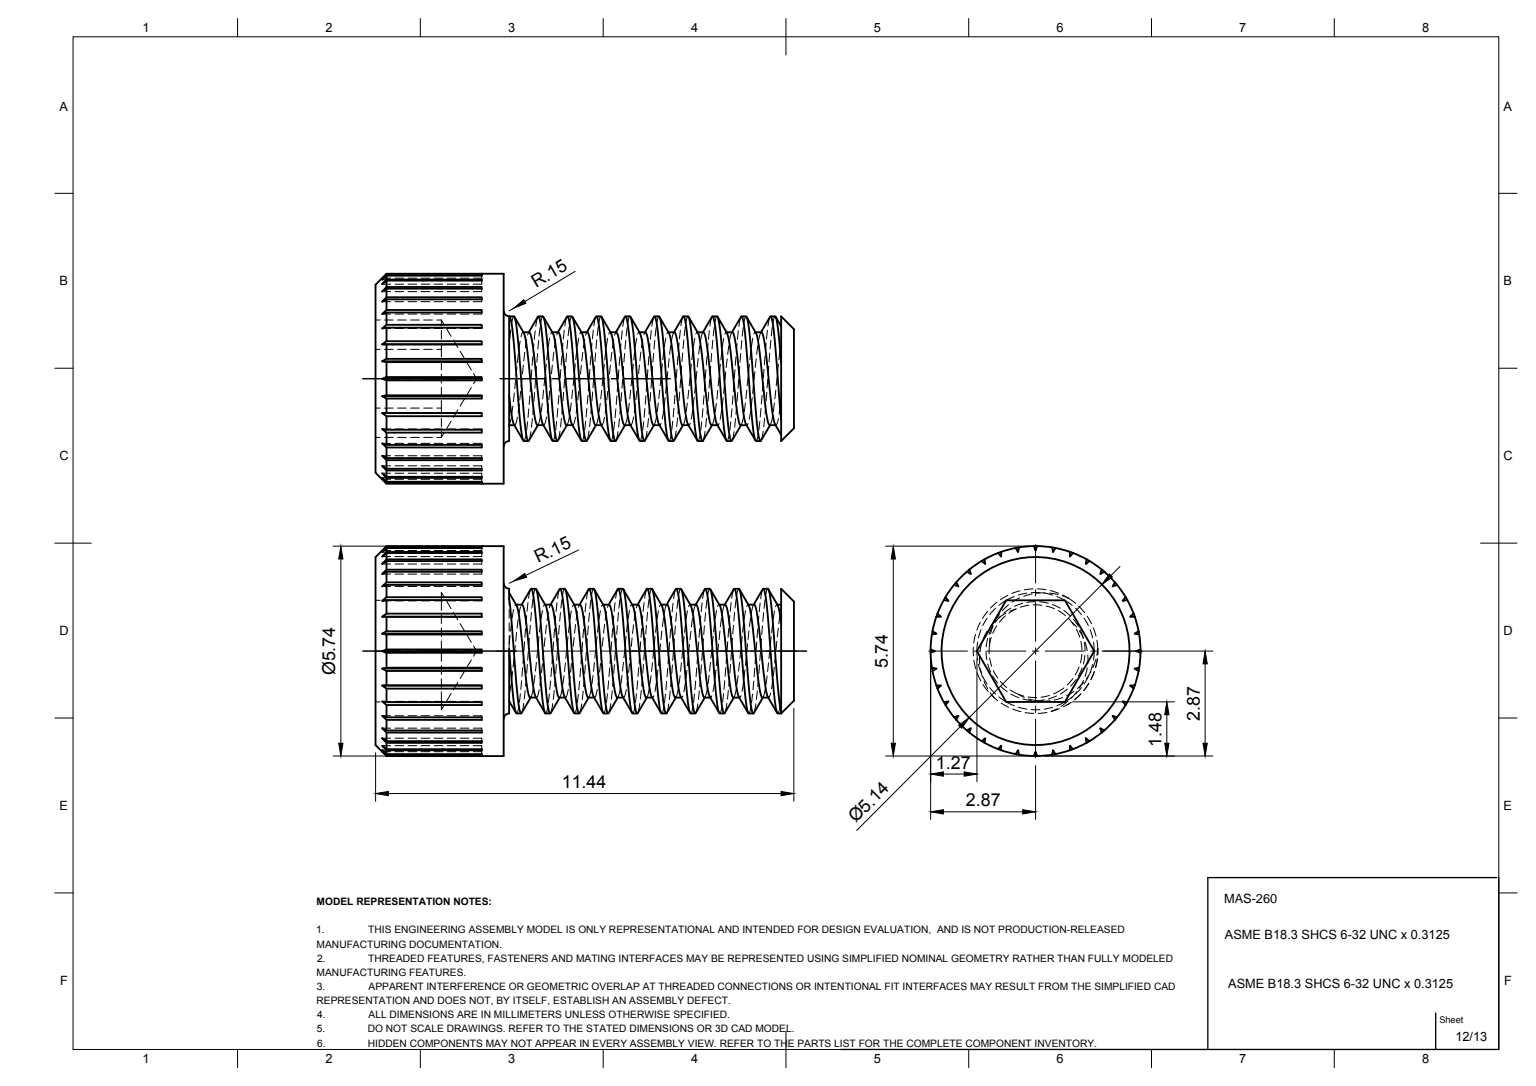
ISO-10303-21;
HEADER;
/* Generated by software containing ST-Developer
 * from STEP Tools, Inc. (www.steptools.com) 
 */

FILE_DESCRIPTION(
/* description */ (''),
/* implementation_level */ '2;1');

FILE_NAME(
/* name */ 'ASME B18.3 SHCS 6-32 UNC x 0.3125.step',
/* time_stamp */ '2026-10-15T13:29:10-07:00',
/* author */ (''),
/* organization */ (''),
/* preprocessor_version */ 'ST-DEVELOPER v20.2',
/* originating_system */ 'Autodesk Translation Framework v15.15.0.0',
/* authorisation */ '');

FILE_SCHEMA (('AUTOMOTIVE_DESIGN { 1 0 10303 214 3 1 1 }'));
ENDSEC;

DATA;
#10=MECHANICAL_DESIGN_GEOMETRIC_PRESENTATION_REPRESENTATION('',(#943),#83219);
#353=(
BOUNDED_CURVE()
B_SPLINE_CURVE(2,(#65992,#65993,#65994),.UNSPECIFIED.,.F.,.F.)
B_SPLINE_CURVE_WITH_KNOTS((3,3),(0.,0.0169283274323722),.UNSPECIFIED.)
CURVE()
GEOMETRIC_REPRESENTATION_ITEM()
RATIONAL_B_SPLINE_CURVE((1.,1.00067437545138,1.00082963690455))
REPRESENTATION_ITEM('')
);
#354=(
BOUNDED_CURVE()
B_SPLINE_CURVE(2,(#65999,#66000,#66001),.UNSPECIFIED.,.F.,.F.)
B_SPLINE_CURVE_WITH_KNOTS((3,3),(0.0270544913418023,0.0439828187741892),
 .UNSPECIFIED.)
CURVE()
GEOMETRIC_REPRESENTATION_ITEM()
RATIONAL_B_SPLINE_CURVE((1.00082963690332,1.00067437545039,1.))
REPRESENTATION_ITEM('')
);
#355=(
BOUNDED_CURVE()
B_SPLINE_CURVE(2,(#66008,#66009,#66010),.UNSPECIFIED.,.F.,.F.)
B_SPLINE_CURVE_WITH_KNOTS((3,3),(0.0270544913418047,0.0439828187741891),
 .UNSPECIFIED.)
CURVE()
GEOMETRIC_REPRESENTATION_ITEM()
RATIONAL_B_SPLINE_CURVE((1.00082963690338,1.00067437545043,1.))
REPRESENTATION_ITEM('')
);
#356=(
BOUNDED_CURVE()
B_SPLINE_CURVE(2,(#66014,#66015,#66016),.UNSPECIFIED.,.F.,.F.)
B_SPLINE_CURVE_WITH_KNOTS((3,3),(0.,0.0169283274323899),.UNSPECIFIED.)
CURVE()
GEOMETRIC_REPRESENTATION_ITEM()
RATIONAL_B_SPLINE_CURVE((1.,1.00067437544971,1.00082963690249))
REPRESENTATION_ITEM('')
);
#357=(
BOUNDED_CURVE()
B_SPLINE_CURVE(2,(#66018,#66019,#66020),.UNSPECIFIED.,.F.,.F.)
B_SPLINE_CURVE_WITH_KNOTS((3,3),(0.0270544913417485,0.0439828187741892),
 .UNSPECIFIED.)
CURVE()
GEOMETRIC_REPRESENTATION_ITEM()
RATIONAL_B_SPLINE_CURVE((1.00082963689667,1.00067437544498,1.))
REPRESENTATION_ITEM('')
);
#358=(
BOUNDED_CURVE()
B_SPLINE_CURVE(2,(#66024,#66025,#66026),.UNSPECIFIED.,.F.,.F.)
B_SPLINE_CURVE_WITH_KNOTS((3,3),(0.,0.0169283274324321),.UNSPECIFIED.)
CURVE()
GEOMETRIC_REPRESENTATION_ITEM()
RATIONAL_B_SPLINE_CURVE((1.,1.00067437544514,1.00082963689687))
REPRESENTATION_ITEM('')
);
#359=(
BOUNDED_CURVE()
B_SPLINE_CURVE(2,(#66028,#66029,#66030),.UNSPECIFIED.,.F.,.F.)
B_SPLINE_CURVE_WITH_KNOTS((3,3),(0.0270544913417875,0.0439828187741892),
 .UNSPECIFIED.)
CURVE()
GEOMETRIC_REPRESENTATION_ITEM()
RATIONAL_B_SPLINE_CURVE((1.00082963689786,1.00067437544595,1.))
REPRESENTATION_ITEM('')
);
#360=(
BOUNDED_CURVE()
B_SPLINE_CURVE(2,(#66034,#66035,#66036),.UNSPECIFIED.,.F.,.F.)
B_SPLINE_CURVE_WITH_KNOTS((3,3),(0.,0.0169283274323828),.UNSPECIFIED.)
CURVE()
GEOMETRIC_REPRESENTATION_ITEM()
RATIONAL_B_SPLINE_CURVE((1.,1.00067437545006,1.00082963690291))
REPRESENTATION_ITEM('')
);
#361=(
BOUNDED_CURVE()
B_SPLINE_CURVE(2,(#66038,#66039,#66040),.UNSPECIFIED.,.F.,.F.)
B_SPLINE_CURVE_WITH_KNOTS((3,3),(0.0270544913418211,0.0439828187741892),
 .UNSPECIFIED.)
CURVE()
GEOMETRIC_REPRESENTATION_ITEM()
RATIONAL_B_SPLINE_CURVE((1.00082963690425,1.00067437545114,1.))
REPRESENTATION_ITEM('')
);
#362=(
BOUNDED_CURVE()
B_SPLINE_CURVE(2,(#66044,#66045,#66046),.UNSPECIFIED.,.F.,.F.)
B_SPLINE_CURVE_WITH_KNOTS((3,3),(0.,0.0169283274323665),.UNSPECIFIED.)
CURVE()
GEOMETRIC_REPRESENTATION_ITEM()
RATIONAL_B_SPLINE_CURVE((1.,1.00067437544743,1.00082963689969))
REPRESENTATION_ITEM('')
);
#363=(
BOUNDED_CURVE()
B_SPLINE_CURVE(2,(#66048,#66049,#66050),.UNSPECIFIED.,.F.,.F.)
B_SPLINE_CURVE_WITH_KNOTS((3,3),(0.0270544913417642,0.043982818774189),
 .UNSPECIFIED.)
CURVE()
GEOMETRIC_REPRESENTATION_ITEM()
RATIONAL_B_SPLINE_CURVE((1.00082963689682,1.0006743754451,1.))
REPRESENTATION_ITEM('')
);
#364=(
BOUNDED_CURVE()
B_SPLINE_CURVE(2,(#66054,#66055,#66056),.UNSPECIFIED.,.F.,.F.)
B_SPLINE_CURVE_WITH_KNOTS((3,3),(0.,0.0169283274324012),.UNSPECIFIED.)
CURVE()
GEOMETRIC_REPRESENTATION_ITEM()
RATIONAL_B_SPLINE_CURVE((1.,1.00067437544784,1.00082963690019))
REPRESENTATION_ITEM('')
);
#365=(
BOUNDED_CURVE()
B_SPLINE_CURVE(2,(#66058,#66059,#66060),.UNSPECIFIED.,.F.,.F.)
B_SPLINE_CURVE_WITH_KNOTS((3,3),(0.0270544913418049,0.0439828187741891),
 .UNSPECIFIED.)
CURVE()
GEOMETRIC_REPRESENTATION_ITEM()
RATIONAL_B_SPLINE_CURVE((1.00082963689975,1.00067437544748,1.))
REPRESENTATION_ITEM('')
);
#366=(
BOUNDED_CURVE()
B_SPLINE_CURVE(2,(#66064,#66065,#66066),.UNSPECIFIED.,.F.,.F.)
B_SPLINE_CURVE_WITH_KNOTS((3,3),(0.,0.0169283274323776),.UNSPECIFIED.)
CURVE()
GEOMETRIC_REPRESENTATION_ITEM()
RATIONAL_B_SPLINE_CURVE((1.,1.00067437545055,1.00082963690352))
REPRESENTATION_ITEM('')
);
#367=(
BOUNDED_CURVE()
B_SPLINE_CURVE(2,(#66068,#66069,#66070),.UNSPECIFIED.,.F.,.F.)
B_SPLINE_CURVE_WITH_KNOTS((3,3),(0.0270544913417675,0.0439828187741888),
 .UNSPECIFIED.)
CURVE()
GEOMETRIC_REPRESENTATION_ITEM()
RATIONAL_B_SPLINE_CURVE((1.00082963689636,1.00067437544473,1.))
REPRESENTATION_ITEM('')
);
#368=(
BOUNDED_CURVE()
B_SPLINE_CURVE(2,(#66074,#66075,#66076),.UNSPECIFIED.,.F.,.F.)
B_SPLINE_CURVE_WITH_KNOTS((3,3),(0.,0.0169283274323805),.UNSPECIFIED.)
CURVE()
GEOMETRIC_REPRESENTATION_ITEM()
RATIONAL_B_SPLINE_CURVE((1.,1.00067437545024,1.00082963690314))
REPRESENTATION_ITEM('')
);
#369=(
BOUNDED_CURVE()
B_SPLINE_CURVE(2,(#66078,#66079,#66080),.UNSPECIFIED.,.F.,.F.)
B_SPLINE_CURVE_WITH_KNOTS((3,3),(0.0270544913417762,0.0439828187741891),
 .UNSPECIFIED.)
CURVE()
GEOMETRIC_REPRESENTATION_ITEM()
RATIONAL_B_SPLINE_CURVE((1.00082963689788,1.00067437544596,1.))
REPRESENTATION_ITEM('')
);
#370=(
BOUNDED_CURVE()
B_SPLINE_CURVE(2,(#66084,#66085,#66086),.UNSPECIFIED.,.F.,.F.)
B_SPLINE_CURVE_WITH_KNOTS((3,3),(0.,0.0169283274323929),.UNSPECIFIED.)
CURVE()
GEOMETRIC_REPRESENTATION_ITEM()
RATIONAL_B_SPLINE_CURVE((1.,1.00067437545034,1.00082963690327))
REPRESENTATION_ITEM('')
);
#371=(
BOUNDED_CURVE()
B_SPLINE_CURVE(2,(#66088,#66089,#66090),.UNSPECIFIED.,.F.,.F.)
B_SPLINE_CURVE_WITH_KNOTS((3,3),(0.0270544913417606,0.0439828187741894),
 .UNSPECIFIED.)
CURVE()
GEOMETRIC_REPRESENTATION_ITEM()
RATIONAL_B_SPLINE_CURVE((1.00082963689914,1.00067437544699,1.))
REPRESENTATION_ITEM('')
);
#372=(
BOUNDED_CURVE()
B_SPLINE_CURVE(2,(#66094,#66095,#66096),.UNSPECIFIED.,.F.,.F.)
B_SPLINE_CURVE_WITH_KNOTS((3,3),(0.,0.0169283274323603),.UNSPECIFIED.)
CURVE()
GEOMETRIC_REPRESENTATION_ITEM()
RATIONAL_B_SPLINE_CURVE((1.,1.00067437544665,1.00082963689872))
REPRESENTATION_ITEM('')
);
#373=(
BOUNDED_CURVE()
B_SPLINE_CURVE(2,(#66098,#66099,#66100),.UNSPECIFIED.,.F.,.F.)
B_SPLINE_CURVE_WITH_KNOTS((3,3),(0.0270544913417842,0.043982818774189),
 .UNSPECIFIED.)
CURVE()
GEOMETRIC_REPRESENTATION_ITEM()
RATIONAL_B_SPLINE_CURVE((1.00082963689636,1.00067437544473,1.))
REPRESENTATION_ITEM('')
);
#374=(
BOUNDED_CURVE()
B_SPLINE_CURVE(2,(#66104,#66105,#66106),.UNSPECIFIED.,.F.,.F.)
B_SPLINE_CURVE_WITH_KNOTS((3,3),(0.,0.0169283274323958),.UNSPECIFIED.)
CURVE()
GEOMETRIC_REPRESENTATION_ITEM()
RATIONAL_B_SPLINE_CURVE((1.,1.00067437544716,1.00082963689935))
REPRESENTATION_ITEM('')
);
#375=(
BOUNDED_CURVE()
B_SPLINE_CURVE(2,(#66108,#66109,#66110),.UNSPECIFIED.,.F.,.F.)
B_SPLINE_CURVE_WITH_KNOTS((3,3),(0.0270544913417961,0.0439828187741891),
 .UNSPECIFIED.)
CURVE()
GEOMETRIC_REPRESENTATION_ITEM()
RATIONAL_B_SPLINE_CURVE((1.00082963689727,1.00067437544546,1.))
REPRESENTATION_ITEM('')
);
#376=(
BOUNDED_CURVE()
B_SPLINE_CURVE(2,(#66114,#66115,#66116),.UNSPECIFIED.,.F.,.F.)
B_SPLINE_CURVE_WITH_KNOTS((3,3),(0.,0.016928327432345),.UNSPECIFIED.)
CURVE()
GEOMETRIC_REPRESENTATION_ITEM()
RATIONAL_B_SPLINE_CURVE((1.,1.00067437545236,1.00082963690575))
REPRESENTATION_ITEM('')
);
#377=(
BOUNDED_CURVE()
B_SPLINE_CURVE(2,(#66118,#66119,#66120),.UNSPECIFIED.,.F.,.F.)
B_SPLINE_CURVE_WITH_KNOTS((3,3),(0.0270544913417455,0.0439828187741891),
 .UNSPECIFIED.)
CURVE()
GEOMETRIC_REPRESENTATION_ITEM()
RATIONAL_B_SPLINE_CURVE((1.00082963689847,1.00067437544644,1.))
REPRESENTATION_ITEM('')
);
#378=(
BOUNDED_CURVE()
B_SPLINE_CURVE(2,(#66124,#66125,#66126),.UNSPECIFIED.,.F.,.F.)
B_SPLINE_CURVE_WITH_KNOTS((3,3),(0.,0.0169283274324359),.UNSPECIFIED.)
CURVE()
GEOMETRIC_REPRESENTATION_ITEM()
RATIONAL_B_SPLINE_CURVE((1.,1.00067437544276,1.00082963689394))
REPRESENTATION_ITEM('')
);
#379=(
BOUNDED_CURVE()
B_SPLINE_CURVE(2,(#66128,#66129,#66130),.UNSPECIFIED.,.F.,.F.)
B_SPLINE_CURVE_WITH_KNOTS((3,3),(0.0270544913417467,0.0439828187741893),
 .UNSPECIFIED.)
CURVE()
GEOMETRIC_REPRESENTATION_ITEM()
RATIONAL_B_SPLINE_CURVE((1.00082963690043,1.00067437544804,1.))
REPRESENTATION_ITEM('')
);
#380=(
BOUNDED_CURVE()
B_SPLINE_CURVE(2,(#66134,#66135,#66136),.UNSPECIFIED.,.F.,.F.)
B_SPLINE_CURVE_WITH_KNOTS((3,3),(0.,0.0169283274323855),.UNSPECIFIED.)
CURVE()
GEOMETRIC_REPRESENTATION_ITEM()
RATIONAL_B_SPLINE_CURVE((1.,1.00067437545031,1.00082963690323))
REPRESENTATION_ITEM('')
);
#381=(
BOUNDED_CURVE()
B_SPLINE_CURVE(2,(#66138,#66139,#66140),.UNSPECIFIED.,.F.,.F.)
B_SPLINE_CURVE_WITH_KNOTS((3,3),(0.0270544913418194,0.043982818774189),
 .UNSPECIFIED.)
CURVE()
GEOMETRIC_REPRESENTATION_ITEM()
RATIONAL_B_SPLINE_CURVE((1.0008296369013,1.00067437544875,1.))
REPRESENTATION_ITEM('')
);
#382=(
BOUNDED_CURVE()
B_SPLINE_CURVE(2,(#66144,#66145,#66146),.UNSPECIFIED.,.F.,.F.)
B_SPLINE_CURVE_WITH_KNOTS((3,3),(0.,0.0169283274324108),.UNSPECIFIED.)
CURVE()
GEOMETRIC_REPRESENTATION_ITEM()
RATIONAL_B_SPLINE_CURVE((1.,1.00067437544706,1.00082963689923))
REPRESENTATION_ITEM('')
);
#383=(
BOUNDED_CURVE()
B_SPLINE_CURVE(2,(#66148,#66149,#66150),.UNSPECIFIED.,.F.,.F.)
B_SPLINE_CURVE_WITH_KNOTS((3,3),(0.0270544913418122,0.043982818774189),
 .UNSPECIFIED.)
CURVE()
GEOMETRIC_REPRESENTATION_ITEM()
RATIONAL_B_SPLINE_CURVE((1.00082963689602,1.00067437544445,1.))
REPRESENTATION_ITEM('')
);
#384=(
BOUNDED_CURVE()
B_SPLINE_CURVE(2,(#66154,#66155,#66156),.UNSPECIFIED.,.F.,.F.)
B_SPLINE_CURVE_WITH_KNOTS((3,3),(0.,0.0169283274323979),.UNSPECIFIED.)
CURVE()
GEOMETRIC_REPRESENTATION_ITEM()
RATIONAL_B_SPLINE_CURVE((1.,1.00067437544686,1.00082963689898))
REPRESENTATION_ITEM('')
);
#385=(
BOUNDED_CURVE()
B_SPLINE_CURVE(2,(#66158,#66159,#66160),.UNSPECIFIED.,.F.,.F.)
B_SPLINE_CURVE_WITH_KNOTS((3,3),(0.0270544913417752,0.0439828187741891),
 .UNSPECIFIED.)
CURVE()
GEOMETRIC_REPRESENTATION_ITEM()
RATIONAL_B_SPLINE_CURVE((1.0008296369011,1.00067437544858,1.))
REPRESENTATION_ITEM('')
);
#386=(
BOUNDED_CURVE()
B_SPLINE_CURVE(2,(#66164,#66165,#66166),.UNSPECIFIED.,.F.,.F.)
B_SPLINE_CURVE_WITH_KNOTS((3,3),(0.,0.0169283274324112),.UNSPECIFIED.)
CURVE()
GEOMETRIC_REPRESENTATION_ITEM()
RATIONAL_B_SPLINE_CURVE((1.,1.00067437544825,1.00082963690069))
REPRESENTATION_ITEM('')
);
#387=(
BOUNDED_CURVE()
B_SPLINE_CURVE(2,(#66168,#66169,#66170),.UNSPECIFIED.,.F.,.F.)
B_SPLINE_CURVE_WITH_KNOTS((3,3),(0.0270544913417757,0.0439828187741891),
 .UNSPECIFIED.)
CURVE()
GEOMETRIC_REPRESENTATION_ITEM()
RATIONAL_B_SPLINE_CURVE((1.00082963690205,1.00067437544935,1.))
REPRESENTATION_ITEM('')
);
#388=(
BOUNDED_CURVE()
B_SPLINE_CURVE(2,(#66174,#66175,#66176),.UNSPECIFIED.,.F.,.F.)
B_SPLINE_CURVE_WITH_KNOTS((3,3),(0.,0.0169283274323844),.UNSPECIFIED.)
CURVE()
GEOMETRIC_REPRESENTATION_ITEM()
RATIONAL_B_SPLINE_CURVE((1.,1.00067437545136,1.00082963690451))
REPRESENTATION_ITEM('')
);
#389=(
BOUNDED_CURVE()
B_SPLINE_CURVE(2,(#66178,#66179,#66180),.UNSPECIFIED.,.F.,.F.)
B_SPLINE_CURVE_WITH_KNOTS((3,3),(0.0270544913417712,0.0439828187741894),
 .UNSPECIFIED.)
CURVE()
GEOMETRIC_REPRESENTATION_ITEM()
RATIONAL_B_SPLINE_CURVE((1.00082963690333,1.00067437545039,1.))
REPRESENTATION_ITEM('')
);
#390=(
BOUNDED_CURVE()
B_SPLINE_CURVE(2,(#66184,#66185,#66186),.UNSPECIFIED.,.F.,.F.)
B_SPLINE_CURVE_WITH_KNOTS((3,3),(0.,0.016928327432381),.UNSPECIFIED.)
CURVE()
GEOMETRIC_REPRESENTATION_ITEM()
RATIONAL_B_SPLINE_CURVE((1.,1.00067437544975,1.00082963690255))
REPRESENTATION_ITEM('')
);
#391=(
BOUNDED_CURVE()
B_SPLINE_CURVE(2,(#66188,#66189,#66190),.UNSPECIFIED.,.F.,.F.)
B_SPLINE_CURVE_WITH_KNOTS((3,3),(0.0270544913418043,0.0439828187741891),
 .UNSPECIFIED.)
CURVE()
GEOMETRIC_REPRESENTATION_ITEM()
RATIONAL_B_SPLINE_CURVE((1.00082963690328,1.00067437545035,1.))
REPRESENTATION_ITEM('')
);
#392=(
BOUNDED_CURVE()
B_SPLINE_CURVE(2,(#66195,#66196,#66197),.UNSPECIFIED.,.F.,.F.)
B_SPLINE_CURVE_WITH_KNOTS((3,3),(0.,0.0169283274323967),.UNSPECIFIED.)
CURVE()
GEOMETRIC_REPRESENTATION_ITEM()
RATIONAL_B_SPLINE_CURVE((1.,1.00067437544999,1.00082963690283))
REPRESENTATION_ITEM('')
);
#393=(
BOUNDED_CURVE()
B_SPLINE_CURVE(2,(#66199,#66200,#66201),.UNSPECIFIED.,.F.,.F.)
B_SPLINE_CURVE_WITH_KNOTS((3,3),(0.0270544913417582,0.0439828187741891),
 .UNSPECIFIED.)
CURVE()
GEOMETRIC_REPRESENTATION_ITEM()
RATIONAL_B_SPLINE_CURVE((1.00082963689937,1.00067437544717,1.))
REPRESENTATION_ITEM('')
);
#394=(
BOUNDED_CURVE()
B_SPLINE_CURVE(2,(#66205,#66206,#66207),.UNSPECIFIED.,.F.,.F.)
B_SPLINE_CURVE_WITH_KNOTS((3,3),(0.,0.0169283274324266),.UNSPECIFIED.)
CURVE()
GEOMETRIC_REPRESENTATION_ITEM()
RATIONAL_B_SPLINE_CURVE((1.,1.00067437544832,1.00082963690078))
REPRESENTATION_ITEM('')
);
#395=(
BOUNDED_CURVE()
B_SPLINE_CURVE(2,(#66209,#66210,#66211),.UNSPECIFIED.,.F.,.F.)
B_SPLINE_CURVE_WITH_KNOTS((3,3),(0.0270544913417777,0.043982818774189),
 .UNSPECIFIED.)
CURVE()
GEOMETRIC_REPRESENTATION_ITEM()
RATIONAL_B_SPLINE_CURVE((1.00082963690226,1.00067437544952,1.))
REPRESENTATION_ITEM('')
);
#396=(
BOUNDED_CURVE()
B_SPLINE_CURVE(2,(#66215,#66216,#66217),.UNSPECIFIED.,.F.,.F.)
B_SPLINE_CURVE_WITH_KNOTS((3,3),(0.,0.0169283274324427),.UNSPECIFIED.)
CURVE()
GEOMETRIC_REPRESENTATION_ITEM()
RATIONAL_B_SPLINE_CURVE((1.,1.00067437544511,1.00082963689683))
REPRESENTATION_ITEM('')
);
#397=(
BOUNDED_CURVE()
B_SPLINE_CURVE(2,(#66219,#66220,#66221),.UNSPECIFIED.,.F.,.F.)
B_SPLINE_CURVE_WITH_KNOTS((3,3),(0.0270544913417577,0.0439828187741891),
 .UNSPECIFIED.)
CURVE()
GEOMETRIC_REPRESENTATION_ITEM()
RATIONAL_B_SPLINE_CURVE((1.00082963689736,1.00067437544554,1.))
REPRESENTATION_ITEM('')
);
#398=(
BOUNDED_CURVE()
B_SPLINE_CURVE(2,(#66225,#66226,#66227),.UNSPECIFIED.,.F.,.F.)
B_SPLINE_CURVE_WITH_KNOTS((3,3),(0.,0.0169283274323561),.UNSPECIFIED.)
CURVE()
GEOMETRIC_REPRESENTATION_ITEM()
RATIONAL_B_SPLINE_CURVE((1.,1.00067437544767,1.00082963689998))
REPRESENTATION_ITEM('')
);
#399=(
BOUNDED_CURVE()
B_SPLINE_CURVE(2,(#66229,#66230,#66231),.UNSPECIFIED.,.F.,.F.)
B_SPLINE_CURVE_WITH_KNOTS((3,3),(0.0270544913417733,0.0439828187741891),
 .UNSPECIFIED.)
CURVE()
GEOMETRIC_REPRESENTATION_ITEM()
RATIONAL_B_SPLINE_CURVE((1.00082963689921,1.00067437544705,1.))
REPRESENTATION_ITEM('')
);
#400=(
BOUNDED_CURVE()
B_SPLINE_CURVE(2,(#66235,#66236,#66237),.UNSPECIFIED.,.F.,.F.)
B_SPLINE_CURVE_WITH_KNOTS((3,3),(0.,0.0169283274323988),.UNSPECIFIED.)
CURVE()
GEOMETRIC_REPRESENTATION_ITEM()
RATIONAL_B_SPLINE_CURVE((1.,1.00067437544932,1.000829636902))
REPRESENTATION_ITEM('')
);
#401=(
BOUNDED_CURVE()
B_SPLINE_CURVE(2,(#66239,#66240,#66241),.UNSPECIFIED.,.F.,.F.)
B_SPLINE_CURVE_WITH_KNOTS((3,3),(0.027054491341826,0.0439828187741891),
 .UNSPECIFIED.)
CURVE()
GEOMETRIC_REPRESENTATION_ITEM()
RATIONAL_B_SPLINE_CURVE((1.00082963690548,1.00067437545214,1.))
REPRESENTATION_ITEM('')
);
#402=(
BOUNDED_CURVE()
B_SPLINE_CURVE(2,(#66245,#66246,#66247),.UNSPECIFIED.,.F.,.F.)
B_SPLINE_CURVE_WITH_KNOTS((3,3),(0.,0.0169283274323669),.UNSPECIFIED.)
CURVE()
GEOMETRIC_REPRESENTATION_ITEM()
RATIONAL_B_SPLINE_CURVE((1.,1.0006743754502,1.00082963690309))
REPRESENTATION_ITEM('')
);
#403=(
BOUNDED_CURVE()
B_SPLINE_CURVE(2,(#66249,#66250,#66251),.UNSPECIFIED.,.F.,.F.)
B_SPLINE_CURVE_WITH_KNOTS((3,3),(0.0270544913418174,0.0439828187741891),
 .UNSPECIFIED.)
CURVE()
GEOMETRIC_REPRESENTATION_ITEM()
RATIONAL_B_SPLINE_CURVE((1.00082963690504,1.00067437545178,1.))
REPRESENTATION_ITEM('')
);
#404=(
BOUNDED_CURVE()
B_SPLINE_CURVE(2,(#66255,#66256,#66257),.UNSPECIFIED.,.F.,.F.)
B_SPLINE_CURVE_WITH_KNOTS((3,3),(0.,0.0169283274323848),.UNSPECIFIED.)
CURVE()
GEOMETRIC_REPRESENTATION_ITEM()
RATIONAL_B_SPLINE_CURVE((1.,1.00067437544897,1.00082963690158))
REPRESENTATION_ITEM('')
);
#405=(
BOUNDED_CURVE()
B_SPLINE_CURVE(2,(#66259,#66260,#66261),.UNSPECIFIED.,.F.,.F.)
B_SPLINE_CURVE_WITH_KNOTS((3,3),(0.0270544913417889,0.0439828187741892),
 .UNSPECIFIED.)
CURVE()
GEOMETRIC_REPRESENTATION_ITEM()
RATIONAL_B_SPLINE_CURVE((1.0008296369053,1.000674375452,1.))
REPRESENTATION_ITEM('')
);
#406=(
BOUNDED_CURVE()
B_SPLINE_CURVE(2,(#66265,#66266,#66267),.UNSPECIFIED.,.F.,.F.)
B_SPLINE_CURVE_WITH_KNOTS((3,3),(0.,0.0169283274323906),.UNSPECIFIED.)
CURVE()
GEOMETRIC_REPRESENTATION_ITEM()
RATIONAL_B_SPLINE_CURVE((1.,1.00067437544955,1.0008296369023))
REPRESENTATION_ITEM('')
);
#407=(
BOUNDED_CURVE()
B_SPLINE_CURVE(2,(#66269,#66270,#66271),.UNSPECIFIED.,.F.,.F.)
B_SPLINE_CURVE_WITH_KNOTS((3,3),(0.02705449134179,0.0439828187741892),
 .UNSPECIFIED.)
CURVE()
GEOMETRIC_REPRESENTATION_ITEM()
RATIONAL_B_SPLINE_CURVE((1.00082963689801,1.00067437544607,1.))
REPRESENTATION_ITEM('')
);
#408=(
BOUNDED_CURVE()
B_SPLINE_CURVE(2,(#66275,#66276,#66277),.UNSPECIFIED.,.F.,.F.)
B_SPLINE_CURVE_WITH_KNOTS((3,3),(0.,0.0169283274324299),.UNSPECIFIED.)
CURVE()
GEOMETRIC_REPRESENTATION_ITEM()
RATIONAL_B_SPLINE_CURVE((1.,1.00067437544605,1.00082963689799))
REPRESENTATION_ITEM('')
);
#409=(
BOUNDED_CURVE()
B_SPLINE_CURVE(2,(#66279,#66280,#66281),.UNSPECIFIED.,.F.,.F.)
B_SPLINE_CURVE_WITH_KNOTS((3,3),(0.0270544913418079,0.0439828187741891),
 .UNSPECIFIED.)
CURVE()
GEOMETRIC_REPRESENTATION_ITEM()
RATIONAL_B_SPLINE_CURVE((1.00082963690421,1.00067437545111,1.))
REPRESENTATION_ITEM('')
);
#410=(
BOUNDED_CURVE()
B_SPLINE_CURVE(2,(#66285,#66286,#66287),.UNSPECIFIED.,.F.,.F.)
B_SPLINE_CURVE_WITH_KNOTS((3,3),(0.,0.0169283274324045),.UNSPECIFIED.)
CURVE()
GEOMETRIC_REPRESENTATION_ITEM()
RATIONAL_B_SPLINE_CURVE((1.,1.00067437544845,1.00082963690094))
REPRESENTATION_ITEM('')
);
#411=(
BOUNDED_CURVE()
B_SPLINE_CURVE(2,(#66289,#66290,#66291),.UNSPECIFIED.,.F.,.F.)
B_SPLINE_CURVE_WITH_KNOTS((3,3),(0.0270544913417581,0.0439828187741892),
 .UNSPECIFIED.)
CURVE()
GEOMETRIC_REPRESENTATION_ITEM()
RATIONAL_B_SPLINE_CURVE((1.00082963689906,1.00067437544692,1.))
REPRESENTATION_ITEM('')
);
#412=(
BOUNDED_CURVE()
B_SPLINE_CURVE(2,(#66295,#66296,#66297),.UNSPECIFIED.,.F.,.F.)
B_SPLINE_CURVE_WITH_KNOTS((3,3),(0.,0.0169283274323899),.UNSPECIFIED.)
CURVE()
GEOMETRIC_REPRESENTATION_ITEM()
RATIONAL_B_SPLINE_CURVE((1.,1.00067437544785,1.0008296369002))
REPRESENTATION_ITEM('')
);
#413=(
BOUNDED_CURVE()
B_SPLINE_CURVE(2,(#66299,#66300,#66301),.UNSPECIFIED.,.F.,.F.)
B_SPLINE_CURVE_WITH_KNOTS((3,3),(0.0270544913417886,0.0439828187741892),
 .UNSPECIFIED.)
CURVE()
GEOMETRIC_REPRESENTATION_ITEM()
RATIONAL_B_SPLINE_CURVE((1.00082963689982,1.00067437544754,1.))
REPRESENTATION_ITEM('')
);
#414=(
BOUNDED_CURVE()
B_SPLINE_CURVE(2,(#66305,#66306,#66307),.UNSPECIFIED.,.F.,.F.)
B_SPLINE_CURVE_WITH_KNOTS((3,3),(0.,0.0169283274324022),.UNSPECIFIED.)
CURVE()
GEOMETRIC_REPRESENTATION_ITEM()
RATIONAL_B_SPLINE_CURVE((1.,1.0006743754471,1.00082963689928))
REPRESENTATION_ITEM('')
);
#415=(
BOUNDED_CURVE()
B_SPLINE_CURVE(2,(#66309,#66310,#66311),.UNSPECIFIED.,.F.,.F.)
B_SPLINE_CURVE_WITH_KNOTS((3,3),(0.02705449134173,0.0439828187741892),
 .UNSPECIFIED.)
CURVE()
GEOMETRIC_REPRESENTATION_ITEM()
RATIONAL_B_SPLINE_CURVE((1.00082963689882,1.00067437544673,1.))
REPRESENTATION_ITEM('')
);
#416=(
BOUNDED_CURVE()
B_SPLINE_CURVE(2,(#66315,#66316,#66317),.UNSPECIFIED.,.F.,.F.)
B_SPLINE_CURVE_WITH_KNOTS((3,3),(0.,0.0169283274323878),.UNSPECIFIED.)
CURVE()
GEOMETRIC_REPRESENTATION_ITEM()
RATIONAL_B_SPLINE_CURVE((1.,1.00067437545001,1.00082963690286))
REPRESENTATION_ITEM('')
);
#417=(
BOUNDED_CURVE()
B_SPLINE_CURVE(2,(#66319,#66320,#66321),.UNSPECIFIED.,.F.,.F.)
B_SPLINE_CURVE_WITH_KNOTS((3,3),(0.0270544913417747,0.043982818774189),
 .UNSPECIFIED.)
CURVE()
GEOMETRIC_REPRESENTATION_ITEM()
RATIONAL_B_SPLINE_CURVE((1.00082963690212,1.00067437544941,1.))
REPRESENTATION_ITEM('')
);
#418=(
BOUNDED_CURVE()
B_SPLINE_CURVE(2,(#66325,#66326,#66327),.UNSPECIFIED.,.F.,.F.)
B_SPLINE_CURVE_WITH_KNOTS((3,3),(0.,0.0169283274324349),.UNSPECIFIED.)
CURVE()
GEOMETRIC_REPRESENTATION_ITEM()
RATIONAL_B_SPLINE_CURVE((1.,1.00067437544449,1.00082963689607))
REPRESENTATION_ITEM('')
);
#419=(
BOUNDED_CURVE()
B_SPLINE_CURVE(2,(#66329,#66330,#66331),.UNSPECIFIED.,.F.,.F.)
B_SPLINE_CURVE_WITH_KNOTS((3,3),(0.0270544913417629,0.0439828187741891),
 .UNSPECIFIED.)
CURVE()
GEOMETRIC_REPRESENTATION_ITEM()
RATIONAL_B_SPLINE_CURVE((1.00082963689925,1.00067437544708,1.))
REPRESENTATION_ITEM('')
);
#420=(
BOUNDED_CURVE()
B_SPLINE_CURVE(2,(#66335,#66336,#66337),.UNSPECIFIED.,.F.,.F.)
B_SPLINE_CURVE_WITH_KNOTS((3,3),(0.,0.01692832743245),.UNSPECIFIED.)
CURVE()
GEOMETRIC_REPRESENTATION_ITEM()
RATIONAL_B_SPLINE_CURVE((1.,1.0006743754471,1.00082963689927))
REPRESENTATION_ITEM('')
);
#421=(
BOUNDED_CURVE()
B_SPLINE_CURVE(2,(#66339,#66340,#66341),.UNSPECIFIED.,.F.,.F.)
B_SPLINE_CURVE_WITH_KNOTS((3,3),(0.027054491341727,0.0439828187741896),
 .UNSPECIFIED.)
CURVE()
GEOMETRIC_REPRESENTATION_ITEM()
RATIONAL_B_SPLINE_CURVE((1.00082963689923,1.00067437544706,1.))
REPRESENTATION_ITEM('')
);
#422=(
BOUNDED_CURVE()
B_SPLINE_CURVE(2,(#66345,#66346,#66347),.UNSPECIFIED.,.F.,.F.)
B_SPLINE_CURVE_WITH_KNOTS((3,3),(0.,0.0169283274324584),.UNSPECIFIED.)
CURVE()
GEOMETRIC_REPRESENTATION_ITEM()
RATIONAL_B_SPLINE_CURVE((1.,1.00067437544543,1.00082963689722))
REPRESENTATION_ITEM('')
);
#423=(
BOUNDED_CURVE()
B_SPLINE_CURVE(2,(#66349,#66350,#66351),.UNSPECIFIED.,.F.,.F.)
B_SPLINE_CURVE_WITH_KNOTS((3,3),(0.0270544913416968,0.0439828187741891),
 .UNSPECIFIED.)
CURVE()
GEOMETRIC_REPRESENTATION_ITEM()
RATIONAL_B_SPLINE_CURVE((1.00082963689609,1.00067437544451,1.))
REPRESENTATION_ITEM('')
);
#424=(
BOUNDED_CURVE()
B_SPLINE_CURVE(2,(#66354,#66355,#66356),.UNSPECIFIED.,.F.,.F.)
B_SPLINE_CURVE_WITH_KNOTS((3,3),(0.,0.0169283274323624),.UNSPECIFIED.)
CURVE()
GEOMETRIC_REPRESENTATION_ITEM()
RATIONAL_B_SPLINE_CURVE((1.,1.00067437544963,1.0008296369024))
REPRESENTATION_ITEM('')
);
#506=TOROIDAL_SURFACE('',#28715,1.85434,0.15);
#693=B_SPLINE_CURVE_WITH_KNOTS('',3,(#59389,#59390,#59391,#59392,#59393,
#59394,#59395,#59396,#59397,#59398,#59399,#59400,#59401,#59402,#59403,#59404,
#59405,#59406,#59407,#59408,#59409,#59410,#59411,#59412,#59413,#59414,#59415,
#59416,#59417,#59418,#59419,#59420,#59421,#59422,#59423,#59424,#59425,#59426,
#59427,#59428,#59429,#59430,#59431,#59432,#59433,#59434,#59435,#59436,#59437,
#59438,#59439,#59440,#59441,#59442,#59443,#59444,#59445,#59446,#59447,#59448,
#59449,#59450,#59451,#59452,#59453,#59454,#59455,#59456,#59457,#59458,#59459,
#59460,#59461,#59462,#59463,#59464,#59465,#59466,#59467,#59468,#59469,#59470,
#59471,#59472,#59473,#59474,#59475,#59476,#59477,#59478,#59479,#59480,#59481,
#59482,#59483,#59484,#59485,#59486,#59487,#59488,#59489,#59490,#59491,#59492,
#59493,#59494,#59495,#59496,#59497,#59498,#59499,#59500,#59501,#59502,#59503,
#59504,#59505,#59506,#59507,#59508,#59509,#59510,#59511,#59512,#59513,#59514,
#59515),.UNSPECIFIED.,.F.,.F.,(4,3,3,3,3,3,3,3,3,3,3,3,3,3,3,3,3,3,3,3,
3,3,3,3,3,3,3,3,3,3,3,3,3,3,3,3,3,3,3,3,3,3,4),(10.3244224454295,10.3347762602768,
10.4523755104341,10.5697567932924,10.687017805337,10.8042083393309,10.921378073836,
11.0386591521697,11.1560016504262,11.273559681505,11.3324641798094,11.4501570625527,
11.5676398197509,11.6850070752187,11.8023084152573,11.9195933182444,12.0369952827684,
12.1544620980084,12.2721483369573,12.3301520993421,12.4475267014295,12.5646823078878,
12.6817172043898,12.7986816223694,12.9156256782421,13.032683561123,13.1498039510826,
13.2671442032613,13.3278400188747,13.4453614082309,13.5626664785529,13.6798523713343,
13.7969690317053,13.9140662920102,14.0312776252005,14.1485518345722,14.2660446675354,
14.3255279384074,14.4430457990983,14.5603521333803,14.6775359904871,14.7946582937227,
14.8497137389722),.UNSPECIFIED.);
#694=B_SPLINE_CURVE_WITH_KNOTS('',3,(#59518,#59519,#59520,#59521,#59522,
#59523,#59524,#59525,#59526,#59527,#59528,#59529,#59530,#59531,#59532,#59533,
#59534,#59535,#59536,#59537,#59538,#59539,#59540,#59541,#59542,#59543,#59544,
#59545,#59546,#59547,#59548,#59549,#59550,#59551,#59552,#59553,#59554,#59555,
#59556,#59557,#59558,#59559,#59560,#59561,#59562,#59563,#59564,#59565,#59566,
#59567,#59568,#59569,#59570,#59571,#59572,#59573,#59574,#59575,#59576,#59577,
#59578,#59579,#59580,#59581,#59582,#59583,#59584,#59585,#59586,#59587,#59588,
#59589,#59590,#59591,#59592,#59593,#59594,#59595,#59596,#59597,#59598,#59599,
#59600,#59601,#59602,#59603,#59604,#59605),.UNSPECIFIED.,.F.,.F.,(4,3,3,
3,3,3,3,3,3,3,3,3,3,3,3,3,3,3,3,3,3,3,3,3,3,3,3,3,3,4),(11.6667261296989,
11.7914371196405,11.9115078206976,12.0315495137313,12.1516029751615,12.27170898462,
12.3920043210467,12.5124089010735,12.6330580926368,12.6644140492316,12.7808766559592,
12.8970982188996,13.0131860262978,13.1291919200962,13.2451676019825,13.3612494874271,
13.4773878723687,13.5937483072809,13.6621019687642,13.7797013220772,13.8970827102571,
14.014343828866,14.1315344704521,14.2487043133647,14.3659855004597,14.4833281078319,
14.6008862472843,14.6597898882969,14.7774514636229,14.8502992189952),
 .UNSPECIFIED.);
#695=B_SPLINE_CURVE_WITH_KNOTS('',3,(#59611,#59612,#59613,#59614,#59615,
#59616,#59617,#59618,#59619,#59620,#59621,#59622,#59623,#59624,#59625,#59626,
#59627,#59628,#59629,#59630,#59631,#59632,#59633,#59634,#59635,#59636,#59637,
#59638,#59639,#59640,#59641,#59642,#59643,#59644,#59645,#59646,#59647,#59648,
#59649,#59650,#59651,#59652,#59653,#59654,#59655,#59656,#59657,#59658,#59659,
#59660,#59661,#59662,#59663,#59664,#59665,#59666,#59667,#59668,#59669,#59670,
#59671,#59672,#59673,#59674,#59675,#59676,#59677,#59678,#59679,#59680,#59681,
#59682,#59683,#59684,#59685,#59686,#59687,#59688,#59689,#59690,#59691,#59692,
#59693,#59694,#59695,#59696,#59697,#59698,#59699,#59700,#59701,#59702,#59703,
#59704,#59705,#59706,#59707,#59708,#59709,#59710,#59711,#59712,#59713,#59714,
#59715,#59716,#59717,#59718,#59719,#59720,#59721,#59722,#59723,#59724,#59725,
#59726,#59727,#59728,#59729,#59730,#59731,#59732,#59733,#59734,#59735,#59736,
#59737,#59738,#59739,#59740,#59741,#59742,#59743,#59744,#59745,#59746,#59747,
#59748,#59749,#59750,#59751,#59752,#59753,#59754,#59755,#59756,#59757,#59758),
 .UNSPECIFIED.,.F.,.F.,(4,3,3,3,3,3,3,3,3,3,3,3,3,3,3,3,3,3,3,3,3,3,3,3,
3,3,3,3,3,3,3,3,3,3,3,3,3,3,3,3,3,3,3,3,3,3,3,3,3,4),(15.7079632679489,
15.826189752956,15.9498682590852,16.0683010825115,16.1868385915478,16.3056105526879,
16.3209037774727,16.4384084206739,16.5556968022436,16.6728660565512,16.7899661610164,
16.9070469803279,17.0242421798739,17.1415004071429,17.2589776838822,17.3185916970053,
17.4360947212145,17.5533815374925,17.6705492611684,17.787647872645,17.9047272396398,
18.0219210605523,18.1391779491447,18.2566539655226,18.3162796165379,18.4337783817821,
18.5510608066487,18.6682240606424,18.785318132747,18.9023928991528,19.0195820630453,
19.1368342556321,19.2543055705415,19.3139675360706,19.4314690346998,19.5487542516085,
19.6659203315695,19.7830172581319,19.9000949020984,20.0172869556911,20.134542049137,
20.2520162480687,20.3116554556032,20.4291191392111,20.5464069655919,20.663569125986,
20.78077716451,20.8978784283634,21.0151398542227,21.132401280082),
 .UNSPECIFIED.);
#696=B_SPLINE_CURVE_WITH_KNOTS('',3,(#59759,#59760,#59761,#59762,#59763,
#59764,#59765,#59766,#59767,#59768,#59769,#59770,#59771,#59772,#59773,#59774,
#59775,#59776,#59777,#59778,#59779,#59780),.UNSPECIFIED.,.F.,.F.,(4,3,3,
3,3,3,3,4),(14.8497137389722,14.9680892687142,15.0853285498675,15.2042722039037,
15.32321585794,15.4550717956996,15.5859966424603,15.7079632672096),
 .UNSPECIFIED.);
#697=B_SPLINE_CURVE_WITH_KNOTS('',3,(#59782,#59783,#59784,#59785,#59786,
#59787,#59788,#59789,#59790,#59791,#59792,#59793,#59794,#59795,#59796,#59797,
#59798,#59799,#59800,#59801,#59802,#59803,#59804,#59805,#59806),
 .UNSPECIFIED.,.F.,.F.,(4,3,3,3,3,3,3,3,4),(14.8502992189952,14.967704568568,
15.0850251599573,15.2023105050779,15.3196994923041,15.4371364444717,15.5548075604255,
15.6574778078295,15.707963267949),.UNSPECIFIED.);
#698=B_SPLINE_CURVE_WITH_KNOTS('',3,(#59807,#59808,#59809,#59810,#59811,
#59812,#59813,#59814,#59815,#59816,#59817,#59818,#59819,#59820,#59821,#59822,
#59823,#59824,#59825,#59826,#59827,#59828,#59829,#59830,#59831,#59832,#59833,
#59834,#59835,#59836,#59837,#59838,#59839,#59840,#59841,#59842,#59843,#59844,
#59845,#59846,#59847,#59848,#59849,#59850,#59851,#59852,#59853,#59854,#59855,
#59856,#59857,#59858,#59859,#59860,#59861,#59862,#59863,#59864,#59865,#59866,
#59867,#59868,#59869,#59870,#59871,#59872,#59873,#59874,#59875,#59876,#59877,
#59878,#59879,#59880,#59881,#59882,#59883,#59884,#59885,#59886,#59887,#59888,
#59889,#59890,#59891,#59892,#59893,#59894,#59895,#59896,#59897,#59898,#59899,
#59900,#59901,#59902,#59903,#59904,#59905,#59906,#59907,#59908,#59909,#59910,
#59911,#59912,#59913,#59914,#59915,#59916,#59917,#59918,#59919,#59920,#59921,
#59922,#59923,#59924,#59925,#59926,#59927,#59928,#59929,#59930,#59931,#59932,
#59933,#59934,#59935,#59936,#59937,#59938),.UNSPECIFIED.,.F.,.F.,(4,2,2,
2,2,2,2,2,2,2,2,2,2,2,2,2,2,2,2,2,2,2,2,2,2,2,2,2,2,2,2,2,2,2,2,2,2,2,2,
2,2,2,2,2,2,2,2,2,2,2,2,2,2,2,2,2,2,2,2,2,2,2,2,2,2,4),(-1.60493377957124,
-1.59987050848402,-1.57873903548264,-1.5648359244767,-1.55461258883571,
-1.54874460226824,-1.54328239853955,-1.53555119059207,-1.51169698163715,
-1.49725423878715,-1.48864381489348,-1.4848726374927,-1.48176283324838,
-1.47715240856349,-1.45189900306032,-1.43756837907325,-1.42713333431231,
-1.42119940320615,-1.4156983768377,-1.40793791028021,-1.38588980103349,
-1.37045291892543,-1.36151402510944,-1.35767587646358,-1.35455596745909,
-1.34996766518868,-1.32452284345291,-1.31030162976917,-1.29992164311062,
-1.29400218866262,-1.288506604496,-1.28074346759365,-1.25749367219419,-1.24276389961884,
-1.23405212812915,-1.23025149730065,-1.2271349817491,-1.22252046117701,
-1.19733279743846,-1.18298886558583,-1.17255509215521,-1.16663137082758,
-1.161147151725,-1.15342827229919,-1.12924645011164,-1.11509233685587,-1.10657725173874,
-1.10280684884489,-1.09968391211381,-1.09501762992913,-1.07028877408506,
-1.05573899165196,-1.04521151415666,-1.03926822881994,-1.03378261817331,
-1.02608890605539,-1.00149665014118,-0.987597931946931,-0.97917098091361,
-0.975410759328862,-0.972282483199418,-0.96758493485304,-0.943147114271868,
-0.928468919189071,-0.917885814304118,-0.912322913525635),.UNSPECIFIED.);
#699=B_SPLINE_CURVE_WITH_KNOTS('',3,(#59944,#59945,#59946,#59947,#59948,
#59949,#59950,#59951,#59952,#59953),.UNSPECIFIED.,.F.,.F.,(4,1,1,1,1,1,
1,4),(21.9911547274662,22.3070312946685,23.3047192142012,24.3024071337338,
25.3000950532664,26.2977829727991,27.2954708923317,27.4168377020878),
 .UNSPECIFIED.);
#700=B_SPLINE_CURVE_WITH_KNOTS('',3,(#59954,#59955,#59956,#59957,#59958,
#59959,#59960,#59961,#59962,#59963,#59964,#59965,#59966,#59967,#59968,#59969,
#59970,#59971,#59972,#59973,#59974,#59975,#59976,#59977,#59978),
 .UNSPECIFIED.,.F.,.F.,(4,3,3,3,3,3,3,3,4),(21.132401280082,21.24987516791,
21.3093433751359,21.4264262274341,21.543322914988,21.6600916557656,21.7767813160478,
21.8934986553372,21.9911485751285),.UNSPECIFIED.);
#701=B_SPLINE_CURVE_WITH_KNOTS('',3,(#59979,#59980,#59981,#59982,#59983,
#59984,#59985,#59986,#59987,#59988,#59989,#59990,#59991,#59992,#59993,#59994,
#59995,#59996,#59997,#59998,#59999,#60000,#60001,#60002,#60003,#60004,#60005,
#60006,#60007,#60008,#60009,#60010,#60011,#60012,#60013,#60014,#60015,#60016,
#60017,#60018,#60019,#60020,#60021,#60022,#60023,#60024,#60025,#60026,#60027,
#60028,#60029,#60030,#60031,#60032,#60033,#60034,#60035,#60036,#60037,#60038,
#60039,#60040,#60041,#60042,#60043,#60044,#60045,#60046,#60047,#60048,#60049,
#60050,#60051,#60052,#60053,#60054,#60055,#60056,#60057,#60058,#60059,#60060,
#60061,#60062,#60063,#60064,#60065,#60066,#60067,#60068,#60069,#60070,#60071,
#60072,#60073,#60074,#60075,#60076,#60077,#60078,#60079,#60080,#60081,#60082,
#60083,#60084,#60085,#60086,#60087,#60088,#60089,#60090,#60091,#60092,#60093,
#60094,#60095,#60096,#60097,#60098,#60099,#60100,#60101,#60102,#60103,#60104,
#60105,#60106,#60107,#60108,#60109,#60110,#60111,#60112,#60113,#60114,#60115,
#60116,#60117,#60118,#60119,#60120,#60121,#60122,#60123,#60124,#60125,#60126,
#60127,#60128,#60129,#60130,#60131,#60132,#60133,#60134),.UNSPECIFIED.,
 .F.,.F.,(4,2,2,2,2,2,2,2,2,2,2,2,2,2,2,2,2,2,2,2,2,2,2,2,2,2,2,2,2,2,2,
2,2,2,2,2,2,2,2,2,2,2,2,2,2,2,2,2,2,2,2,2,2,2,2,2,2,2,2,2,2,2,2,2,2,2,2,
2,2,2,2,2,2,2,2,2,2,4),(-0.912322913525635,-0.911934213429162,-0.906453142965189,
-0.898787260140372,-0.879414340197368,-0.858265688943076,-0.851153416297868,
-0.847603568824797,-0.844442247367097,-0.83930043026472,-0.820203687819216,
-0.802826045528258,-0.791154694853652,-0.785032783277211,-0.779599803321779,
-0.772326703986733,-0.749367388765553,-0.727078572155622,-0.722152171413902,
-0.719024174275046,-0.71539076438579,-0.707779059166838,-0.696050432795616,
-0.666943894355935,-0.659817099380472,-0.65438565197958,-0.648253517458123,
-0.636518001640174,-0.61896776714075,-0.600080746878765,-0.594948576159234,
-0.591788718033106,-0.588234959186982,-0.581099904991374,-0.559933117993286,
-0.540654512818056,-0.532995259329514,-0.527515290701031,-0.521561513614715,
-0.510965354953334,-0.496256999783314,-0.471830933835663,-0.467128044760812,
-0.463999773517692,-0.460244777094813,-0.451847253290902,-0.438031839855466,
-0.413316089936075,-0.405633971576458,-0.400151068729167,-0.394206016891429,
-0.383662826190182,-0.369075146164618,-0.344381314246961,-0.339707249571018,
-0.336582537398261,-0.332812105706658,-0.324309442893067,-0.310192603935533,
-0.286007069481154,-0.278290719175982,-0.272803145618507,-0.266870405857176,
-0.256402921158967,-0.241986607365549,-0.216907104545424,-0.212274690725974,
-0.209154858986032,-0.205361231085055,-0.19669793812975,-0.182109284583203,
-0.158703230132587,-0.150951523297094,-0.145459124057986,-0.13953890466759,
-0.129147838899375,-0.114902840850451,-0.110035658503537),.UNSPECIFIED.);
#702=B_SPLINE_CURVE_WITH_KNOTS('',3,(#60140,#60141,#60142,#60143,#60144,
#60145,#60146,#60147,#60148,#60149,#60150,#60151,#60152,#60153,#60154,#60155,
#60156,#60157,#60158,#60159,#60160,#60161,#60162,#60163,#60164,#60165,#60166,
#60167,#60168,#60169,#60170,#60171,#60172,#60173,#60174,#60175,#60176,#60177,
#60178,#60179,#60180,#60181,#60182,#60183,#60184,#60185,#60186,#60187,#60188,
#60189,#60190,#60191,#60192,#60193,#60194,#60195,#60196,#60197,#60198,#60199,
#60200,#60201,#60202,#60203,#60204,#60205,#60206,#60207,#60208,#60209,#60210,
#60211,#60212,#60213,#60214,#60215,#60216,#60217,#60218,#60219,#60220,#60221,
#60222,#60223,#60224,#60225,#60226,#60227,#60228,#60229,#60230,#60231,#60232,
#60233,#60234,#60235,#60236,#60237,#60238,#60239,#60240,#60241,#60242,#60243,
#60244,#60245,#60246,#60247,#60248,#60249,#60250,#60251,#60252,#60253,#60254,
#60255,#60256,#60257,#60258,#60259,#60260,#60261,#60262,#60263,#60264,#60265,
#60266,#60267,#60268,#60269,#60270,#60271,#60272,#60273,#60274,#60275,#60276,
#60277,#60278,#60279,#60280,#60281,#60282,#60283,#60284,#60285,#60286,#60287,
#60288,#60289,#60290),.UNSPECIFIED.,.F.,.F.,(4,3,3,3,3,3,3,3,3,3,3,3,3,
3,3,3,3,3,3,3,3,3,3,3,3,3,3,3,3,3,3,3,3,3,3,3,3,3,3,3,3,3,3,3,3,3,3,3,3,
3,4),(28.2743338823081,28.2931588118644,28.4106596979302,28.5279442948967,
28.6451097508825,28.7622060506395,28.8792830661675,28.996474493875,29.1137289619717,
29.2312025437845,29.290846731397,29.4083476154735,29.5256322104213,29.642797664372,
29.7598939620814,29.8769709755534,29.9941624012081,30.1114168672509,30.2288904470325,
30.2885346509297,30.4060355346255,30.5233201291716,30.6404855827079,30.7575818799911,
30.8746588930257,30.9918503182297,31.1091047838135,31.2265783631284,31.2862225704623,
31.4037234548693,31.5210080501455,31.638173504423,31.755269802457,31.8723468162507,
31.9895382422202,32.1067927085743,32.2242662886579,32.283910489995,32.4014113741103,
32.5186959690898,32.6358614230678,32.7529577208,32.8700347342901,32.987226159956,
33.104480626006,33.2219542057883,33.2815984095276,33.399060761611,33.5163536756721,
33.633518003233,33.6995974475487),.UNSPECIFIED.);
#703=B_SPLINE_CURVE_WITH_KNOTS('',3,(#60291,#60292,#60293,#60294),
 .UNSPECIFIED.,.F.,.F.,(4,4),(27.4168377020878,28.27433136801),
 .UNSPECIFIED.);
#704=B_SPLINE_CURVE_WITH_KNOTS('',3,(#60296,#60297,#60298,#60299,#60300,
#60301,#60302,#60303,#60304,#60305,#60306,#60307,#60308,#60309,#60310,#60311,
#60312,#60313,#60314,#60315,#60316,#60317,#60318,#60319,#60320,#60321),
 .UNSPECIFIED.,.F.,.F.,(4,2,2,2,2,2,2,2,2,2,2,2,4),(-0.110035658503537,
-0.0894303473050645,-0.0848411241296203,-0.0817261029194477,-0.0779073952651996,
-0.0690669192919908,-0.0472928151504454,-0.0292032109585574,-0.0223105991302409,
-0.0169104081760242,-0.0118102046580991,-0.00662420233944239,-0.000375289463787094),
 .UNSPECIFIED.);
#705=B_SPLINE_CURVE_WITH_KNOTS('',3,(#60322,#60323,#60324,#60325,#60326,
#60327,#60328,#60329,#60330,#60331),.UNSPECIFIED.,.F.,.F.,(4,1,1,1,1,1,
1,4),(28.2743410485279,28.6274207617539,29.6251086812865,30.6227966008192,
31.6204845203518,32.6181724398845,33.6158603594171,33.6998501991794),
 .UNSPECIFIED.);
#706=B_SPLINE_CURVE_WITH_KNOTS('',3,(#60337,#60338,#60339,#60340,#60341,
#60342,#60343,#60344,#60345),.UNSPECIFIED.,.F.,.F.,(4,1,1,1,1,1,4),(34.5575191894877,
35.2769742485929,36.2746621681255,37.2723500876582,38.2700380071908,39.2677259267235,
39.9816638270269),.UNSPECIFIED.);
#707=B_SPLINE_CURVE_WITH_KNOTS('',3,(#60346,#60347,#60348,#60349,#60350,
#60351,#60352,#60353,#60354,#60355,#60356,#60357,#60358,#60359,#60360,#60361,
#60362,#60363,#60364,#60365,#60366,#60367),.UNSPECIFIED.,.F.,.F.,(4,3,3,
3,3,3,3,4),(33.6995974475487,33.8166767415956,33.9338547022906,34.0510762006772,
34.1685337552212,34.2792863290602,34.4251381581413,34.5575191894877),
 .UNSPECIFIED.);
#708=B_SPLINE_CURVE_WITH_KNOTS('',3,(#60369,#60370,#60371,#60372),
 .UNSPECIFIED.,.F.,.F.,(4,4),(33.6998501991794,34.5575124975197),
 .UNSPECIFIED.);
#709=B_SPLINE_CURVE_WITH_KNOTS('',3,(#60373,#60374,#60375,#60376,#60377,
#60378,#60379,#60380,#60381,#60382,#60383,#60384,#60385,#60386,#60387,#60388,
#60389,#60390,#60391,#60392,#60393,#60394,#60395,#60396,#60397,#60398,#60399,
#60400,#60401,#60402,#60403,#60404,#60405,#60406,#60407,#60408,#60409,#60410,
#60411,#60412,#60413,#60414,#60415,#60416,#60417,#60418,#60419,#60420,#60421,
#60422,#60423,#60424,#60425,#60426,#60427,#60428,#60429,#60430,#60431,#60432,
#60433,#60434,#60435,#60436,#60437,#60438,#60439,#60440,#60441,#60442,#60443,
#60444,#60445,#60446,#60447,#60448,#60449,#60450,#60451,#60452,#60453,#60454,
#60455,#60456,#60457,#60458,#60459,#60460,#60461,#60462,#60463,#60464,#60465,
#60466,#60467,#60468,#60469,#60470,#60471,#60472,#60473,#60474,#60475,#60476,
#60477,#60478,#60479,#60480,#60481,#60482,#60483,#60484,#60485,#60486,#60487,
#60488,#60489,#60490,#60491,#60492,#60493,#60494,#60495,#60496,#60497,#60498,
#60499,#60500,#60501,#60502,#60503,#60504,#60505,#60506,#60507,#60508,#60509,
#60510),.UNSPECIFIED.,.F.,.F.,(4,2,2,2,2,2,2,2,2,2,2,2,2,2,2,2,2,2,2,2,
2,2,2,2,2,2,2,2,2,2,2,2,2,2,2,2,2,2,2,2,2,2,2,2,2,2,2,2,2,2,2,2,2,2,2,2,
2,2,2,2,2,2,2,2,2,2,2,2,4),(-1.60459719055946,-1.60178300272715,-1.59909075093962,
-1.59628461001764,-1.59236418356326,-1.5833727425585,-1.5722137340225,-1.55111601522325,
-1.54075620618843,-1.53484335691492,-1.52935184120328,-1.52159118596671,
-1.49857215188127,-1.4837211004988,-1.47497180794081,-1.47116706137049,
-1.46805121871521,-1.46344367854927,-1.43820349813744,-1.42389164310272,
-1.41347210593244,-1.40754925737045,-1.40206130202897,-1.39432808903217,
-1.37046814396921,-1.35614401031577,-1.34757135725019,-1.34379175533296,
-1.34067063425579,-1.3360182526735,-1.31118737489542,-1.29669394191008,
-1.28619358587361,-1.28025730799103,-1.27477405070355,-1.26707709862348,
-1.24256716076334,-1.22862131963994,-1.22017908177656,-1.21641834587374,
-1.21329281820254,-1.20860514426719,-1.18409967261904,-1.16945948900438,
-1.15889436100026,-1.15294727887949,-1.14746751063494,-1.13979855686478,
-1.1105184887593,-1.0995710482709,-1.0922829839777,-1.08870398743655,-1.08555668711595,
-1.08049892228391,-1.06041648563823,-1.04356751459763,-1.0320968106417,
-1.02600645043121,-1.02056807886404,-1.01323587052882,-0.985107442701769,
-0.972946762200217,-0.965164547068087,-0.961504382705103,-0.958386055406396,
-0.953524227222894,-0.930646036895216,-0.915256780825494,-0.912207559110817),
 .UNSPECIFIED.);
#710=B_SPLINE_CURVE_WITH_KNOTS('',3,(#60516,#60517,#60518,#60519,#60520,
#60521,#60522,#60523,#60524,#60525,#60526,#60527,#60528,#60529,#60530,#60531,
#60532,#60533,#60534,#60535,#60536,#60537,#60538,#60539,#60540,#60541,#60542,
#60543,#60544,#60545,#60546,#60547,#60548,#60549,#60550,#60551,#60552,#60553,
#60554,#60555,#60556,#60557,#60558,#60559,#60560,#60561,#60562,#60563,#60564,
#60565,#60566,#60567,#60568,#60569,#60570,#60571,#60572,#60573,#60574,#60575,
#60576,#60577,#60578,#60579,#60580,#60581,#60582,#60583,#60584,#60585,#60586,
#60587,#60588,#60589,#60590,#60591,#60592,#60593,#60594,#60595,#60596,#60597,
#60598,#60599,#60600,#60601,#60602,#60603,#60604,#60605,#60606,#60607,#60608,
#60609,#60610,#60611,#60612,#60613,#60614,#60615,#60616,#60617,#60618,#60619,
#60620,#60621,#60622,#60623,#60624,#60625,#60626,#60627,#60628,#60629,#60630,
#60631,#60632,#60633,#60634,#60635,#60636,#60637,#60638,#60639,#60640,#60641,
#60642,#60643,#60644,#60645,#60646,#60647,#60648,#60649),.UNSPECIFIED.,
 .F.,.F.,(4,2,2,2,2,2,2,2,2,2,2,2,2,2,2,2,2,2,2,2,2,2,2,2,2,2,2,2,2,2,2,
2,2,2,2,2,2,2,2,2,2,2,2,2,2,2,2,2,2,2,2,2,2,2,2,2,2,2,2,2,2,2,2,2,2,2,4),
(-0.692954581112378,-0.690107125872129,-0.686278982582345,-0.677373495051638,
-0.662046489541168,-0.639752470891751,-0.631985260140913,-0.626489929875214,
-0.620573383190546,-0.610208902127747,-0.596023681417976,-0.570414862652245,
-0.565840706522337,-0.562726803929921,-0.558897581131768,-0.549984389854336,
-0.534633358682857,-0.512373323730011,-0.504606311021614,-0.499110991348438,
-0.493194343690737,-0.482829345411824,-0.468643009062657,-0.443036561584647,
-0.438462109864493,-0.435348166185292,-0.431519097085452,-0.422607085052476,
-0.407259789393917,-0.384994282016187,-0.377227200757971,-0.371731854577023,
-0.36581519746099,-0.355450240397643,-0.341264029676267,-0.315657064695619,
-0.311082642573696,-0.307968691858849,-0.304139579431889,-0.29522732708495,
-0.279879328197489,-0.257614650002929,-0.249847545373831,-0.244352178954194,
-0.238435496831611,-0.228070486209916,-0.213884190487116,-0.188277197981138,
-0.183702750285698,-0.180588786759347,-0.176759664444986,-0.167847412637021,
-0.152499463549225,-0.130234545281643,-0.122467409702783,-0.116972022015258,
-0.111055317542599,-0.100690269437631,-0.0865039244304431,-0.0608968211554993,
-0.056322357259471,-0.0532083819119233,-0.0493792440502393,-0.0404669520209199,
-0.0251189252975217,-0.00796884978255691,-0.000386348129261924),
 .UNSPECIFIED.);
#711=B_SPLINE_CURVE_WITH_KNOTS('',3,(#60650,#60651,#60652,#60653,#60654),
 .UNSPECIFIED.,.F.,.F.,(4,1,4),(39.9816638270269,40.2654138462561,40.8407044966673),
 .UNSPECIFIED.);
#712=B_SPLINE_CURVE_WITH_KNOTS('',3,(#60655,#60656,#60657,#60658,#60659,
#60660,#60661,#60662,#60663,#60664,#60665,#60666,#60667,#60668,#60669,#60670,
#60671,#60672,#60673,#60674,#60675,#60676,#60677,#60678,#60679,#60680,#60681,
#60682,#60683,#60684,#60685,#60686,#60687,#60688,#60689,#60690,#60691,#60692,
#60693,#60694,#60695,#60696,#60697,#60698,#60699,#60700,#60701,#60702,#60703,
#60704,#60705,#60706,#60707,#60708,#60709,#60710,#60711,#60712,#60713,#60714,
#60715,#60716,#60717,#60718,#60719,#60720,#60721,#60722,#60723,#60724,#60725,
#60726,#60727,#60728,#60729,#60730,#60731,#60732,#60733,#60734,#60735,#60736,
#60737,#60738,#60739,#60740,#60741,#60742,#60743,#60744,#60745,#60746,#60747,
#60748,#60749,#60750,#60751,#60752,#60753,#60754,#60755,#60756,#60757,#60758,
#60759,#60760,#60761,#60762,#60763,#60764,#60765,#60766,#60767,#60768,#60769,
#60770,#60771,#60772,#60773,#60774,#60775,#60776,#60777,#60778,#60779,#60780,
#60781,#60782,#60783,#60784,#60785,#60786,#60787,#60788,#60789,#60790,#60791,
#60792,#60793,#60794,#60795,#60796,#60797,#60798,#60799,#60800,#60801,#60802,
#60803,#60804,#60805,#60806,#60807,#60808,#60809,#60810),.UNSPECIFIED.,
 .F.,.F.,(4,2,2,2,2,2,2,2,2,2,2,2,2,2,2,2,2,2,2,2,2,2,2,2,2,2,2,2,2,2,2,
2,2,2,2,2,2,2,2,2,2,2,2,2,2,2,2,2,2,2,2,2,2,2,2,2,2,2,2,2,2,2,2,2,2,2,2,
2,2,2,2,2,2,2,2,2,2,4),(-0.912207559110817,-0.904370165018042,-0.898370552967401,
-0.892906950896839,-0.885368518653862,-0.859004877746807,-0.846026001349283,
-0.837931341722297,-0.834222107250463,-0.831082361507067,-0.826290219671332,
-0.802745556480474,-0.781907852870987,-0.774180285949588,-0.768691256216211,
-0.762762661445065,-0.752320124607763,-0.737959821906094,-0.712753076978956,
-0.708134615440343,-0.705016407763125,-0.701214897319066,-0.692496119353534,
-0.677741073643799,-0.654596569845275,-0.646837505688292,-0.641344129898751,
-0.635426541025622,-0.625051280915556,-0.610841403772924,-0.585288240426161,
-0.580708109696272,-0.577594080775163,-0.573769985347027,-0.564890782074043,
-0.5496450193943,-0.527232792518649,-0.519465674065646,-0.513971162216523,
-0.508056312617709,-0.497697863482222,-0.483525402616645,-0.457884935306767,
-0.453314591437652,-0.450201581226279,-0.446371545490143,-0.437449679017519,
-0.422070873728227,-0.399848281471212,-0.392082141709777,-0.386587747014567,
-0.380672524523701,-0.37031191181269,-0.356134682483944,-0.330505082013807,
-0.32593348053507,-0.322820327675395,-0.318991027074598,-0.310074542004067,
-0.294712639716686,-0.272465930605739,-0.264699561163723,-0.259205115734093,
-0.253289935586837,-0.242929690592456,-0.228753315889827,-0.20312147323728,
-0.198550092769763,-0.195436951782767,-0.191607488944604,-0.182689913914197,
-0.167324653862376,-0.145082514942491,-0.137316149014768,-0.131821685233644,
-0.125906467248585,-0.115546101238224,-0.109987797047057),.UNSPECIFIED.);
#713=B_SPLINE_CURVE_WITH_KNOTS('',3,(#60815,#60816,#60817,#60818,#60819,
#60820,#60821,#60822,#60823,#60824,#60825,#60826,#60827,#60828,#60829,#60830,
#60831,#60832,#60833,#60834,#60835,#60836,#60837,#60838,#60839,#60840,#60841,
#60842,#60843,#60844,#60845,#60846,#60847,#60848,#60849,#60850,#60851,#60852,
#60853,#60854,#60855,#60856,#60857,#60858,#60859,#60860,#60861,#60862,#60863,
#60864,#60865,#60866,#60867,#60868,#60869,#60870,#60871,#60872,#60873,#60874,
#60875,#60876,#60877,#60878,#60879,#60880,#60881,#60882,#60883,#60884,#60885,
#60886,#60887,#60888,#60889,#60890,#60891,#60892,#60893,#60894,#60895,#60896,
#60897,#60898,#60899,#60900,#60901,#60902,#60903,#60904,#60905,#60906,#60907,
#60908,#60909,#60910,#60911,#60912,#60913,#60914,#60915,#60916,#60917,#60918,
#60919,#60920,#60921,#60922,#60923,#60924,#60925,#60926,#60927,#60928,#60929,
#60930,#60931,#60932,#60933,#60934,#60935,#60936,#60937,#60938,#60939,#60940,
#60941,#60942,#60943,#60944,#60945,#60946,#60947,#60948,#60949,#60950,#60951,
#60952,#60953,#60954,#60955,#60956,#60957,#60958,#60959,#60960,#60961,#60962,
#60963,#60964,#60965,#60966,#60967,#60968,#60969,#60970),.UNSPECIFIED.,
 .F.,.F.,(4,2,2,2,2,2,2,2,2,2,2,2,2,2,2,2,2,2,2,2,2,2,2,2,2,2,2,2,2,2,2,
2,2,2,2,2,2,2,2,2,2,2,2,2,2,2,2,2,2,2,2,2,2,2,2,2,2,2,2,2,2,2,2,2,2,2,2,
2,2,2,2,2,2,2,2,2,2,4),(-1.49501924537234,-1.4813148627293,-1.4680560708403,
-1.45985967772397,-1.45613571858057,-1.45300108845073,-1.44824188592874,
-1.42441831558675,-1.40947559509268,-1.39877973307688,-1.39281157526604,
-1.38733914050731,-1.37972551975406,-1.36135837627754,-1.3392218732596,
-1.33204697502592,-1.32848721336543,-1.32533156571223,-1.3202210330441,
-1.30334686340635,-1.28450939122364,-1.27232355275591,-1.26612681232264,
-1.26070911642611,-1.25370128228088,-1.223683914122,-1.21231884988458,-1.20485647270919,
-1.20124821922491,-1.19811194125785,-1.19312727429328,-1.16698170234289,
-1.14721464618892,-1.1402747148536,-1.13487197761727,-1.12855288409598,
-1.11549579071886,-1.09015955699211,-1.0845256833055,-1.07735056944568,
-1.07379032513158,-1.07063398630341,-1.06552193230557,-1.04852546653233,
-1.02976380151225,-1.01760252893791,-1.01140849831093,-1.00598913462564,
-0.998973454584765,-0.968999378925303,-0.957612454266797,-0.950140546560794,
-0.946530264797707,-0.94339388808695,-0.93841158710968,-0.916919533769083,
-0.900843325589779,-0.895540675846777,-0.887302561368203,-0.881737349025378,
-0.875957444673054,-0.866415137657659,-0.836302707806108,-0.824285207096203,
-0.820102754030312,-0.817013494298257,-0.812957478266099,-0.802620066898701,
-0.781287309984028,-0.764815006180216,-0.757981913640745,-0.752583991849499,
-0.746183167213547,-0.732509174772806,-0.708505726807608,-0.69705333904176,
-0.693221201266409,-0.692954581112378),.UNSPECIFIED.);
#714=B_SPLINE_CURVE_WITH_KNOTS('',3,(#60972,#60973,#60974,#60975,#60976,
#60977,#60978,#60979,#60980,#60981,#60982,#60983,#60984,#60985,#60986,#60987,
#60988,#60989,#60990,#60991,#60992,#60993,#60994,#60995),.UNSPECIFIED.,
 .F.,.F.,(4,2,2,2,2,2,2,2,2,2,2,4),(-0.109987797047057,-0.101369495396899,
-0.075737941276712,-0.0711664964469346,-0.0680533374928693,-0.0642238855499439,
-0.0553064687578774,-0.0311046932610105,-0.0150614501695526,-0.00846605047845859,
-0.00415225361026194,-0.000375256628440777),.UNSPECIFIED.);
#715=B_SPLINE_CURVE_WITH_KNOTS('',3,(#60996,#60997,#60998,#60999,#61000,
#61001,#61002,#61003,#61004,#61005,#61006,#61007,#61008,#61009,#61010,#61011,
#61012,#61013,#61014,#61015,#61016,#61017,#61018,#61019,#61020,#61021,#61022,
#61023,#61024,#61025,#61026,#61027,#61028,#61029,#61030,#61031,#61032,#61033,
#61034,#61035,#61036,#61037,#61038,#61039,#61040,#61041,#61042,#61043,#61044,
#61045,#61046,#61047,#61048,#61049,#61050,#61051,#61052,#61053,#61054,#61055,
#61056,#61057,#61058,#61059,#61060,#61061,#61062,#61063,#61064,#61065,#61066,
#61067,#61068,#61069,#61070,#61071,#61072,#61073,#61074,#61075,#61076,#61077,
#61078,#61079,#61080,#61081,#61082,#61083,#61084,#61085,#61086,#61087,#61088,
#61089,#61090,#61091,#61092,#61093,#61094,#61095,#61096,#61097,#61098,#61099,
#61100,#61101,#61102,#61103,#61104,#61105,#61106,#61107,#61108,#61109,#61110,
#61111,#61112,#61113,#61114,#61115,#61116,#61117,#61118,#61119,#61120,#61121,
#61122,#61123,#61124,#61125,#61126,#61127,#61128,#61129),.UNSPECIFIED.,
 .F.,.F.,(4,2,2,2,2,2,2,2,2,2,2,2,2,2,2,2,2,2,2,2,2,2,2,2,2,2,2,2,2,2,2,
2,2,2,2,2,2,2,2,2,2,2,2,2,2,2,2,2,2,2,2,2,2,2,2,2,2,2,2,2,2,2,2,2,2,2,4),
(-1.60449821208469,-1.60117471261476,-1.5964950956904,-1.57927261005758,
-1.55964101744956,-1.55073034444578,-1.54690289634666,-1.54379106829042,
-1.5392214159838,-1.51363830730631,-1.49947413214974,-1.48912065473405,
-1.48320849903881,-1.47771605866567,-1.46995134538992,-1.44716422048722,
-1.43215693757249,-1.42335600900917,-1.41954376404826,-1.41642901785842,
-1.41183336949047,-1.38647980163793,-1.37221523595865,-1.36181650035951,
-1.35589671095472,-1.35040691634006,-1.34266296414325,-1.31903487511374,
-1.30456705053649,-1.29594528770798,-1.29215839630123,-1.28903848600272,
-1.28439822543246,-1.25944944744898,-1.24500617328139,-1.23452766812593,
-1.22859461485906,-1.22310952751012,-1.21540170343605,-1.19105122703047,
-1.1770120704431,-1.16853703489118,-1.16477128929525,-1.16164658806205,
-1.15696730819572,-1.13237787336056,-1.11777328673824,-1.10722343391458,
-1.10127850483346,-1.09579736075833,-1.08812072654645,-1.06330042126066,
-1.04952425952151,-1.04114113150227,-1.03738875342865,-1.03426069615257,
-1.02955558930728,-1.00520370460247,-0.990490798635368,-0.979893298103208,
-0.973940345202394,-0.968461572877665,-0.960804945540949,-0.941597207766749,
-0.920368754853509,-0.913200300898691,-0.91205896481613),.UNSPECIFIED.);
#716=B_SPLINE_CURVE_WITH_KNOTS('',3,(#61135,#61136,#61137,#61138,#61139,
#61140,#61141,#61142,#61143,#61144,#61145,#61146,#61147,#61148,#61149,#61150,
#61151,#61152,#61153,#61154,#61155,#61156,#61157,#61158,#61159,#61160,#61161,
#61162,#61163,#61164,#61165,#61166,#61167,#61168,#61169,#61170,#61171,#61172,
#61173,#61174,#61175,#61176,#61177,#61178,#61179,#61180,#61181,#61182,#61183,
#61184,#61185,#61186,#61187,#61188,#61189,#61190,#61191,#61192,#61193,#61194,
#61195,#61196,#61197,#61198,#61199,#61200,#61201,#61202,#61203,#61204,#61205,
#61206,#61207,#61208,#61209,#61210,#61211,#61212,#61213,#61214,#61215,#61216,
#61217,#61218,#61219,#61220,#61221,#61222,#61223,#61224,#61225,#61226,#61227,
#61228,#61229,#61230,#61231,#61232,#61233,#61234,#61235,#61236,#61237,#61238,
#61239,#61240,#61241,#61242,#61243,#61244,#61245,#61246,#61247,#61248,#61249,
#61250,#61251,#61252,#61253,#61254,#61255,#61256,#61257,#61258,#61259,#61260,
#61261,#61262,#61263,#61264,#61265,#61266,#61267,#61268),.UNSPECIFIED.,
 .F.,.F.,(4,2,2,2,2,2,2,2,2,2,2,2,2,2,2,2,2,2,2,2,2,2,2,2,2,2,2,2,2,2,2,
2,2,2,2,2,2,2,2,2,2,2,2,2,2,2,2,2,2,2,2,2,2,2,2,2,2,2,2,2,2,2,2,2,2,2,4),
(-0.693092190322639,-0.69015751324097,-0.683629814231713,-0.678135474982164,
-0.672219676221536,-0.66185585975289,-0.647671272007037,-0.622063065460699,
-0.617489398199346,-0.614375868776239,-0.610547105340709,-0.601636182823502,
-0.586291488509274,-0.564025137267241,-0.556258413123572,-0.550763259234434,
-0.544846718803061,-0.534481498986856,-0.520294010175215,-0.494696856336391,
-0.490121956830987,-0.487008036423791,-0.483179390638319,-0.474269339850772,
-0.458927345536385,-0.436657672917112,-0.428891116117865,-0.423396145940555,
-0.417479898096204,-0.407115695748478,-0.392930632900304,-0.367324168061133,
-0.362750151519772,-0.359636451799163,-0.355807641911074,-0.346896099110626,
-0.331549403124372,-0.309285851925463,-0.30151931723584,-0.296024383199857,
-0.290108201420297,-0.279744208456879,-0.265559527413953,-0.239952679004846,
-0.235378741065102,-0.232265027776118,-0.228436081640495,-0.219523849181067,
-0.204175110058433,-0.181914328415961,-0.174147724031108,-0.168652691117248,
-0.1627363451117,-0.152371828144423,-0.138186047639759,-0.112582005190155,
-0.108007722257923,-0.104893934068742,-0.101065105805702,-0.0921537708571086,
-0.0768078722055855,-0.0545429654360646,-0.0467763330896944,-0.0412813060508978,
-0.0353649943164301,-0.0291760048854813,-0.000377328695443869),
 .UNSPECIFIED.);
#717=B_SPLINE_CURVE_WITH_KNOTS('',3,(#61269,#61270,#61271,#61272,#61273,
#61274,#61275,#61276,#61277,#61278,#61279,#61280,#61281,#61282,#61283,#61284,
#61285,#61286,#61287,#61288,#61289,#61290,#61291,#61292,#61293,#61294),
 .UNSPECIFIED.,.F.,.F.,(4,2,2,2,2,2,2,2,2,2,2,2,4),(-1.6044068850231,-1.58965030014154,
-1.58600505033392,-1.58313059790593,-1.57997861077168,-1.57488842166979,
-1.55622031234691,-1.53687287755627,-1.52612913631752,-1.5201536495453,
-1.51468433454594,-1.5070915873584,-1.49501924537234),.UNSPECIFIED.);
#718=B_SPLINE_CURVE_WITH_KNOTS('',3,(#61295,#61296,#61297,#61298,#61299,
#61300,#61301,#61302,#61303,#61304,#61305,#61306,#61307,#61308,#61309,#61310,
#61311,#61312,#61313,#61314,#61315,#61316,#61317,#61318,#61319,#61320,#61321,
#61322,#61323,#61324,#61325,#61326,#61327,#61328,#61329,#61330,#61331,#61332,
#61333,#61334,#61335,#61336,#61337,#61338,#61339,#61340,#61341,#61342,#61343,
#61344,#61345,#61346,#61347,#61348,#61349,#61350,#61351,#61352,#61353,#61354,
#61355,#61356,#61357,#61358,#61359,#61360,#61361,#61362,#61363,#61364,#61365,
#61366,#61367,#61368,#61369,#61370,#61371,#61372,#61373,#61374,#61375,#61376,
#61377,#61378,#61379,#61380,#61381,#61382,#61383,#61384,#61385,#61386,#61387,
#61388,#61389,#61390,#61391,#61392,#61393,#61394,#61395,#61396,#61397,#61398,
#61399,#61400,#61401,#61402,#61403,#61404,#61405,#61406,#61407,#61408,#61409,
#61410,#61411,#61412,#61413,#61414,#61415,#61416,#61417,#61418,#61419,#61420,
#61421,#61422,#61423,#61424,#61425,#61426,#61427,#61428,#61429,#61430,#61431,
#61432,#61433,#61434,#61435,#61436,#61437,#61438,#61439,#61440,#61441,#61442,
#61443,#61444,#61445,#61446,#61447,#61448,#61449,#61450),.UNSPECIFIED.,
 .F.,.F.,(4,2,2,2,2,2,2,2,2,2,2,2,2,2,2,2,2,2,2,2,2,2,2,2,2,2,2,2,2,2,2,
2,2,2,2,2,2,2,2,2,2,2,2,2,2,2,2,2,2,2,2,2,2,2,2,2,2,2,2,2,2,2,2,2,2,2,2,
2,2,2,2,2,2,2,2,2,2,4),(-0.91205896481613,-0.909641274075211,-0.906484757659767,
-0.901370813566233,-0.883580462577556,-0.865336335945879,-0.853353310013507,
-0.847185477149381,-0.841762079830826,-0.834703030030153,-0.802386647355041,
-0.788162487199457,-0.78368682748423,-0.780582916630038,-0.776692340219932,
-0.7673210843246,-0.750468369436933,-0.730191570429174,-0.722488183294921,
-0.717002468854449,-0.711065268165521,-0.700569900903023,-0.686090510172526,
-0.661154549454114,-0.656506695364241,-0.653385135258693,-0.649600352511887,
-0.640998333487524,-0.626591103568252,-0.602893192725773,-0.59515264780876,
-0.589661864442072,-0.583737896584683,-0.573323485776892,-0.559026165743644,
-0.533675502827674,-0.529072911650881,-0.525956483314419,-0.522145786804655,
-0.513361985762053,-0.498409770813735,-0.475566300732396,-0.467801680461069,
-0.462307564151859,-0.456391951088547,-0.446028567705263,-0.431845053560707,
-0.406230905898853,-0.40165767015328,-0.398544387244274,-0.394716183375895,
-0.385807319102666,-0.37046908015249,-0.348189297192809,-0.340422788135625,
-0.334928386813119,-0.329013379124437,-0.318653814887083,-0.304478820778654,
-0.278844633442578,-0.274273621962933,-0.27116054542505,-0.267330907141639,
-0.258411916877638,-0.243042049144117,-0.22080730784035,-0.213041109021085,
-0.207546705730238,-0.201631496399774,-0.191270958101461,-0.177093877680558,
-0.151464194025713,-0.146892634147559,-0.143779507584902,-0.139950258764867,
-0.131033882126756,-0.115672220255292,-0.109848755237784),.UNSPECIFIED.);
#719=B_SPLINE_CURVE_WITH_KNOTS('',3,(#61455,#61456,#61457,#61458,#61459,
#61460,#61461,#61462,#61463,#61464,#61465,#61466,#61467,#61468,#61469,#61470,
#61471,#61472,#61473,#61474,#61475,#61476,#61477,#61478,#61479,#61480,#61481,
#61482,#61483,#61484,#61485,#61486,#61487,#61488,#61489,#61490,#61491,#61492,
#61493,#61494,#61495,#61496,#61497,#61498,#61499,#61500,#61501,#61502,#61503,
#61504,#61505,#61506,#61507,#61508,#61509,#61510,#61511,#61512,#61513,#61514,
#61515,#61516,#61517,#61518,#61519,#61520,#61521,#61522,#61523,#61524,#61525,
#61526,#61527,#61528,#61529,#61530,#61531,#61532,#61533,#61534,#61535,#61536,
#61537,#61538,#61539,#61540,#61541,#61542,#61543,#61544,#61545,#61546,#61547,
#61548,#61549,#61550,#61551,#61552,#61553,#61554,#61555,#61556,#61557,#61558,
#61559,#61560,#61561,#61562,#61563,#61564,#61565,#61566,#61567,#61568,#61569,
#61570,#61571,#61572,#61573,#61574,#61575,#61576,#61577,#61578,#61579,#61580,
#61581,#61582,#61583,#61584,#61585,#61586,#61587,#61588,#61589,#61590,#61591,
#61592,#61593,#61594,#61595,#61596,#61597,#61598,#61599,#61600,#61601,#61602,
#61603,#61604),.UNSPECIFIED.,.F.,.F.,(4,2,2,2,2,2,2,2,2,2,2,2,2,2,2,2,2,
2,2,2,2,2,2,2,2,2,2,2,2,2,2,2,2,2,2,2,2,2,2,2,2,2,2,2,2,2,2,2,2,2,2,2,2,
2,2,2,2,2,2,2,2,2,2,2,2,2,2,2,2,2,2,2,2,2,4),(-1.49514144568264,-1.47438857105786,
-1.46045849771916,-1.45022305357444,-1.44435288172889,-1.43889105456154,
-1.43116435290765,-1.40722401557869,-1.39283837472975,-1.38424761820676,
-1.38047920020778,-1.37736852119829,-1.37275211016375,-1.34755948942701,
-1.3332063100285,-1.32276142634397,-1.31682570935194,-1.31132487155196,
-1.30356762536673,-1.28058029495704,-1.26579136510866,-1.25706287817131,
-1.25325415294809,-1.25012853345904,-1.24548894090294,-1.22051819483855,
-1.20609396748146,-1.1956236845839,-1.18968929617281,-1.18419905470653,
-1.17647659214743,-1.15227168670788,-1.1381312685222,-1.12961958896452,
-1.1258477102684,-1.12272495591843,-1.11805801926491,-1.09336125123812,
-1.07880424687313,-1.06827635035556,-1.06233706940999,-1.05685815177955,
-1.04918041937155,-1.02437341766863,-1.01057935952288,-1.00219012882368,
-0.998438102967066,-0.995310611511707,-0.990608829365062,-0.966217676459732,
-0.951520438289615,-0.940928504456857,-0.934974506764387,-0.929492180425934,
-0.921825366122576,-0.902404848674383,-0.881301853283018,-0.874215287049936,
-0.870668989897699,-0.867504006166135,-0.862343635961059,-0.842881735424566,
-0.825765477070716,-0.814192386661388,-0.808084946221302,-0.802647876831401,
-0.795342854681945,-0.772617796786585,-0.750144313039306,-0.745236044253845,
-0.742110626730573,-0.738469454742124,-0.730808221723706,-0.718954873859401,
-0.693092190322639),.UNSPECIFIED.);
#720=B_SPLINE_CURVE_WITH_KNOTS('',3,(#61606,#61607,#61608,#61609,#61610,
#61611,#61612,#61613,#61614,#61615,#61616,#61617,#61618,#61619,#61620,#61621,
#61622,#61623,#61624,#61625,#61626,#61627,#61628,#61629,#61630,#61631),
 .UNSPECIFIED.,.F.,.F.,(4,2,2,2,2,2,2,2,2,2,2,2,4),(-0.109848755237784,
-0.0934252676034876,-0.0856589675731766,-0.0801646032460511,-0.0742495478951926,
-0.0643588753228271,-0.0439802194508923,-0.025130067662574,-0.0200474136688195,
-0.016895840425231,-0.0140198172539918,-0.0103707398875634,-0.0003752626807542),
 .UNSPECIFIED.);
#721=B_SPLINE_CURVE_WITH_KNOTS('',3,(#61632,#61633,#61634,#61635,#61636,
#61637,#61638,#61639,#61640,#61641,#61642,#61643,#61644,#61645,#61646,#61647,
#61648,#61649,#61650,#61651,#61652,#61653,#61654,#61655,#61656,#61657,#61658,
#61659,#61660,#61661,#61662,#61663,#61664,#61665,#61666,#61667,#61668,#61669,
#61670,#61671,#61672,#61673,#61674,#61675,#61676,#61677,#61678,#61679,#61680,
#61681,#61682,#61683,#61684,#61685,#61686,#61687,#61688,#61689,#61690,#61691,
#61692,#61693,#61694,#61695,#61696,#61697,#61698,#61699,#61700,#61701,#61702,
#61703,#61704,#61705,#61706,#61707,#61708,#61709,#61710,#61711,#61712,#61713,
#61714,#61715,#61716,#61717,#61718,#61719,#61720,#61721,#61722,#61723,#61724,
#61725,#61726,#61727,#61728,#61729,#61730,#61731,#61732,#61733,#61734,#61735,
#61736,#61737,#61738,#61739,#61740,#61741,#61742,#61743,#61744,#61745,#61746,
#61747,#61748,#61749,#61750,#61751,#61752,#61753,#61754,#61755,#61756,#61757,
#61758,#61759,#61760,#61761,#61762,#61763,#61764,#61765,#61766,#61767,#61768,
#61769,#61770,#61771,#61772,#61773,#61774,#61775,#61776,#61777,#61778,#61779),
 .UNSPECIFIED.,.F.,.F.,(4,3,3,3,3,3,3,3,3,3,3,3,3,3,3,3,3,3,3,3,3,3,3,3,
3,3,3,3,3,3,3,3,3,3,3,3,3,3,3,3,3,3,3,3,3,3,3,3,3,4),(59.6902604187055,
59.8059365886586,59.9214749790758,60.0369282464819,60.1523488894859,60.2678696341567,
60.3834462962811,60.4992335231002,60.5534341867985,60.6709356877518,60.7882209063099,
60.9053869875018,61.0224839148767,61.1395615592371,61.2567536125899,61.3740087054347,
61.491482903214,61.5511221063311,61.6686207302785,61.7859030669755,61.9030662657053,
62.0201603153612,62.1372350920866,62.2544243155958,62.3716765959422,62.4891480410998,
62.5488100258638,62.6663133455865,62.7836003454799,62.9007681834644,63.0178668401377,
63.1349461833192,63.2521398766191,63.3693965783365,63.4868723183997,63.5464979453964,
63.6640025093476,63.7812908428973,63.8984600685255,64.0155601635914,64.1326409927496,
64.2498362310647,64.3670945136204,64.4845718705366,64.5441858649291,64.6616585799595,
64.7789258711664,64.8960709870156,65.0131746409143,65.1150562521972),
 .UNSPECIFIED.);
#722=B_SPLINE_CURVE_WITH_KNOTS('',3,(#61783,#61784,#61785,#61786,#61787,
#61788,#61789,#61790,#61791,#61792,#61793,#61794,#61795,#61796,#61797,#61798,
#61799,#61800,#61801,#61802,#61803,#61804,#61805,#61806,#61807,#61808,#61809,
#61810,#61811,#61812,#61813,#61814,#61815,#61816,#61817,#61818,#61819,#61820,
#61821,#61822,#61823,#61824,#61825,#61826,#61827,#61828,#61829,#61830,#61831,
#61832,#61833,#61834,#61835,#61836,#61837,#61838,#61839,#61840,#61841,#61842,
#61843),.UNSPECIFIED.,.F.,.F.,(4,3,3,3,3,3,3,3,3,3,3,3,3,3,3,3,3,3,3,3,
4),(-4.04123713824999,-3.99075167813058,-3.88138448277551,-3.77034439225331,
-3.66127980526779,-3.55228313954551,-3.44331469571073,-3.33075196143253,
-3.22165200987809,-3.10735788423801,-2.99306375859793,-2.88381609209196,
-2.77276106046363,-2.66380817130367,-2.5549200056019,-2.44605671409851,
-2.33338649534021,-2.22438227090265,-2.10987905498397,-1.99537583906529,
-1.98502202421796),.UNSPECIFIED.);
#723=B_SPLINE_CURVE_WITH_KNOTS('',3,(#61847,#61848,#61849,#61850,#61851),
 .UNSPECIFIED.,.F.,.F.,(4,1,4),(0.,0.997687919532644,1.08537753955778),
 .UNSPECIFIED.);
#724=B_SPLINE_CURVE_WITH_KNOTS('',3,(#61853,#61854,#61855,#61856,#61857,
#61858,#61859,#61860,#61861,#61862,#61863,#61864,#61865,#61866,#61867,#61868,
#61869,#61870,#61871,#61872,#61873,#61874,#61875,#61876,#61877,#61878,#61879,
#61880,#61881,#61882,#61883,#61884,#61885,#61886,#61887,#61888,#61889,#61890,
#61891,#61892,#61893,#61894,#61895,#61896,#61897,#61898,#61899,#61900,#61901,
#61902,#61903,#61904,#61905,#61906,#61907,#61908,#61909,#61910,#61911,#61912,
#61913,#61914,#61915,#61916,#61917,#61918,#61919,#61920,#61921,#61922,#61923,
#61924,#61925,#61926,#61927,#61928,#61929,#61930,#61931,#61932,#61933,#61934,
#61935,#61936,#61937,#61938,#61939,#61940,#61941,#61942,#61943,#61944,#61945,
#61946,#61947,#61948,#61949,#61950,#61951,#61952,#61953,#61954,#61955,#61956,
#61957,#61958,#61959,#61960,#61961,#61962,#61963,#61964,#61965,#61966,#61967,
#61968,#61969,#61970,#61971,#61972,#61973,#61974,#61975,#61976,#61977,#61978,
#61979,#61980,#61981,#61982,#61983,#61984,#61985,#61986,#61987,#61988,#61989,
#61990,#61991,#61992,#61993,#61994,#61995,#61996,#61997,#61998,#61999,#62000,
#62001,#62002,#62003,#62004,#62005,#62006,#62007,#62008,#62009,#62010,#62011,
#62012,#62013,#62014,#62015,#62016,#62017,#62018,#62019,#62020,#62021,#62022,
#62023,#62024,#62025,#62026,#62027,#62028,#62029,#62030),.UNSPECIFIED.,
 .F.,.F.,(4,3,3,3,3,3,3,3,3,3,3,3,3,3,3,3,3,3,3,3,3,3,3,3,3,3,3,3,3,3,3,
3,3,3,3,3,3,3,3,3,3,3,3,3,3,3,3,3,3,3,3,3,3,3,3,3,3,3,3,4),(1.08537753955778,
1.19234574493029,1.29913105914354,1.40581587747835,1.51244291764453,1.61905479404571,
1.72576691819386,1.83253406091469,1.93949157832785,1.99537583906529,2.10463715419484,
2.21569047974523,2.32464897406955,2.43353974323111,2.54240264139813,2.65506792069808,
2.7640643232495,2.87856404092371,2.99306375859793,3.10241206764536,3.21345451895602,
3.32251126192849,3.43150420770341,3.54047304919539,3.65304270642919,3.76215325291235,
3.87645246552146,3.99075167813058,4.09980427302158,4.21088368860178,4.3196319345462,
4.42831248282007,4.53696553861079,4.64983405337389,4.75862402872994,4.86749101609525,
4.97653965670554,4.98843959766322,5.09762857242077,5.20869094051765,5.3175794422449,
5.42640130271024,5.5351964991536,5.64792925366416,5.75686180175626,5.87149465947606,
5.98612751719586,6.0953168100183,6.20637913835707,6.31526902205822,6.42409265844288,
6.53289002301757,6.64562137644531,6.75455705278224,6.86918624475538,6.98381543672851,
7.10632262234372,7.22836033829121,7.34964575624075,7.36856284629316),
 .UNSPECIFIED.);
#725=B_SPLINE_CURVE_WITH_KNOTS('',3,(#62032,#62033,#62034,#62035,#62036,
#62037,#62038,#62039,#62040,#62041,#62042,#62043,#62044,#62045,#62046,#62047,
#62048,#62049,#62050,#62051,#62052,#62053,#62054,#62055,#62056,#62057,#62058,
#62059,#62060,#62061,#62062,#62063,#62064,#62065,#62066,#62067,#62068,#62069,
#62070,#62071,#62072,#62073,#62074,#62075,#62076,#62077,#62078,#62079,#62080,
#62081,#62082,#62083,#62084,#62085,#62086,#62087,#62088,#62089,#62090,#62091,
#62092,#62093,#62094,#62095,#62096,#62097,#62098,#62099,#62100,#62101,#62102,
#62103,#62104,#62105,#62106,#62107,#62108,#62109,#62110,#62111,#62112,#62113,
#62114,#62115,#62116,#62117,#62118,#62119,#62120,#62121,#62122,#62123,#62124,
#62125,#62126,#62127,#62128,#62129,#62130,#62131,#62132,#62133,#62134,#62135,
#62136,#62137,#62138,#62139,#62140,#62141,#62142,#62143,#62144,#62145,#62146,
#62147,#62148,#62149,#62150,#62151,#62152,#62153,#62154,#62155,#62156,#62157,
#62158,#62159,#62160,#62161,#62162,#62163,#62164,#62165,#62166,#62167,#62168,
#62169,#62170,#62171,#62172,#62173,#62174,#62175,#62176,#62177,#62178,#62179,
#62180,#62181,#62182,#62183,#62184,#62185,#62186,#62187,#62188,#62189,#62190,
#62191,#62192,#62193,#62194,#62195,#62196,#62197,#62198,#62199,#62200,#62201,
#62202,#62203,#62204,#62205,#62206),.UNSPECIFIED.,.F.,.F.,(4,3,3,3,3,3,
3,3,3,3,3,3,3,3,3,3,3,3,3,3,3,3,3,3,3,3,3,3,3,3,3,3,3,3,3,3,3,3,3,3,3,3,
3,3,3,3,3,3,3,3,3,3,3,3,3,3,3,3,4),(7.36856284673735,7.4784069249757,7.58827792776978,
7.69829983037369,7.8084040130256,7.91873166272418,7.98150335626115,8.09067677218719,
8.20174108513802,8.31061410652896,8.41942055999989,8.5282004487066,8.64094815547839,
8.74986582499829,8.86452855039604,8.97919127579379,9.08836318751633,9.19942768849259,
9.30829928229541,9.41710434087364,9.5258828698046,9.63863195118506,9.7475483651341,
9.86221378023027,9.97687919532644,10.0860471500499,10.1971121456511,10.3059795915811,
10.4147804426623,10.523554711276,10.6363078121718,10.7452198829806,10.8598934989198,
10.9745671148591,11.0837376091672,11.1948022873202,11.3036723575658,11.4124758572139,
11.5212527943222,11.6340033543396,11.7429181124569,11.8575865734243,11.9722550343917,
12.0814251445948,12.192489870761,12.3013595589726,12.410162678443,12.5189392378677,
12.6316901668819,12.7406045580105,12.8552737559675,12.9699429539244,13.078724484454,
13.1873437619597,13.2958416021516,13.4042699324801,13.5126593842041,13.621079592138,
13.651748153917),.UNSPECIFIED.);
#726=B_SPLINE_CURVE_WITH_KNOTS('',3,(#62208,#62209,#62210,#62211,#62212,
#62213,#62214,#62215,#62216,#62217,#62218,#62219,#62220,#62221,#62222,#62223,
#62224,#62225,#62226,#62227,#62228,#62229,#62230,#62231,#62232,#62233,#62234,
#62235,#62236,#62237,#62238,#62239,#62240,#62241,#62242,#62243,#62244,#62245,
#62246,#62247,#62248,#62249,#62250,#62251,#62252,#62253,#62254,#62255,#62256,
#62257,#62258,#62259,#62260,#62261,#62262,#62263,#62264,#62265,#62266,#62267,
#62268,#62269,#62270,#62271,#62272,#62273,#62274,#62275,#62276,#62277,#62278,
#62279,#62280,#62281,#62282,#62283,#62284,#62285,#62286,#62287,#62288,#62289,
#62290,#62291,#62292,#62293,#62294,#62295,#62296,#62297,#62298,#62299,#62300,
#62301,#62302,#62303,#62304,#62305,#62306,#62307,#62308,#62309,#62310,#62311,
#62312,#62313,#62314,#62315,#62316,#62317,#62318,#62319,#62320,#62321,#62322,
#62323,#62324,#62325,#62326,#62327,#62328,#62329,#62330,#62331,#62332,#62333,
#62334,#62335,#62336,#62337,#62338,#62339,#62340,#62341,#62342,#62343,#62344,
#62345,#62346,#62347,#62348,#62349,#62350,#62351,#62352,#62353,#62354,#62355,
#62356,#62357,#62358,#62359,#62360,#62361,#62362,#62363,#62364,#62365,#62366,
#62367,#62368,#62369,#62370,#62371,#62372,#62373,#62374,#62375,#62376,#62377,
#62378,#62379),.UNSPECIFIED.,.F.,.F.,(4,3,3,3,3,3,3,3,3,3,3,3,3,3,3,3,3,
3,3,3,3,3,3,3,3,3,3,3,3,3,3,3,3,3,3,3,3,3,3,3,3,3,3,3,3,3,3,3,3,3,3,3,3,
3,3,3,3,4),(13.6517481543043,13.7804829473712,13.9108082109149,13.967630873457,
14.0768008840177,14.1878656226392,14.2967352004234,14.4055382057466,14.5143146474821,
14.627065683859,14.7359799497759,14.8506493713828,14.9653187929896,15.0744887311938,
15.1855534788599,15.2944229835671,15.4032259157507,15.5120022844056,15.6247533914348,
15.7336675852756,15.8483371488989,15.9630067125223,16.0721766057685,16.1832413590543,
16.2921108162111,16.4009137000096,16.5096900195225,16.6224411726556,16.7313553160279,
16.8460249740414,16.9606946320549,17.0698645681445,17.1809293160749,17.2897988176718,
17.3986017463818,17.5073781112041,17.6201292213,17.7290434104513,17.8437129810194,
17.9583825515876,18.0675524756807,18.1786172251106,18.2874867144961,18.3962896309488,
18.5050659834882,18.6178171053962,18.7267312823442,18.8414008767322,18.9560704711202,
19.0648897450418,19.1736452095118,19.2821672095361,19.3906233509149,19.4990541980267,
19.6080240137205,19.7165924406379,19.8257629507199,19.9349334608019),
 .UNSPECIFIED.);
#727=B_SPLINE_CURVE_WITH_KNOTS('',3,(#62381,#62382,#62383,#62384,#62385,
#62386,#62387,#62388,#62389,#62390,#62391,#62392,#62393,#62394,#62395,#62396,
#62397,#62398,#62399,#62400,#62401,#62402,#62403,#62404,#62405,#62406,#62407,
#62408,#62409,#62410,#62411,#62412,#62413,#62414,#62415,#62416,#62417,#62418,
#62419,#62420,#62421,#62422,#62423,#62424,#62425,#62426,#62427,#62428,#62429,
#62430,#62431,#62432,#62433,#62434,#62435,#62436,#62437,#62438,#62439,#62440,
#62441,#62442,#62443,#62444,#62445,#62446,#62447,#62448,#62449,#62450,#62451,
#62452,#62453,#62454,#62455,#62456,#62457,#62458,#62459,#62460,#62461,#62462,
#62463,#62464,#62465,#62466,#62467,#62468,#62469,#62470,#62471,#62472,#62473,
#62474,#62475,#62476,#62477,#62478,#62479,#62480,#62481,#62482,#62483,#62484,
#62485,#62486,#62487,#62488,#62489,#62490,#62491,#62492,#62493,#62494,#62495,
#62496,#62497,#62498,#62499,#62500,#62501,#62502,#62503,#62504,#62505,#62506,
#62507,#62508,#62509,#62510,#62511,#62512,#62513,#62514,#62515,#62516,#62517,
#62518,#62519,#62520,#62521,#62522,#62523,#62524,#62525,#62526,#62527,#62528,
#62529,#62530,#62531,#62532,#62533,#62534,#62535,#62536,#62537,#62538,#62539,
#62540,#62541,#62542,#62543,#62544,#62545,#62546,#62547,#62548,#62549,#62550,
#62551,#62552),.UNSPECIFIED.,.F.,.F.,(4,3,3,3,3,3,3,3,3,3,3,3,3,3,3,3,3,
3,3,3,3,3,3,3,3,3,3,3,3,3,3,3,3,3,3,3,3,3,3,3,3,3,3,3,3,3,3,3,3,3,3,3,3,
3,3,3,3,4),(19.9349334610966,19.9537583906529,20.0629283158291,20.1739930651237,
20.2828625555163,20.391665472945,20.5004418264274,20.6131929473669,20.722107125164,
20.8367767176748,20.9514463101855,21.0606162335135,21.1716809830391,21.280550471541,
21.3893533870683,21.4981297386421,21.6108808614111,21.7197950373033,21.8344646335107,
21.9491342297182,22.0583041526924,22.1693689022622,22.2782383903802,22.3870413055133,
22.4958176566833,22.6085687798252,22.7174829552942,22.8321525522725,22.9468221492508,
23.0559920728858,23.167056822373,23.2759263111791,23.3847292270085,23.4935055788819,
23.6062567013573,23.7151708775393,23.8298404731614,23.9445100687835,24.0536799921475,
24.1647447416686,24.2736142301963,24.3824171457456,24.4911934973373,24.603944620082,
24.7128587959821,24.8275283921491,24.9421979883161,25.0513679116608,25.1624326611843,
25.2713021496898,25.3801050652158,25.4888814167832,25.6016325395496,25.7105467154231,
25.8252163116359,25.9398859078487,26.0790023378198,26.2181187677909),
 .UNSPECIFIED.);
#728=B_SPLINE_CURVE_WITH_KNOTS('',3,(#62554,#62555,#62556,#62557,#62558,
#62559,#62560,#62561,#62562,#62563,#62564,#62565,#62566,#62567,#62568,#62569,
#62570,#62571,#62572,#62573,#62574,#62575,#62576,#62577,#62578,#62579,#62580,
#62581,#62582,#62583,#62584,#62585,#62586,#62587,#62588,#62589,#62590,#62591,
#62592,#62593,#62594,#62595,#62596,#62597,#62598,#62599,#62600,#62601,#62602,
#62603,#62604,#62605,#62606,#62607,#62608,#62609,#62610,#62611,#62612,#62613,
#62614,#62615,#62616,#62617,#62618,#62619,#62620,#62621,#62622,#62623,#62624,
#62625,#62626,#62627,#62628,#62629,#62630,#62631,#62632,#62633,#62634,#62635,
#62636,#62637,#62638,#62639,#62640,#62641,#62642,#62643,#62644,#62645,#62646,
#62647,#62648,#62649,#62650,#62651,#62652,#62653,#62654,#62655,#62656,#62657,
#62658,#62659,#62660,#62661,#62662,#62663,#62664,#62665,#62666,#62667,#62668,
#62669,#62670,#62671,#62672,#62673,#62674,#62675,#62676,#62677,#62678,#62679,
#62680,#62681,#62682,#62683,#62684,#62685,#62686,#62687,#62688,#62689,#62690,
#62691,#62692,#62693,#62694,#62695,#62696,#62697,#62698,#62699,#62700,#62701,
#62702,#62703,#62704,#62705,#62706,#62707,#62708,#62709,#62710,#62711,#62712,
#62713,#62714,#62715,#62716,#62717,#62718,#62719,#62720,#62721,#62722,#62723,
#62724,#62725,#62726,#62727,#62728),.UNSPECIFIED.,.F.,.F.,(4,3,3,3,3,3,
3,3,3,3,3,3,3,3,3,3,3,3,3,3,3,3,3,3,3,3,3,3,3,3,3,3,3,3,3,3,3,3,3,3,3,3,
3,3,3,3,3,3,3,3,3,3,3,3,3,3,3,3,4),(26.2181187682761,26.3260314065148,26.4338895648003,
26.5417345758493,26.6496837906648,26.7576875372505,26.8658900149683,26.9375738273814,
27.0467437507667,27.1578085002851,27.2666779888336,27.3754809044032,27.484257256015,
27.5970083787398,27.7059225546589,27.8205921507864,27.935261746914,28.0444316703009,
28.1554964198191,28.264365908369,28.3731688239399,28.4819451755529,28.5946962982764,
28.7036104741963,28.8182800703215,28.9329496664467,29.0421195898417,29.1531843393589,
29.2620538279173,29.3708567434968,29.4796330951187,29.5923842178338,29.7012983937628,
29.8159679898711,29.9306375859793,30.0398075093685,30.1508722588864,30.2597417474389,
30.3685446630125,30.4773210146281,30.5900721373491,30.6989863132719,30.8136559093919,
30.928325505512,31.0374954289073,31.1485601784245,31.2574296669829,31.3662325825624,
31.4750089341842,31.5877600568993,31.6966742328281,31.8113438289363,31.9260134250446,
32.037541760806,32.1534823394684,32.2646132694227,32.3756310959963,32.4865598326513,
32.5013040754557),.UNSPECIFIED.);
#729=B_SPLINE_CURVE_WITH_KNOTS('',3,(#62730,#62731,#62732,#62733,#62734,
#62735,#62736,#62737,#62738,#62739,#62740,#62741,#62742,#62743,#62744,#62745,
#62746,#62747,#62748,#62749,#62750,#62751,#62752,#62753,#62754,#62755,#62756,
#62757,#62758,#62759,#62760,#62761,#62762,#62763,#62764,#62765,#62766,#62767,
#62768,#62769,#62770,#62771,#62772,#62773,#62774,#62775,#62776,#62777,#62778,
#62779,#62780,#62781,#62782,#62783,#62784,#62785,#62786,#62787,#62788,#62789,
#62790,#62791,#62792,#62793,#62794,#62795,#62796,#62797,#62798,#62799,#62800,
#62801,#62802,#62803,#62804,#62805,#62806,#62807,#62808,#62809,#62810,#62811,
#62812,#62813,#62814,#62815,#62816,#62817,#62818,#62819,#62820,#62821,#62822,
#62823,#62824,#62825,#62826,#62827,#62828,#62829,#62830,#62831,#62832,#62833,
#62834,#62835,#62836,#62837,#62838,#62839,#62840,#62841,#62842,#62843,#62844,
#62845,#62846,#62847,#62848,#62849,#62850,#62851,#62852,#62853,#62854,#62855,
#62856,#62857,#62858,#62859,#62860,#62861,#62862,#62863,#62864,#62865,#62866,
#62867,#62868,#62869,#62870,#62871,#62872,#62873,#62874,#62875,#62876,#62877,
#62878,#62879,#62880,#62881,#62882,#62883,#62884,#62885,#62886,#62887,#62888,
#62889,#62890,#62891,#62892,#62893,#62894,#62895,#62896,#62897,#62898,#62899,
#62900,#62901),.UNSPECIFIED.,.F.,.F.,(4,3,3,3,3,3,3,3,3,3,3,3,3,3,3,3,3,
3,3,3,3,3,3,3,3,3,3,3,3,3,3,3,3,3,3,3,3,3,3,3,3,3,3,3,3,3,3,3,3,3,3,3,3,
3,3,3,3,4),(32.5013040758074,32.6198608438911,32.7387777837186,32.858217674201,
32.9237013445772,33.0328712679628,33.1439360174812,33.2528055060299,33.3616084215996,
33.4703847732114,33.583135895936,33.692050071855,33.8067196679824,33.9213892641099,
34.0305591875354,34.1416239370488,34.2504934256376,34.3592963412474,34.4680726928993,
34.5808238155851,34.6897379915434,34.804407587593,34.9190771836425,35.0282471069821,
35.1393118565063,35.2481813450097,35.3569842605347,35.4657606121023,35.5785117348705,
35.6874259107468,35.802095506961,35.9167651031752,36.025935026543,36.1369997760636,
36.2458692645929,36.3546721801429,36.4634485317346,36.5761996544779,36.6851138303758,
36.7997834265418,36.9144530227078,37.0236229463545,37.1346876958402,37.2435571846511,
37.3523601004828,37.461136452356,37.5738875748271,37.6828017510026,37.7974713466216,
37.9121409422405,38.021184497235,38.1286405836999,38.2359927120742,38.343283022873,
38.4535846127039,38.5609344442578,38.6727119132271,38.7844893821964),
 .UNSPECIFIED.);
#730=B_SPLINE_CURVE_WITH_KNOTS('',3,(#62903,#62904,#62905,#62906,#62907,
#62908,#62909,#62910,#62911,#62912,#62913,#62914,#62915,#62916,#62917,#62918,
#62919,#62920,#62921,#62922,#62923,#62924,#62925,#62926,#62927,#62928,#62929,
#62930,#62931,#62932,#62933,#62934,#62935,#62936,#62937,#62938,#62939,#62940,
#62941,#62942,#62943,#62944,#62945,#62946,#62947,#62948,#62949,#62950,#62951,
#62952,#62953,#62954,#62955,#62956,#62957,#62958,#62959,#62960,#62961,#62962,
#62963,#62964,#62965,#62966,#62967,#62968,#62969,#62970,#62971,#62972,#62973,
#62974,#62975,#62976,#62977,#62978,#62979,#62980,#62981,#62982,#62983,#62984,
#62985,#62986,#62987,#62988,#62989,#62990,#62991,#62992,#62993,#62994,#62995,
#62996,#62997,#62998,#62999,#63000,#63001,#63002,#63003,#63004,#63005,#63006,
#63007,#63008,#63009,#63010,#63011,#63012,#63013,#63014,#63015,#63016,#63017,
#63018,#63019,#63020,#63021,#63022,#63023,#63024,#63025,#63026,#63027,#63028,
#63029,#63030,#63031,#63032,#63033,#63034,#63035,#63036,#63037,#63038,#63039,
#63040,#63041,#63042,#63043,#63044,#63045,#63046,#63047,#63048,#63049,#63050,
#63051,#63052,#63053,#63054,#63055,#63056,#63057,#63058,#63059,#63060,#63061,
#63062,#63063,#63064,#63065,#63066,#63067,#63068,#63069,#63070,#63071),
 .UNSPECIFIED.,.F.,.F.,(4,3,3,3,3,3,3,3,3,3,3,3,3,3,3,3,3,3,3,3,3,3,3,3,
3,3,3,3,3,3,3,3,3,3,3,3,3,3,3,3,3,3,3,3,3,3,3,3,3,3,3,3,3,3,3,3,4),(38.7844893826353,
38.9098288617731,39.0189987851414,39.130063534662,39.2389330231807,39.3477359387159,
39.4565122902888,39.569263413043,39.6781775889125,39.7928471851092,39.9075167813058,
40.0166867065533,40.1277514558389,40.2366209462611,40.3454238637035,40.4542002171843,
40.5669513380978,40.6758655158546,40.7905351083465,40.9052047008384,41.0143746203194,
41.1254393703258,41.2343088549957,41.3431117667068,41.4518881144863,41.5646392409575,
41.6735534131527,41.7882230167618,41.902892620371,42.0120625448578,42.1231272942385,
42.2319967837874,42.3407997003176,42.4495760528488,42.5623271746126,42.6712413513396,
42.7859109456216,42.9005805399037,43.0097504763836,43.1208152242651,43.2296847260242,
43.338487654811,43.4472640196252,43.560015129578,43.6689293185101,43.7835988889732,
43.8982684594363,44.007438350286,44.1185031038713,44.2273725600332,44.3361754433597,
44.4449517629223,44.557702916934,44.6666170616515,44.7812867203103,44.895956378969,
45.0676746898149),.UNSPECIFIED.);
#731=B_SPLINE_CURVE_WITH_KNOTS('',3,(#63073,#63074,#63075,#63076,#63077,
#63078,#63079,#63080,#63081,#63082,#63083,#63084,#63085,#63086,#63087,#63088,
#63089,#63090,#63091,#63092,#63093,#63094,#63095,#63096,#63097,#63098,#63099,
#63100,#63101,#63102,#63103,#63104,#63105,#63106,#63107,#63108,#63109,#63110,
#63111,#63112,#63113,#63114,#63115,#63116,#63117,#63118,#63119,#63120,#63121,
#63122,#63123,#63124,#63125,#63126,#63127,#63128,#63129,#63130,#63131,#63132,
#63133,#63134,#63135,#63136,#63137,#63138,#63139,#63140,#63141,#63142,#63143,
#63144,#63145,#63146,#63147,#63148,#63149,#63150,#63151,#63152,#63153,#63154,
#63155,#63156,#63157,#63158,#63159,#63160,#63161,#63162,#63163,#63164,#63165,
#63166,#63167,#63168,#63169,#63170,#63171,#63172,#63173,#63174,#63175,#63176,
#63177,#63178,#63179,#63180,#63181,#63182,#63183,#63184,#63185,#63186,#63187,
#63188,#63189,#63190,#63191,#63192,#63193,#63194,#63195,#63196,#63197,#63198,
#63199,#63200,#63201,#63202,#63203,#63204,#63205,#63206,#63207,#63208,#63209,
#63210,#63211,#63212,#63213,#63214,#63215,#63216,#63217,#63218,#63219,#63220,
#63221,#63222,#63223,#63224,#63225,#63226,#63227,#63228,#63229,#63230,#63231,
#63232,#63233,#63234,#63235,#63236,#63237,#63238,#63239,#63240,#63241,#63242,
#63243,#63244),.UNSPECIFIED.,.F.,.F.,(4,3,3,3,3,3,3,3,3,3,3,3,3,3,3,3,3,
3,3,3,3,3,3,3,3,3,3,3,3,3,3,3,3,3,3,3,3,3,3,3,3,3,3,3,3,3,3,3,3,3,3,3,3,
3,3,3,3,4),(45.0676746901124,45.1750417725799,45.282302053759,45.3894977918574,
45.4966711412374,45.6039382377035,45.7112531460519,45.8187617443077,45.8936442985016,
46.002814310719,46.1138790491335,46.2227486276055,46.331551633255,46.4403280749561,
46.5530791107256,46.6619933757127,46.7766627968735,46.8913322180343,47.000501877111,
47.111566659668,47.2204358846347,47.3292385376104,47.4380146280312,47.5507660054152,
47.6596799266104,47.7743500320886,47.8890201375669,47.9981902797867,48.1092550019508,
48.2181247034541,48.3269278292316,48.4357043879899,48.5484553052673,48.6573696784251,
48.7720388677623,48.8867080570995,48.995878553069,49.1069432310144,49.2158133019497,
49.3246168019251,49.4333937389989,49.5461442984073,49.6550590555919,49.7697275161121,
49.8843959766322,49.9935638013074,50.1046288131645,50.2134962051043,50.322297030565,
50.4310713018833,50.5438244504537,50.6527365942569,50.7674102452109,50.8820838961648,
50.999277921294,51.1153231035882,51.2330915501348,51.3508599966814),
 .UNSPECIFIED.);
#732=B_SPLINE_CURVE_WITH_KNOTS('',3,(#63246,#63247,#63248,#63249,#63250,
#63251,#63252,#63253,#63254,#63255,#63256,#63257,#63258,#63259,#63260,#63261,
#63262,#63263,#63264,#63265,#63266,#63267,#63268,#63269,#63270,#63271,#63272,
#63273,#63274,#63275,#63276,#63277,#63278,#63279,#63280,#63281,#63282,#63283,
#63284,#63285,#63286,#63287,#63288,#63289,#63290,#63291,#63292,#63293,#63294,
#63295,#63296,#63297,#63298,#63299,#63300,#63301,#63302,#63303,#63304,#63305,
#63306,#63307,#63308,#63309,#63310,#63311,#63312,#63313,#63314,#63315,#63316,
#63317,#63318,#63319,#63320,#63321,#63322,#63323,#63324,#63325,#63326,#63327,
#63328,#63329,#63330,#63331,#63332,#63333,#63334,#63335,#63336,#63337,#63338,
#63339,#63340,#63341,#63342,#63343,#63344,#63345,#63346,#63347,#63348,#63349,
#63350,#63351,#63352,#63353,#63354,#63355,#63356,#63357,#63358,#63359,#63360,
#63361,#63362,#63363,#63364,#63365,#63366,#63367,#63368,#63369,#63370,#63371,
#63372,#63373,#63374,#63375,#63376,#63377,#63378,#63379,#63380,#63381,#63382,
#63383,#63384,#63385,#63386,#63387,#63388,#63389,#63390,#63391,#63392,#63393,
#63394,#63395,#63396,#63397,#63398,#63399,#63400,#63401,#63402,#63403,#63404,
#63405,#63406,#63407,#63408,#63409,#63410,#63411,#63412,#63413,#63414,#63415,
#63416,#63417,#63418,#63419,#63420),.UNSPECIFIED.,.F.,.F.,(4,3,3,3,3,3,
3,3,3,3,3,3,3,3,3,3,3,3,3,3,3,3,3,3,3,3,3,3,3,3,3,3,3,3,3,3,3,3,3,3,3,3,
3,3,3,3,3,3,3,3,3,3,3,3,3,3,3,3,4),(51.3508599969945,51.4634741467203,51.5763443922042,
51.6893483676939,51.8026435838821,51.8797718156975,51.988945155237,52.1000094777362,
52.2088824674154,52.3176889058393,52.4264687961371,52.5392165309103,52.6481342433072,
52.7627969892686,52.8774597352301,52.9866133635763,53.0976801499746,53.2065333314141,
53.3153199798818,53.4240801302457,53.536847011375,53.6457453351107,53.7604464949367,
53.8751476547628,53.9843392307382,54.0954012736828,54.2042921051629,54.3131161911514,
54.421913507944,54.5346440245319,54.6435784190957,54.7582069966955,54.8728355742954,
54.9820232591834,55.093085788514,55.2019737547881,55.3107953612392,55.4195905846614,
55.5323238119531,55.6412570841702,55.7558902889992,55.8705234938281,55.9795699161335,
56.0906501032869,56.199395785453,56.3080751149658,56.4167282948664,56.52959907449,
56.638392510654,56.747264113805,56.8563189544076,56.8682114133607,56.9761882052863,
57.0840128847663,57.1917273855887,57.3023068652351,57.4099598206258,57.5220025623999,
57.6340453041741),.UNSPECIFIED.);
#733=B_SPLINE_CURVE_WITH_KNOTS('',3,(#63422,#63423,#63424,#63425,#63426,
#63427,#63428,#63429,#63430,#63431,#63432,#63433,#63434,#63435,#63436,#63437,
#63438,#63439,#63440,#63441,#63442,#63443,#63444,#63445,#63446,#63447,#63448,
#63449,#63450,#63451,#63452,#63453,#63454,#63455,#63456,#63457,#63458),
 .UNSPECIFIED.,.F.,.F.,(4,3,3,3,3,3,3,3,3,3,3,3,4),(57.6340453045496,57.779619983922,
57.8658993328933,57.9751468990343,58.0862019432083,58.1951547315241,58.3040427964902,
58.4129059875357,58.5255763037583,58.6345804296199,58.7490838410229,58.863587252426,
58.8739410672733),.UNSPECIFIED.);
#734=B_SPLINE_CURVE_WITH_KNOTS('',3,(#63462,#63463,#63464,#63465,#63466,
#63467,#63468),.UNSPECIFIED.,.F.,.F.,(4,3,4),(-60.8589630914912,-60.7203125906016,
-60.5899052282396),.UNSPECIFIED.);
#735=B_SPLINE_CURVE_WITH_KNOTS('',3,(#63470,#63471,#63472,#63473,#63474,
#63475,#63476,#63477,#63478,#63479),.UNSPECIFIED.,.F.,.F.,(4,1,1,1,1,1,
1,4),(-60.5899049028663,-59.8612751719586,-58.863587252426,-57.8658993328933,
-56.8682114133607,-55.8705234938281,-54.8728355742954,-54.3067195956867),
 .UNSPECIFIED.);
#736=B_SPLINE_CURVE_WITH_KNOTS('',3,(#63481,#63482,#63483,#63484,#63485,
#63486,#63487,#63488,#63489,#63490,#63491,#63492,#63493,#63494,#63495,#63496,
#63497,#63498,#63499,#63500,#63501,#63502,#63503,#63504,#63505,#63506,#63507,
#63508,#63509,#63510,#63511,#63512,#63513,#63514,#63515,#63516,#63517,#63518,
#63519,#63520,#63521,#63522,#63523,#63524,#63525,#63526,#63527,#63528,#63529,
#63530,#63531,#63532,#63533,#63534,#63535,#63536,#63537,#63538,#63539,#63540,
#63541,#63542,#63543,#63544,#63545,#63546,#63547,#63548,#63549,#63550,#63551,
#63552,#63553,#63554,#63555,#63556,#63557,#63558,#63559,#63560,#63561,#63562,
#63563,#63564,#63565,#63566,#63567,#63568,#63569,#63570,#63571,#63572,#63573,
#63574,#63575,#63576,#63577,#63578,#63579,#63580,#63581,#63582,#63583,#63584,
#63585,#63586,#63587,#63588,#63589,#63590,#63591,#63592,#63593,#63594,#63595,
#63596,#63597,#63598,#63599,#63600,#63601,#63602,#63603,#63604,#63605,#63606,
#63607,#63608,#63609,#63610,#63611,#63612,#63613,#63614,#63615,#63616,#63617,
#63618,#63619,#63620,#63621,#63622,#63623,#63624,#63625,#63626,#63627,#63628,
#63629,#63630,#63631,#63632,#63633,#63634,#63635,#63636,#63637,#63638,#63639,
#63640,#63641,#63642,#63643,#63644,#63645,#63646,#63647,#63648,#63649,#63650,
#63651,#63652),.UNSPECIFIED.,.F.,.F.,(4,3,3,3,3,3,3,3,3,3,3,3,3,3,3,3,3,
3,3,3,3,3,3,3,3,3,3,3,3,3,3,3,3,3,3,3,3,3,3,3,3,3,3,3,3,3,3,3,3,3,3,3,3,
3,3,3,3,4),(-54.3067192612381,-54.1887395011815,-54.0704302450224,-53.9516185764346,
-53.8751476547628,-53.7659931173469,-53.6549264445823,-53.5460728899735,
-53.437286068191,-53.3285259440385,-53.2157593918364,-53.1068615894403,
-52.9921606623352,-52.8774597352301,-52.7682863165904,-52.6572220039788,
-52.5483489798132,-52.4395425235527,-52.3307626320459,-52.2180149279588,
-52.1090972556454,-51.9944345356715,-51.8797718156975,-51.7705999034038,
-51.6595354024989,-51.5506638080811,-51.4418587488731,-51.3330802192985,
-51.2203311385151,-51.1114147238957,-50.9967493100302,-50.8820838961648,
-50.772915942593,-50.6618509468479,-50.5529835021134,-50.4441826522408,
-50.3354083848465,-50.222655282793,-50.1137432132176,-49.9990695949249,
-49.8843959766322,-49.7752254818367,-49.6641608037445,-49.5552907329995,
-49.4464872328491,-49.3377102952362,-49.224959735702,-49.1160449770806,
-49.0013765170901,-48.8867080570995,-48.7788113360781,-48.6713935084339,
-48.5640801570707,-48.4568290977937,-48.3485053955774,-48.2411984952054,
-48.1323663920669,-48.0235342889285),.UNSPECIFIED.);
#737=B_SPLINE_CURVE_WITH_KNOTS('',3,(#63654,#63655,#63656,#63657,#63658,
#63659,#63660,#63661,#63662,#63663,#63664,#63665,#63666,#63667,#63668,#63669,
#63670,#63671,#63672,#63673,#63674,#63675,#63676,#63677,#63678,#63679,#63680,
#63681,#63682,#63683,#63684,#63685,#63686,#63687,#63688,#63689,#63690,#63691,
#63692,#63693,#63694,#63695,#63696,#63697,#63698,#63699,#63700,#63701,#63702,
#63703,#63704,#63705,#63706,#63707,#63708,#63709,#63710,#63711,#63712,#63713,
#63714,#63715,#63716,#63717,#63718,#63719,#63720,#63721,#63722,#63723,#63724,
#63725,#63726,#63727,#63728,#63729,#63730,#63731,#63732,#63733,#63734,#63735,
#63736,#63737,#63738,#63739,#63740,#63741,#63742,#63743,#63744,#63745,#63746,
#63747,#63748,#63749,#63750,#63751,#63752,#63753,#63754,#63755,#63756,#63757,
#63758,#63759,#63760,#63761,#63762,#63763,#63764,#63765,#63766,#63767,#63768,
#63769,#63770,#63771,#63772,#63773,#63774,#63775,#63776,#63777,#63778,#63779,
#63780,#63781,#63782,#63783,#63784,#63785,#63786,#63787,#63788,#63789,#63790,
#63791,#63792,#63793,#63794,#63795,#63796,#63797,#63798,#63799,#63800,#63801,
#63802,#63803,#63804,#63805,#63806,#63807,#63808,#63809,#63810,#63811,#63812,
#63813,#63814,#63815,#63816,#63817,#63818,#63819,#63820,#63821,#63822),
 .UNSPECIFIED.,.F.,.F.,(4,3,3,3,3,3,3,3,3,3,3,3,3,3,3,3,3,3,3,3,3,3,3,3,
3,3,3,3,3,3,3,3,3,3,3,3,3,3,3,3,3,3,3,3,3,3,3,3,3,3,3,3,3,3,3,3,4),(-48.0235342885071,
-47.8890201375669,-47.7798504607805,-47.6687856804372,-47.5599164482297,
-47.4511137919178,-47.3423377020588,-47.2295863310527,-47.12067242009,-47.0060023190621,
-46.8913322180343,-46.7821622073899,-46.6710974687789,-46.5622278909087,
-46.453424885499,-46.3446484436765,-46.2318974073827,-46.1229831413787,
-46.0083137199401,-45.8936442985016,-45.7844743602938,-45.6734096126282,
-45.5645401079166,-45.4557371757283,-45.3469608070684,-45.2342097000436,
-45.1252955061971,-45.0106259425831,-44.895956378969,-44.7867864857488,
-44.6757217324597,-44.56685227533,-44.4580493915589,-44.3492730720737,-44.2365219189143,
-44.1276077755701,-44.0129381175032,-43.8982684594363,-43.789098523333,
-43.6780337754043,-43.5691642737932,-43.460361345069,-43.3515849802323,
-43.2388338701502,-43.1299196809845,-43.0152501104441,-42.9005805399037,
-42.7914106158111,-42.6803458663811,-42.571476376996,-42.4626734605437,
-42.3538971080047,-42.2411459860962,-42.1322318091485,-42.0175622147598,
-41.902892620371,-41.7403489813275),.UNSPECIFIED.);
#738=B_SPLINE_CURVE_WITH_KNOTS('',3,(#63824,#63825,#63826,#63827,#63828,
#63829,#63830,#63831,#63832,#63833,#63834,#63835,#63836,#63837,#63838,#63839,
#63840,#63841,#63842,#63843,#63844,#63845,#63846,#63847,#63848,#63849,#63850,
#63851,#63852,#63853,#63854,#63855,#63856,#63857,#63858,#63859,#63860,#63861,
#63862,#63863,#63864,#63865,#63866,#63867,#63868,#63869,#63870,#63871,#63872,
#63873,#63874,#63875,#63876,#63877,#63878,#63879,#63880,#63881,#63882,#63883,
#63884,#63885,#63886,#63887,#63888,#63889,#63890,#63891,#63892,#63893,#63894,
#63895,#63896,#63897,#63898,#63899,#63900,#63901,#63902,#63903,#63904,#63905,
#63906,#63907,#63908,#63909,#63910,#63911,#63912,#63913,#63914,#63915,#63916,
#63917,#63918,#63919,#63920,#63921,#63922,#63923,#63924,#63925,#63926,#63927,
#63928,#63929,#63930,#63931,#63932,#63933,#63934,#63935,#63936,#63937,#63938,
#63939,#63940,#63941,#63942,#63943,#63944,#63945,#63946,#63947,#63948,#63949,
#63950,#63951,#63952,#63953,#63954,#63955,#63956,#63957,#63958,#63959,#63960,
#63961,#63962,#63963,#63964,#63965,#63966,#63967,#63968,#63969,#63970,#63971,
#63972,#63973,#63974,#63975,#63976,#63977,#63978,#63979,#63980,#63981,#63982,
#63983,#63984,#63985,#63986,#63987,#63988,#63989,#63990,#63991,#63992,#63993,
#63994,#63995),.UNSPECIFIED.,.F.,.F.,(4,3,3,3,3,3,3,3,3,3,3,3,3,3,3,3,3,
3,3,3,3,3,3,3,3,3,3,3,3,3,3,3,3,3,3,3,3,3,3,3,3,3,3,3,3,3,3,3,3,3,3,3,3,
3,3,3,3,4),(-41.7403489809942,-41.6329694234406,-41.5257002609243,-41.4184992250767,
-41.3113241566121,-41.204057916278,-41.0967470791135,-40.9892397008504,
-40.9052047008384,-40.7960347756599,-40.6849700263657,-40.5761005359707,
-40.4672976185397,-40.3585212650549,-40.2457701441176,-40.1368559663182,
-40.0221863738119,-39.9075167813057,-39.798346857978,-39.6872821084524,
-39.5784126199507,-39.4696097044238,-39.3608333528504,-39.2480822300811,
-39.1391680541892,-39.0244984579812,-38.9098288617731,-38.8006589387994,
-38.6895941892295,-38.580724701112,-38.4719217859793,-38.3631454348099,
-38.2503943116676,-38.1414801361991,-38.0268105392198,-37.9121409422405,
-37.8029710186051,-37.691906269118,-37.5830367803116,-37.4742338644818,
-37.3654575126082,-37.2527063901331,-37.1437922139506,-37.0291226183292,
-36.9144530227078,-36.8052830993439,-36.6942183498228,-36.5853488612952,
-36.4765459457459,-36.3677695941543,-36.2550184714095,-36.1461042955095,
-36.0314346993424,-35.9167651031752,-35.7999067404385,-35.6833251833026,
-35.5671586433901,-35.4571636745501),.UNSPECIFIED.);
#739=B_SPLINE_CURVE_WITH_KNOTS('',3,(#63997,#63998,#63999,#64000,#64001,
#64002,#64003,#64004,#64005,#64006,#64007,#64008,#64009,#64010,#64011,#64012,
#64013,#64014,#64015,#64016,#64017,#64018,#64019,#64020,#64021,#64022,#64023,
#64024,#64025,#64026,#64027,#64028,#64029,#64030,#64031,#64032,#64033,#64034,
#64035,#64036,#64037,#64038,#64039,#64040,#64041,#64042,#64043,#64044,#64045,
#64046,#64047,#64048,#64049,#64050,#64051,#64052,#64053,#64054,#64055,#64056,
#64057,#64058,#64059,#64060,#64061,#64062,#64063,#64064,#64065,#64066,#64067,
#64068,#64069,#64070,#64071,#64072,#64073,#64074,#64075,#64076,#64077,#64078,
#64079,#64080,#64081,#64082,#64083,#64084,#64085,#64086,#64087,#64088,#64089,
#64090,#64091,#64092,#64093,#64094,#64095,#64096,#64097,#64098,#64099,#64100,
#64101,#64102,#64103,#64104,#64105,#64106,#64107,#64108,#64109,#64110,#64111,
#64112,#64113,#64114,#64115,#64116,#64117,#64118,#64119,#64120,#64121,#64122,
#64123,#64124,#64125,#64126,#64127,#64128,#64129,#64130,#64131,#64132,#64133,
#64134,#64135,#64136,#64137,#64138,#64139,#64140,#64141,#64142,#64143,#64144,
#64145,#64146,#64147,#64148,#64149,#64150,#64151,#64152,#64153,#64154,#64155,
#64156,#64157,#64158,#64159,#64160,#64161,#64162,#64163,#64164,#64165,#64166,
#64167,#64168),.UNSPECIFIED.,.F.,.F.,(4,3,3,3,3,3,3,3,3,3,3,3,3,3,3,3,3,
3,3,3,3,3,3,3,3,3,3,3,3,3,3,3,3,3,3,3,3,3,3,3,3,3,3,3,3,3,3,3,3,3,3,3,3,
3,3,3,3,4),(-35.4571636741479,-35.344912853165,-35.2324236048642,-35.1198119929548,
-35.0069133599008,-34.9190771836425,-34.8099072602187,-34.6988425107051,
-34.5899730221171,-34.4811701065077,-34.3723937548559,-34.2596426321694,
-34.1507284562101,-34.03605886016,-33.9213892641099,-33.8122193407245,-33.7011545912061,
-33.5922851026576,-33.4834821870879,-33.374705835476,-33.2619547127513,
-33.1530405368323,-33.0383709407047,-32.9237013445772,-32.8145314211901,
-32.7034666716719,-32.5945971831221,-32.4857942675512,-32.3770179159381,
-32.2642667932148,-32.1553526172948,-32.0406830211697,-31.9260134250446,
-31.8168435016496,-31.7057787521324,-31.5969092635741,-31.4881063479944,
-31.3793299963728,-31.2665788736576,-31.1576646977287,-31.0429951016203,
-30.9283255055119,-30.8191555821226,-30.7080908326047,-30.5992213440521,
-30.4904184284786,-30.3816420768629,-30.268890954142,-30.1599767782191,
-30.0453071820992,-29.9306375859793,-29.8228320190155,-29.7151785918317,
-29.6076351924948,-29.4992209861132,-29.3917393866121,-29.2828588767902,
-29.1739783669683),.UNSPECIFIED.);
#740=B_SPLINE_CURVE_WITH_KNOTS('',3,(#64170,#64171,#64172,#64173,#64174,
#64175,#64176,#64177,#64178,#64179,#64180,#64181,#64182,#64183,#64184,#64185,
#64186,#64187,#64188,#64189,#64190,#64191,#64192,#64193,#64194,#64195,#64196,
#64197,#64198,#64199,#64200,#64201,#64202,#64203,#64204,#64205,#64206,#64207,
#64208,#64209,#64210,#64211,#64212,#64213,#64214,#64215,#64216,#64217,#64218,
#64219,#64220,#64221,#64222,#64223,#64224,#64225,#64226,#64227,#64228,#64229,
#64230,#64231,#64232,#64233,#64234,#64235,#64236,#64237,#64238,#64239,#64240,
#64241,#64242,#64243,#64244,#64245,#64246,#64247,#64248,#64249,#64250,#64251,
#64252,#64253,#64254,#64255,#64256,#64257,#64258,#64259,#64260,#64261,#64262,
#64263,#64264,#64265,#64266,#64267,#64268,#64269,#64270,#64271,#64272,#64273,
#64274,#64275,#64276,#64277,#64278,#64279,#64280,#64281,#64282,#64283,#64284,
#64285,#64286,#64287,#64288,#64289,#64290,#64291,#64292,#64293,#64294,#64295,
#64296,#64297,#64298,#64299,#64300,#64301,#64302,#64303,#64304,#64305,#64306,
#64307,#64308,#64309,#64310,#64311,#64312,#64313,#64314,#64315,#64316,#64317,
#64318,#64319,#64320,#64321,#64322,#64323,#64324,#64325,#64326,#64327,#64328,
#64329,#64330,#64331,#64332,#64333,#64334,#64335,#64336,#64337,#64338,#64339,
#64340,#64341),.UNSPECIFIED.,.F.,.F.,(4,3,3,3,3,3,3,3,3,3,3,3,3,3,3,3,3,
3,3,3,3,3,3,3,3,3,3,3,3,3,3,3,3,3,3,3,3,3,3,3,3,3,3,3,3,3,3,3,3,3,3,3,3,
3,3,3,3,4),(-29.1739783666309,-29.0306086412345,-28.9329496664467,-28.8237797430603,
-28.712714993542,-28.6038455049923,-28.4950425894213,-28.3862662378082,
-28.2735151150846,-28.1646009391642,-28.0499313430391,-27.935261746914,
-27.8260918235285,-27.7150270740101,-27.6061575854616,-27.497354669892,
-27.3885783182803,-27.2758271955556,-27.1669130196368,-27.0522434235091,
-26.9375738273814,-26.8284039039558,-26.7173391544424,-26.6084696658535,
-26.4996667502436,-26.3908903985916,-26.2781392759059,-26.1692250999475,
-26.0545555038981,-25.9398859078487,-25.8307159845091,-25.719651234985,
-25.6107817464816,-25.5019788309567,-25.3932024793892,-25.2804513566209,
-25.1715371807446,-25.0568675845304,-24.9421979883161,-24.8330280649484,
-24.7219633154277,-24.6130938268984,-24.5042909113485,-24.3955145597569,
-24.2827634370135,-24.1738492611156,-24.0591796649495,-23.9445100687834,
-23.8353401451363,-23.7242753956507,-23.6154059068394,-23.5066029910073,
-23.3978266391338,-23.2850755166631,-23.1761613404872,-23.061491744869,
-22.9468221492508,-22.8907930597887),.UNSPECIFIED.);
#741=B_SPLINE_CURVE_WITH_KNOTS('',3,(#64343,#64344,#64345,#64346,#64347,
#64348,#64349,#64350,#64351,#64352,#64353,#64354,#64355,#64356,#64357,#64358,
#64359,#64360,#64361,#64362,#64363,#64364,#64365,#64366,#64367,#64368,#64369,
#64370,#64371,#64372,#64373,#64374,#64375,#64376,#64377,#64378,#64379,#64380,
#64381,#64382,#64383,#64384,#64385,#64386,#64387,#64388,#64389,#64390,#64391,
#64392,#64393,#64394,#64395,#64396,#64397,#64398,#64399,#64400,#64401,#64402,
#64403,#64404,#64405,#64406,#64407,#64408,#64409,#64410,#64411,#64412,#64413,
#64414,#64415,#64416,#64417,#64418,#64419,#64420,#64421,#64422,#64423,#64424,
#64425,#64426,#64427,#64428,#64429,#64430,#64431,#64432,#64433,#64434,#64435,
#64436,#64437,#64438,#64439,#64440,#64441,#64442,#64443,#64444,#64445,#64446,
#64447,#64448,#64449,#64450,#64451,#64452,#64453,#64454,#64455,#64456,#64457,
#64458,#64459,#64460,#64461,#64462,#64463,#64464,#64465,#64466,#64467,#64468,
#64469,#64470,#64471,#64472,#64473,#64474,#64475,#64476,#64477,#64478,#64479,
#64480,#64481,#64482,#64483,#64484,#64485,#64486,#64487,#64488,#64489,#64490,
#64491,#64492,#64493,#64494,#64495,#64496,#64497,#64498,#64499,#64500,#64501,
#64502,#64503,#64504,#64505,#64506,#64507,#64508,#64509,#64510,#64511,#64512,
#64513,#64514),.UNSPECIFIED.,.F.,.F.,(4,3,3,3,3,3,3,3,3,3,3,3,3,3,3,3,3,
3,3,3,3,3,3,3,3,3,3,3,3,3,3,3,3,3,3,3,3,3,3,3,3,3,3,3,3,3,3,3,3,3,3,3,3,
3,3,3,3,4),(-22.8907930594412,-22.7825589193295,-22.6745058528515,-22.5665527900898,
-22.4586583131073,-22.3507810903025,-22.2428041434464,-22.1347762876769,
-22.026550528337,-21.9491342297182,-21.8399643063501,-21.7288995568295,
-21.620030068311,-21.511227152776,-21.4024508012033,-21.2896996784488,-21.1807855025796,
-21.0661159063825,-20.9514463101855,-20.8422763849356,-20.7312116356503,
-20.6223421452257,-20.5135392277807,-20.4047628742975,-20.2920117533864,
-20.1830975756272,-20.0684279831401,-19.9537583906529,-19.8445884711759,
-19.733523721169,-19.624654236503,-19.5158513247957,-19.40707497702,-19.2943238505451,
-19.1854096783537,-19.0707400747369,-18.9560704711202,-18.8469005466336,
-18.7358357972529,-18.6269663077043,-18.5181633911742,-18.4093870386433,
-18.2966359168794,-18.1877217401528,-18.0730521458702,-17.9583825515876,
-17.8492126150935,-17.7381478672137,-17.6292783654402,-17.520475436639,
-17.4116990718104,-17.2989479618716,-17.1900337729252,-17.0753642024901,
-16.9606946320549,-16.8349352911367,-16.7102672428761,-16.6076077530603),
 .UNSPECIFIED.);
#742=B_SPLINE_CURVE_WITH_KNOTS('',3,(#64516,#64517,#64518,#64519,#64520,
#64521,#64522,#64523,#64524,#64525,#64526,#64527,#64528,#64529,#64530,#64531,
#64532,#64533,#64534,#64535,#64536,#64537,#64538,#64539,#64540,#64541,#64542,
#64543,#64544,#64545,#64546,#64547,#64548,#64549,#64550,#64551,#64552,#64553,
#64554,#64555,#64556,#64557,#64558,#64559,#64560,#64561,#64562,#64563,#64564,
#64565,#64566,#64567,#64568,#64569,#64570,#64571,#64572,#64573,#64574,#64575,
#64576,#64577,#64578,#64579,#64580,#64581,#64582,#64583,#64584,#64585,#64586,
#64587,#64588,#64589,#64590,#64591,#64592,#64593,#64594,#64595,#64596,#64597,
#64598,#64599,#64600,#64601,#64602,#64603,#64604,#64605,#64606,#64607,#64608,
#64609,#64610,#64611,#64612,#64613,#64614,#64615,#64616,#64617,#64618,#64619,
#64620,#64621,#64622,#64623,#64624,#64625,#64626,#64627,#64628,#64629,#64630,
#64631,#64632,#64633,#64634,#64635,#64636,#64637,#64638,#64639,#64640,#64641,
#64642,#64643,#64644,#64645,#64646,#64647,#64648,#64649,#64650,#64651,#64652,
#64653,#64654,#64655,#64656,#64657,#64658,#64659,#64660,#64661,#64662,#64663,
#64664,#64665,#64666,#64667,#64668,#64669,#64670,#64671,#64672,#64673,#64674,
#64675,#64676,#64677,#64678,#64679,#64680,#64681,#64682,#64683,#64684,#64685,
#64686,#64687),.UNSPECIFIED.,.F.,.F.,(4,3,3,3,3,3,3,3,3,3,3,3,3,3,3,3,3,
3,3,3,3,3,3,3,3,3,3,3,3,3,3,3,3,3,3,3,3,3,3,3,3,3,3,3,3,3,3,3,3,3,3,3,3,
3,3,3,3,4),(-16.6076077526092,-16.4984911608107,-16.3893763320133,-16.2801378311394,
-16.1708390750773,-16.0613160672559,-15.9630067125223,-15.8538367706882,
-15.7427720234759,-15.6339025172588,-15.5250995843561,-15.4163232157718,
-15.3035721100763,-15.1946579182654,-15.0799883556275,-14.9653187929897,
-14.8561487806862,-14.7450840422826,-14.6362144637235,-14.5274114579869,
-14.4186350161989,-14.3058839805135,-14.1969697154406,-14.0823002944488,
-13.967630873457,-13.8584612145722,-13.7473964319912,-13.6385272072156,
-13.5297245544302,-13.4209484641989,-13.3081970866303,-13.1992831656195,
-13.084613059772,-12.9699429539244,-12.8607728116244,-12.7497080894703,
-12.6408383878908,-12.5320352620388,-12.4232587032078,-12.3105077860037,
-12.2015934127785,-12.0869242235851,-11.9722550343917,-11.8630845379244,
-11.7520198600413,-11.6431497886023,-11.5343462881227,-11.4255693505448,
-11.3128187916234,-11.2039040339403,-11.0892355743997,-10.9745671148591,
-10.8651519782074,-10.7559060984897,-10.6467953979075,-10.5377672062601,
-10.428744585677,-10.3244224454296),.UNSPECIFIED.);
#743=B_SPLINE_CURVE_WITH_KNOTS('',3,(#64688,#64689,#64690,#64691,#64692,
#64693,#64694,#64695,#64696,#64697,#64698,#64699,#64700,#64701,#64702,#64703,
#64704,#64705,#64706,#64707,#64708,#64709,#64710,#64711,#64712,#64713,#64714,
#64715,#64716,#64717,#64718,#64719,#64720,#64721,#64722,#64723,#64724,#64725,
#64726,#64727,#64728,#64729,#64730,#64731,#64732,#64733,#64734,#64735,#64736,
#64737,#64738,#64739,#64740,#64741,#64742,#64743,#64744,#64745,#64746,#64747,
#64748,#64749,#64750,#64751,#64752,#64753,#64754,#64755,#64756,#64757,#64758,
#64759,#64760,#64761,#64762,#64763,#64764,#64765,#64766,#64767,#64768,#64769,
#64770,#64771,#64772,#64773,#64774,#64775,#64776,#64777,#64778,#64779,#64780,
#64781,#64782,#64783,#64784,#64785,#64786,#64787,#64788,#64789,#64790,#64791,
#64792,#64793,#64794,#64795,#64796,#64797,#64798,#64799,#64800,#64801,#64802,
#64803,#64804,#64805,#64806,#64807,#64808,#64809,#64810,#64811,#64812,#64813,
#64814,#64815,#64816,#64817,#64818,#64819,#64820,#64821,#64822,#64823,#64824,
#64825,#64826,#64827,#64828,#64829,#64830,#64831,#64832,#64833,#64834,#64835,
#64836,#64837,#64838,#64839,#64840,#64841,#64842,#64843,#64844,#64845,#64846,
#64847,#64848,#64849,#64850,#64851,#64852,#64853,#64854,#64855,#64856,#64857,
#64858,#64859),.UNSPECIFIED.,.F.,.F.,(4,3,3,3,3,3,3,3,3,3,3,3,3,3,3,3,3,
3,3,3,3,3,3,3,3,3,3,3,3,3,3,3,3,3,3,3,3,3,3,3,3,3,3,3,3,3,3,3,3,3,3,3,3,
3,3,3,3,4),(-10.3244224449824,-10.1993916813248,-10.0731708785139,-9.97687919532644,
-9.86770700904284,-9.75664254238671,-9.64777083422229,-9.5389657210407,
-9.43018719717089,-9.31743821682662,-9.20852195600055,-9.09385661589717,
-8.9791912757938,-8.87001793349893,-8.7589536113442,-8.65008061887294,-8.54127417765129,
-8.43249428455432,-8.31974655248103,-8.21082883731402,-8.09616609678758,
-7.98150335626115,-7.87234973519855,-7.76128294788979,-7.65242977373111,
-7.54364313252348,-7.4348829893877,-7.3221161012229,-7.21321778455413,-7.09851661064132,
-6.98381543672851,-6.87462385635979,-6.7635618139643,-6.65467097820688,
-6.54584688799528,-6.43704956703977,-6.32431905457879,-6.21538465604731,
-6.10075608662159,-5.98612751719586,-5.87693981736238,-5.76587728989998,
-5.65698930848159,-5.5481676868544,-5.43937244824885,-5.32663923560244,
-5.21770594836024,-5.10307277301173,-4.98843959766322,-4.88022583904749,
-4.77220199698845,-4.66428364169945,-4.55642929382362,-4.44859756765392,
-4.34067235294103,-4.23270085154882,-4.12453357256264,-4.04123713858576),
 .UNSPECIFIED.);
#744=B_SPLINE_CURVE_WITH_KNOTS('',3,(#64862,#64863,#64864,#64865,#64866,
#64867,#64868,#64869,#64870,#64871,#64872,#64873,#64874,#64875,#64876,#64877,
#64878,#64879,#64880,#64881,#64882,#64883,#64884,#64885,#64886),
 .UNSPECIFIED.,.F.,.F.,(4,3,3,3,3,3,3,3,4),(65.1150562521972,65.2322256069618,
65.3494523200733,65.4669033672003,65.5418737844617,65.669718746099,65.7971813969394,
65.9240711597633,65.9734457248706),.UNSPECIFIED.);
#745=B_SPLINE_CURVE_WITH_KNOTS('',3,(#64888,#64889,#64890,#64891,#64892,
#64893,#64894,#64895,#64896,#64897,#64898,#64899,#64900,#64901,#64902,#64903,
#64904,#64905,#64906,#64907,#64908,#64909,#64910,#64911,#64912,#64913,#64914,
#64915,#64916,#64917,#64918,#64919,#64920,#64921,#64922,#64923,#64924,#64925,
#64926,#64927,#64928,#64929,#64930,#64931,#64932,#64933,#64934,#64935,#64936,
#64937,#64938,#64939,#64940,#64941,#64942,#64943,#64944,#64945,#64946,#64947,
#64948,#64949,#64950,#64951,#64952,#64953,#64954,#64955,#64956,#64957,#64958,
#64959,#64960,#64961,#64962,#64963,#64964,#64965,#64966,#64967,#64968,#64969,
#64970,#64971,#64972,#64973,#64974,#64975,#64976,#64977,#64978,#64979,#64980,
#64981,#64982,#64983,#64984,#64985,#64986,#64987,#64988,#64989,#64990,#64991,
#64992,#64993,#64994,#64995,#64996,#64997,#64998,#64999,#65000,#65001,#65002,
#65003,#65004,#65005,#65006,#65007,#65008,#65009,#65010,#65011,#65012,#65013,
#65014),.UNSPECIFIED.,.F.,.F.,(4,3,3,3,3,3,3,3,3,3,3,3,3,3,3,3,3,3,3,3,
3,3,3,3,3,3,3,3,3,3,3,3,3,3,3,3,3,3,3,3,3,3,4),(65.9734457253856,66.0931803203325,
66.2131255046649,66.3331795104007,66.453526391453,66.5395617039943,66.6570817211347,
66.7743859463503,66.8915713205084,67.0086877877879,67.1257851800162,67.2429971337764,
67.3602722427648,67.4777663961338,67.537249623527,67.6546175408908,67.7717689826245,
67.8888012744095,68.0057646433112,68.1227092034736,68.239769929466,68.356894496607,
68.4742409440685,68.5349375430596,68.65265075336,68.7701461217343,68.8875212053768,
69.0048256039178,69.1221088027688,69.2395019098775,69.3569557779961,69.4746229182873,
69.5326254625923,69.650210022574,69.7675822346185,69.8848376574316,70.0020260737922,
70.1191971568852,70.2364847930213,70.3538368252063,70.4714088735417,70.5303133821249,
70.5406671969722),.UNSPECIFIED.);
#746=B_SPLINE_CURVE_WITH_KNOTS('',3,(#65018,#65019,#65020,#65021,#65022,
#65023,#65024,#65025,#65026,#65027,#65028,#65029,#65030,#65031,#65032,#65033,
#65034,#65035,#65036,#65037,#65038,#65039,#65040,#65041,#65042,#65043,#65044,
#65045,#65046,#65047,#65048,#65049,#65050,#65051,#65052,#65053,#65054,#65055,
#65056,#65057,#65058,#65059,#65060,#65061,#65062,#65063,#65064,#65065,#65066,
#65067,#65068,#65069,#65070,#65071,#65072,#65073,#65074,#65075,#65076,#65077,
#65078,#65079,#65080,#65081,#65082,#65083,#65084,#65085,#65086,#65087,#65088,
#65089,#65090,#65091,#65092,#65093,#65094,#65095,#65096,#65097,#65098,#65099,
#65100,#65101,#65102,#65103,#65104,#65105),.UNSPECIFIED.,.F.,.F.,(4,3,3,
3,3,3,3,3,3,3,3,3,3,3,3,3,3,3,3,3,3,3,3,3,3,3,3,3,3,4),(65.9734457260144,
66.1301294810741,66.2052997541048,66.3228842060623,66.4402563097625,66.5575116241308,
66.6746999321573,66.7918709072384,66.9091584367217,67.0265103628761,67.1440823074026,
67.2029876736375,67.3193780628697,67.4355547744305,67.5516145993876,67.6676093259448,
67.7835906279157,67.8997035752663,68.0158874444454,68.1323155233877,68.2006755931701,
68.3253865831117,68.4457795259765,68.5660152672273,68.6861349469942,68.8061795199567,
68.9262260304059,69.0462720762451,69.1664064774643,69.1983635127028),
 .UNSPECIFIED.);
#747=B_SPLINE_CURVE_WITH_KNOTS('',3,(#65106,#65107,#65108,#65109,#65110,
#65111,#65112,#65113,#65114,#65115,#65116,#65117,#65118,#65119,#65120,#65121,
#65122,#65123,#65124,#65125,#65126,#65127,#65128,#65129,#65130,#65131),
 .UNSPECIFIED.,.F.,.F.,(4,2,2,2,2,2,2,2,2,2,2,2,4),(-1.60477775251229,-1.58384253663988,
-1.57768502680862,-1.57259023840276,-1.56713336014366,-1.55999142624319,
-1.53082582288673,-1.51900551052497,-1.51135046950296,-1.50770451735264,
-1.5045888071128,-1.49970347412066,-1.49514144568264),.UNSPECIFIED.);
#748=B_SPLINE_CURVE_WITH_KNOTS('',3,(#65136,#65137,#65138,#65139,#65140,
#65141,#65142,#65143,#65144,#65145,#65146,#65147,#65148,#65149,#65150,#65151,
#65152,#65153,#65154,#65155,#65156,#65157,#65158,#65159,#65160,#65161,#65162,
#65163,#65164,#65165,#65166,#65167,#65168,#65169,#65170,#65171,#65172,#65173,
#65174,#65175,#65176,#65177,#65178,#65179,#65180,#65181,#65182,#65183,#65184,
#65185,#65186,#65187,#65188,#65189,#65190,#65191,#65192,#65193,#65194,#65195,
#65196,#65197,#65198,#65199,#65200,#65201,#65202,#65203,#65204,#65205,#65206,
#65207,#65208,#65209,#65210,#65211),.UNSPECIFIED.,.F.,.F.,(4,3,3,3,3,3,
3,3,3,3,3,3,3,3,3,3,3,3,3,3,3,3,3,3,3,4),(-0.295806539842427,-0.276346651201055,
-0.259153393254382,-0.254907740575419,-0.235952882819617,-0.223306156021738,
-0.218631602919718,-0.200333195629182,-0.182499890135021,-0.171713515924353,
-0.162763868116522,-0.158783796512119,-0.141685011629867,-0.139512866501546,
-0.121939884475205,-0.106697398915805,-0.103668917575034,-0.0868295933515879,
-0.0702531503661989,-0.0538124404507125,-0.0507919491436113,-0.0475503654479505,
-0.0317536154610128,-0.0158768077305064,-0.000838403874092872,0.),
 .UNSPECIFIED.);
#749=B_SPLINE_CURVE_WITH_KNOTS('',3,(#65212,#65213,#65214,#65215,#65216,
#65217,#65218,#65219,#65220,#65221,#65222,#65223,#65224,#65225,#65226,#65227,
#65228,#65229,#65230,#65231,#65232,#65233,#65234,#65235,#65236,#65237,#65238,
#65239,#65240,#65241,#65242,#65243,#65244,#65245,#65246,#65247,#65248,#65249,
#65250,#65251,#65252,#65253,#65254,#65255,#65256,#65257,#65258,#65259,#65260,
#65261,#65262,#65263,#65264,#65265,#65266,#65267,#65268,#65269,#65270,#65271,
#65272,#65273,#65274,#65275,#65276,#65277,#65278,#65279,#65280,#65281,#65282,
#65283,#65284,#65285,#65286,#65287,#65288,#65289,#65290),.UNSPECIFIED.,
 .F.,.F.,(4,3,3,3,3,3,3,3,3,3,3,3,3,3,3,3,3,3,3,3,3,3,3,3,3,3,4),(-0.300067541140094,
-0.284765732859265,-0.273496979675118,-0.269500054551934,-0.253423326962788,
-0.241927110787518,-0.238274241091951,-0.221422988791485,-0.204571736491019,
-0.193777643808902,-0.184331465755972,-0.181440948090128,-0.16362648013299,
-0.161395365762553,-0.144213237170065,-0.134885024745118,-0.128123522255208,
-0.123524962845352,-0.1055412340923,-0.086985134185087,-0.0684290342778744,
-0.0649136170042364,-0.0612783534074245,-0.0420227137929396,-0.0227330075651508,
-0.00361430569105197,0.),.UNSPECIFIED.);
#750=B_SPLINE_CURVE_WITH_KNOTS('',3,(#65548,#65549,#65550,#65551),
 .UNSPECIFIED.,.F.,.F.,(4,4),(-0.0234767871018056,0.),.UNSPECIFIED.);
#751=B_SPLINE_CURVE_WITH_KNOTS('',3,(#65552,#65553,#65554,#65555,#65556,
#65557,#65558,#65559,#65560,#65561,#65562,#65563,#65564,#65565,#65566,#65567,
#65568,#65569,#65570,#65571,#65572,#65573,#65574,#65575,#65576,#65577,#65578,
#65579,#65580,#65581,#65582,#65583,#65584,#65585,#65586,#65587,#65588,#65589,
#65590,#65591,#65592,#65593,#65594,#65595,#65596,#65597,#65598,#65599,#65600,
#65601,#65602,#65603,#65604,#65605,#65606,#65607,#65608,#65609,#65610,#65611,
#65612,#65613,#65614,#65615,#65616,#65617,#65618,#65619,#65620,#65621,#65622,
#65623,#65624,#65625,#65626,#65627,#65628,#65629,#65630),.UNSPECIFIED.,
 .F.,.F.,(4,3,3,3,3,3,3,3,3,3,3,3,3,3,3,3,3,3,3,3,3,3,3,3,3,3,4),(-0.300067541140075,
-0.284903775252137,-0.273496984748414,-0.269500055156834,-0.253431644196808,
-0.241927109392526,-0.238274239829673,-0.221422986437265,-0.204571733044858,
-0.193777641224282,-0.184331461696163,-0.181440940855814,-0.163626472874271,
-0.161395365762553,-0.144213236819044,-0.134885024154862,-0.128123521102825,
-0.12352496320423,-0.105490429091212,-0.0870510242177805,-0.0684290325616374,
-0.0649136213287457,-0.0612783543927973,-0.0420227138085096,-0.0227330091795879,
-0.00361430957713989,-2.23591124697115E-15),.UNSPECIFIED.);
#752=B_SPLINE_CURVE_WITH_KNOTS('',3,(#65635,#65636,#65637,#65638,#65639,
#65640,#65641,#65642,#65643,#65644,#65645,#65646,#65647,#65648,#65649,#65650,
#65651,#65652,#65653,#65654,#65655,#65656,#65657,#65658,#65659,#65660,#65661,
#65662,#65663,#65664,#65665,#65666,#65667,#65668,#65669,#65670,#65671,#65672,
#65673,#65674,#65675,#65676,#65677,#65678,#65679,#65680,#65681,#65682,#65683,
#65684,#65685,#65686,#65687,#65688,#65689,#65690,#65691,#65692,#65693,#65694,
#65695,#65696,#65697,#65698,#65699,#65700,#65701,#65702,#65703,#65704,#65705,
#65706,#65707,#65708,#65709,#65710),.UNSPECIFIED.,.F.,.F.,(4,3,3,3,3,3,
3,3,3,3,3,3,3,3,3,3,3,3,3,3,3,3,3,3,3,4),(-0.295806546771922,-0.276346658132916,
-0.259153396697353,-0.254907741902912,-0.235934549609346,-0.223306160924828,
-0.21863160323213,-0.200313417110245,-0.182506801147177,-0.171713519137717,
-0.162763872690389,-0.158783797445154,-0.141685015599876,-0.139512866501534,
-0.121934206365092,-0.106697398496199,-0.103668916910145,-0.0868283976391997,
-0.0701246001375039,-0.0538124336143781,-0.0507919606835372,-0.0475503673793636,
-0.0317536141940222,-0.0162960065267044,-0.000838398859386542,0.),
 .UNSPECIFIED.);
#753=B_SPLINE_CURVE_WITH_KNOTS('',3,(#65968,#65969,#65970,#65971),
 .UNSPECIFIED.,.F.,.F.,(4,4),(-0.0234767213281991,0.),.UNSPECIFIED.);
#901=B_SPLINE_SURFACE_WITH_KNOTS('',3,3,((#65292,#65293,#65294,#65295,#65296,
#65297,#65298,#65299,#65300,#65301,#65302,#65303,#65304,#65305,#65306,#65307,
#65308,#65309,#65310,#65311,#65312,#65313,#65314,#65315,#65316,#65317,#65318,
#65319,#65320,#65321,#65322,#65323,#65324,#65325,#65326,#65327,#65328,#65329,
#65330,#65331,#65332,#65333,#65334,#65335,#65336,#65337,#65338,#65339,#65340,
#65341,#65342,#65343,#65344,#65345,#65346,#65347,#65348,#65349,#65350,#65351,
#65352,#65353,#65354,#65355),(#65356,#65357,#65358,#65359,#65360,#65361,
#65362,#65363,#65364,#65365,#65366,#65367,#65368,#65369,#65370,#65371,#65372,
#65373,#65374,#65375,#65376,#65377,#65378,#65379,#65380,#65381,#65382,#65383,
#65384,#65385,#65386,#65387,#65388,#65389,#65390,#65391,#65392,#65393,#65394,
#65395,#65396,#65397,#65398,#65399,#65400,#65401,#65402,#65403,#65404,#65405,
#65406,#65407,#65408,#65409,#65410,#65411,#65412,#65413,#65414,#65415,#65416,
#65417,#65418,#65419),(#65420,#65421,#65422,#65423,#65424,#65425,#65426,
#65427,#65428,#65429,#65430,#65431,#65432,#65433,#65434,#65435,#65436,#65437,
#65438,#65439,#65440,#65441,#65442,#65443,#65444,#65445,#65446,#65447,#65448,
#65449,#65450,#65451,#65452,#65453,#65454,#65455,#65456,#65457,#65458,#65459,
#65460,#65461,#65462,#65463,#65464,#65465,#65466,#65467,#65468,#65469,#65470,
#65471,#65472,#65473,#65474,#65475,#65476,#65477,#65478,#65479,#65480,#65481,
#65482,#65483),(#65484,#65485,#65486,#65487,#65488,#65489,#65490,#65491,
#65492,#65493,#65494,#65495,#65496,#65497,#65498,#65499,#65500,#65501,#65502,
#65503,#65504,#65505,#65506,#65507,#65508,#65509,#65510,#65511,#65512,#65513,
#65514,#65515,#65516,#65517,#65518,#65519,#65520,#65521,#65522,#65523,#65524,
#65525,#65526,#65527,#65528,#65529,#65530,#65531,#65532,#65533,#65534,#65535,
#65536,#65537,#65538,#65539,#65540,#65541,#65542,#65543,#65544,#65545,#65546,
#65547)),.UNSPECIFIED.,.F.,.F.,.F.,(4,4),(4,1,1,1,1,1,1,1,1,1,1,1,1,1,1,
1,1,1,1,1,1,1,1,1,1,1,1,1,1,1,1,1,1,1,1,1,1,1,1,1,1,1,1,1,1,1,1,1,1,1,1,
1,1,1,1,1,1,1,1,1,1,4),(-0.000266152038421994,0.0504103259038983),(8.3394004212115,
9.33708834074415,10.3347762602768,11.3324641798094,12.3301520993421,13.3278400188747,
14.3255279384074,15.32321585794,16.3209037774727,17.3185916970053,18.3162796165379,
19.3139675360706,20.3116554556032,21.3093433751359,22.3070312946685,23.3047192142012,
24.3024071337338,25.3000950532664,26.2977829727991,27.2954708923317,28.2931588118644,
29.290846731397,30.2885346509297,31.2862225704623,32.283910489995,33.2815984095276,
34.2792863290602,35.2769742485929,36.2746621681255,37.2723500876582,38.2700380071908,
39.2677259267235,40.2654138462561,41.2631017657887,42.2607896853214,43.258477604854,
44.2561655243867,45.2538534439193,46.251541363452,47.2492292829846,48.2469172025173,
49.2446051220499,50.2422930415825,51.2399809611152,52.2376688806478,53.2353568001805,
54.2330447197131,55.2307326392458,56.2284205587784,57.226108478311,58.2237963978437,
59.2214843173763,60.219172236909,61.2168601564416,62.2145480759743,63.2122359955069,
64.2099239150396,65.2076118345722,66.2052997541048,67.2029876736375,68.2006755931701,
69.1986296647412),.UNSPECIFIED.);
#902=B_SPLINE_SURFACE_WITH_KNOTS('',3,3,((#65712,#65713,#65714,#65715,#65716,
#65717,#65718,#65719,#65720,#65721,#65722,#65723,#65724,#65725,#65726,#65727,
#65728,#65729,#65730,#65731,#65732,#65733,#65734,#65735,#65736,#65737,#65738,
#65739,#65740,#65741,#65742,#65743,#65744,#65745,#65746,#65747,#65748,#65749,
#65750,#65751,#65752,#65753,#65754,#65755,#65756,#65757,#65758,#65759,#65760,
#65761,#65762,#65763,#65764,#65765,#65766,#65767,#65768,#65769,#65770,#65771,
#65772,#65773,#65774,#65775),(#65776,#65777,#65778,#65779,#65780,#65781,
#65782,#65783,#65784,#65785,#65786,#65787,#65788,#65789,#65790,#65791,#65792,
#65793,#65794,#65795,#65796,#65797,#65798,#65799,#65800,#65801,#65802,#65803,
#65804,#65805,#65806,#65807,#65808,#65809,#65810,#65811,#65812,#65813,#65814,
#65815,#65816,#65817,#65818,#65819,#65820,#65821,#65822,#65823,#65824,#65825,
#65826,#65827,#65828,#65829,#65830,#65831,#65832,#65833,#65834,#65835,#65836,
#65837,#65838,#65839),(#65840,#65841,#65842,#65843,#65844,#65845,#65846,
#65847,#65848,#65849,#65850,#65851,#65852,#65853,#65854,#65855,#65856,#65857,
#65858,#65859,#65860,#65861,#65862,#65863,#65864,#65865,#65866,#65867,#65868,
#65869,#65870,#65871,#65872,#65873,#65874,#65875,#65876,#65877,#65878,#65879,
#65880,#65881,#65882,#65883,#65884,#65885,#65886,#65887,#65888,#65889,#65890,
#65891,#65892,#65893,#65894,#65895,#65896,#65897,#65898,#65899,#65900,#65901,
#65902,#65903),(#65904,#65905,#65906,#65907,#65908,#65909,#65910,#65911,
#65912,#65913,#65914,#65915,#65916,#65917,#65918,#65919,#65920,#65921,#65922,
#65923,#65924,#65925,#65926,#65927,#65928,#65929,#65930,#65931,#65932,#65933,
#65934,#65935,#65936,#65937,#65938,#65939,#65940,#65941,#65942,#65943,#65944,
#65945,#65946,#65947,#65948,#65949,#65950,#65951,#65952,#65953,#65954,#65955,
#65956,#65957,#65958,#65959,#65960,#65961,#65962,#65963,#65964,#65965,#65966,
#65967)),.UNSPECIFIED.,.F.,.F.,.F.,(4,4),(4,1,1,1,1,1,1,1,1,1,1,1,1,1,1,
1,1,1,1,1,1,1,1,1,1,1,1,1,1,1,1,1,1,1,1,1,1,1,1,1,1,1,1,1,1,1,1,1,1,1,1,
1,1,1,1,1,1,1,1,1,1,4),(-0.000246149933917203,0.0504194085446373),(11.6664599843382,
12.6644140492316,13.6621019687642,14.6597898882969,15.6574778078295,16.6551657273622,
17.6528536468948,18.6505415664274,19.6482294859601,20.6459174054927,21.6436053250254,
22.641293244558,23.6389811640907,24.6366690836233,25.634357003156,26.6320449226886,
27.6297328422212,28.6274207617539,29.6251086812865,30.6227966008192,31.6204845203518,
32.6181724398845,33.6158603594171,34.6135482789498,35.6112361984824,36.608924118015,
37.6066120375477,38.6042999570803,39.601987876613,40.5996757961456,41.5973637156783,
42.5950516352109,43.5927395547435,44.5904274742762,45.5881153938088,46.5858033133415,
47.5834912328741,48.5811791524068,49.5788670719394,50.5765549914721,51.5742429110047,
52.5719308305373,53.56961875007,54.5673066696026,55.5649945891353,56.5626825086679,
57.5603704282006,58.5580583477332,59.5557462672658,60.5534341867985,61.5511221063311,
62.5488100258638,63.5464979453964,64.5441858649291,65.5418737844617,66.5395617039943,
67.537249623527,68.5349375430596,69.5326254625923,70.5303133821249,71.5280013016576,
72.5256892211902),.UNSPECIFIED.);
#915=SHAPE_REPRESENTATION_RELATIONSHIP('SRR','None',#83310,#929);
#929=ADVANCED_BREP_SHAPE_REPRESENTATION('',(#957),#83215);
#943=STYLED_ITEM('',(#83389),#957);
#957=MANIFOLD_SOLID_BREP('Body1',#26939);
#1113=FACE_BOUND('',#4966,.T.);
#1114=FACE_BOUND('',#5080,.T.);
#1880=PLANE('',#28709);
#1881=PLANE('',#28712);
#1882=PLANE('',#28718);
#1883=PLANE('',#28722);
#1884=PLANE('',#28723);
#1885=PLANE('',#28724);
#1886=PLANE('',#28725);
#1887=PLANE('',#28765);
#1888=PLANE('',#28766);
#1889=PLANE('',#28767);
#1890=PLANE('',#28769);
#1891=PLANE('',#28770);
#1892=PLANE('',#28771);
#1893=PLANE('',#28773);
#1894=PLANE('',#28774);
#1895=PLANE('',#28775);
#1896=PLANE('',#28777);
#1897=PLANE('',#28778);
#1898=PLANE('',#28779);
#1899=PLANE('',#28781);
#1900=PLANE('',#28782);
#1901=PLANE('',#28783);
#1902=PLANE('',#28785);
#1903=PLANE('',#28786);
#1904=PLANE('',#28787);
#1905=PLANE('',#28789);
#1906=PLANE('',#28790);
#1907=PLANE('',#28791);
#1908=PLANE('',#28793);
#1909=PLANE('',#28794);
#1910=PLANE('',#28795);
#1911=PLANE('',#28797);
#1912=PLANE('',#28798);
#1913=PLANE('',#28799);
#1914=PLANE('',#28801);
#1915=PLANE('',#28802);
#1916=PLANE('',#28803);
#1917=PLANE('',#28805);
#1918=PLANE('',#28806);
#1919=PLANE('',#28807);
#1920=PLANE('',#28809);
#1921=PLANE('',#28810);
#1922=PLANE('',#28811);
#1923=PLANE('',#28813);
#1924=PLANE('',#28814);
#1925=PLANE('',#28815);
#1926=PLANE('',#28817);
#1927=PLANE('',#28818);
#1928=PLANE('',#28819);
#1929=PLANE('',#28821);
#1930=PLANE('',#28822);
#1931=PLANE('',#28823);
#1932=PLANE('',#28825);
#1933=PLANE('',#28826);
#1934=PLANE('',#28827);
#1935=PLANE('',#28829);
#1936=PLANE('',#28830);
#1937=PLANE('',#28831);
#1938=PLANE('',#28834);
#1939=PLANE('',#28835);
#1940=PLANE('',#28836);
#1941=PLANE('',#28838);
#1942=PLANE('',#28839);
#1943=PLANE('',#28840);
#1944=PLANE('',#28842);
#1945=PLANE('',#28843);
#1946=PLANE('',#28844);
#1947=PLANE('',#28846);
#1948=PLANE('',#28847);
#1949=PLANE('',#28848);
#1950=PLANE('',#28850);
#1951=PLANE('',#28851);
#1952=PLANE('',#28852);
#1953=PLANE('',#28854);
#1954=PLANE('',#28855);
#1955=PLANE('',#28856);
#1956=PLANE('',#28858);
#1957=PLANE('',#28859);
#1958=PLANE('',#28860);
#1959=PLANE('',#28862);
#1960=PLANE('',#28863);
#1961=PLANE('',#28864);
#1962=PLANE('',#28866);
#1963=PLANE('',#28867);
#1964=PLANE('',#28868);
#1965=PLANE('',#28870);
#1966=PLANE('',#28871);
#1967=PLANE('',#28872);
#1968=PLANE('',#28874);
#1969=PLANE('',#28875);
#1970=PLANE('',#28876);
#1971=PLANE('',#28878);
#1972=PLANE('',#28879);
#1973=PLANE('',#28880);
#1974=PLANE('',#28882);
#1975=PLANE('',#28883);
#1976=PLANE('',#28884);
#1977=PLANE('',#28886);
#1978=PLANE('',#28887);
#1979=PLANE('',#28888);
#1980=PLANE('',#28890);
#1981=PLANE('',#28891);
#1982=PLANE('',#28892);
#1983=PLANE('',#28894);
#1984=PLANE('',#28895);
#1985=PLANE('',#28896);
#1986=PLANE('',#28898);
#1987=PLANE('',#28899);
#1988=PLANE('',#28900);
#1989=PLANE('',#28902);
#1990=PLANE('',#28903);
#1991=PLANE('',#28904);
#1992=PLANE('',#28907);
#1993=PLANE('',#28908);
#1994=PLANE('',#28910);
#1995=PLANE('',#28912);
#1996=PLANE('',#28914);
#1997=PLANE('',#28916);
#1998=PLANE('',#28918);
#1999=PLANE('',#28921);
#2000=PLANE('',#28922);
#2001=PLANE('',#28923);
#2002=PLANE('',#28924);
#2003=PLANE('',#28925);
#2004=PLANE('',#28926);
#2318=CYLINDRICAL_SURFACE('',#28694,1.27);
#2319=CYLINDRICAL_SURFACE('',#28696,1.27);
#2320=CYLINDRICAL_SURFACE('',#28697,1.27);
#2321=CYLINDRICAL_SURFACE('',#28698,1.27);
#2322=CYLINDRICAL_SURFACE('',#28699,1.27);
#2323=CYLINDRICAL_SURFACE('',#28700,1.27);
#2324=CYLINDRICAL_SURFACE('',#28701,1.27);
#2325=CYLINDRICAL_SURFACE('',#28702,1.27);
#2326=CYLINDRICAL_SURFACE('',#28703,1.27);
#2327=CYLINDRICAL_SURFACE('',#28704,1.70434);
#2328=CYLINDRICAL_SURFACE('',#28707,1.27);
#2329=CYLINDRICAL_SURFACE('',#28906,2.8702);
#3418=FACE_OUTER_BOUND('',#4949,.T.);
#3419=FACE_OUTER_BOUND('',#4950,.T.);
#3420=FACE_OUTER_BOUND('',#4951,.T.);
#3421=FACE_OUTER_BOUND('',#4952,.T.);
#3422=FACE_OUTER_BOUND('',#4953,.T.);
#3423=FACE_OUTER_BOUND('',#4954,.T.);
#3424=FACE_OUTER_BOUND('',#4955,.T.);
#3425=FACE_OUTER_BOUND('',#4956,.T.);
#3426=FACE_OUTER_BOUND('',#4957,.T.);
#3427=FACE_OUTER_BOUND('',#4958,.T.);
#3428=FACE_OUTER_BOUND('',#4959,.T.);
#3429=FACE_OUTER_BOUND('',#4960,.T.);
#3430=FACE_OUTER_BOUND('',#4961,.T.);
#3431=FACE_OUTER_BOUND('',#4962,.T.);
#3432=FACE_OUTER_BOUND('',#4963,.T.);
#3433=FACE_OUTER_BOUND('',#4964,.T.);
#3434=FACE_OUTER_BOUND('',#4965,.T.);
#3435=FACE_OUTER_BOUND('',#4967,.T.);
#3436=FACE_OUTER_BOUND('',#4968,.T.);
#3437=FACE_OUTER_BOUND('',#4969,.T.);
#3438=FACE_OUTER_BOUND('',#4970,.T.);
#3439=FACE_OUTER_BOUND('',#4971,.T.);
#3440=FACE_OUTER_BOUND('',#4972,.T.);
#3441=FACE_OUTER_BOUND('',#4973,.T.);
#3442=FACE_OUTER_BOUND('',#4974,.T.);
#3443=FACE_OUTER_BOUND('',#4975,.T.);
#3444=FACE_OUTER_BOUND('',#4976,.T.);
#3445=FACE_OUTER_BOUND('',#4977,.T.);
#3446=FACE_OUTER_BOUND('',#4978,.T.);
#3447=FACE_OUTER_BOUND('',#4979,.T.);
#3448=FACE_OUTER_BOUND('',#4980,.T.);
#3449=FACE_OUTER_BOUND('',#4981,.T.);
#3450=FACE_OUTER_BOUND('',#4982,.T.);
#3451=FACE_OUTER_BOUND('',#4983,.T.);
#3452=FACE_OUTER_BOUND('',#4984,.T.);
#3453=FACE_OUTER_BOUND('',#4985,.T.);
#3454=FACE_OUTER_BOUND('',#4986,.T.);
#3455=FACE_OUTER_BOUND('',#4987,.T.);
#3456=FACE_OUTER_BOUND('',#4988,.T.);
#3457=FACE_OUTER_BOUND('',#4989,.T.);
#3458=FACE_OUTER_BOUND('',#4990,.T.);
#3459=FACE_OUTER_BOUND('',#4991,.T.);
#3460=FACE_OUTER_BOUND('',#4992,.T.);
#3461=FACE_OUTER_BOUND('',#4993,.T.);
#3462=FACE_OUTER_BOUND('',#4994,.T.);
#3463=FACE_OUTER_BOUND('',#4995,.T.);
#3464=FACE_OUTER_BOUND('',#4996,.T.);
#3465=FACE_OUTER_BOUND('',#4997,.T.);
#3466=FACE_OUTER_BOUND('',#4998,.T.);
#3467=FACE_OUTER_BOUND('',#4999,.T.);
#3468=FACE_OUTER_BOUND('',#5000,.T.);
#3469=FACE_OUTER_BOUND('',#5001,.T.);
#3470=FACE_OUTER_BOUND('',#5002,.T.);
#3471=FACE_OUTER_BOUND('',#5003,.T.);
#3472=FACE_OUTER_BOUND('',#5004,.T.);
#3473=FACE_OUTER_BOUND('',#5005,.T.);
#3474=FACE_OUTER_BOUND('',#5006,.T.);
#3475=FACE_OUTER_BOUND('',#5007,.T.);
#3476=FACE_OUTER_BOUND('',#5008,.T.);
#3477=FACE_OUTER_BOUND('',#5009,.T.);
#3478=FACE_OUTER_BOUND('',#5010,.T.);
#3479=FACE_OUTER_BOUND('',#5011,.T.);
#3480=FACE_OUTER_BOUND('',#5012,.T.);
#3481=FACE_OUTER_BOUND('',#5013,.T.);
#3482=FACE_OUTER_BOUND('',#5014,.T.);
#3483=FACE_OUTER_BOUND('',#5015,.T.);
#3484=FACE_OUTER_BOUND('',#5016,.T.);
#3485=FACE_OUTER_BOUND('',#5017,.T.);
#3486=FACE_OUTER_BOUND('',#5018,.T.);
#3487=FACE_OUTER_BOUND('',#5019,.T.);
#3488=FACE_OUTER_BOUND('',#5020,.T.);
#3489=FACE_OUTER_BOUND('',#5021,.T.);
#3490=FACE_OUTER_BOUND('',#5022,.T.);
#3491=FACE_OUTER_BOUND('',#5023,.T.);
#3492=FACE_OUTER_BOUND('',#5024,.T.);
#3493=FACE_OUTER_BOUND('',#5025,.T.);
#3494=FACE_OUTER_BOUND('',#5026,.T.);
#3495=FACE_OUTER_BOUND('',#5027,.T.);
#3496=FACE_OUTER_BOUND('',#5028,.T.);
#3497=FACE_OUTER_BOUND('',#5029,.T.);
#3498=FACE_OUTER_BOUND('',#5030,.T.);
#3499=FACE_OUTER_BOUND('',#5031,.T.);
#3500=FACE_OUTER_BOUND('',#5032,.T.);
#3501=FACE_OUTER_BOUND('',#5033,.T.);
#3502=FACE_OUTER_BOUND('',#5034,.T.);
#3503=FACE_OUTER_BOUND('',#5035,.T.);
#3504=FACE_OUTER_BOUND('',#5036,.T.);
#3505=FACE_OUTER_BOUND('',#5037,.T.);
#3506=FACE_OUTER_BOUND('',#5038,.T.);
#3507=FACE_OUTER_BOUND('',#5039,.T.);
#3508=FACE_OUTER_BOUND('',#5040,.T.);
#3509=FACE_OUTER_BOUND('',#5041,.T.);
#3510=FACE_OUTER_BOUND('',#5042,.T.);
#3511=FACE_OUTER_BOUND('',#5043,.T.);
#3512=FACE_OUTER_BOUND('',#5044,.T.);
#3513=FACE_OUTER_BOUND('',#5045,.T.);
#3514=FACE_OUTER_BOUND('',#5046,.T.);
#3515=FACE_OUTER_BOUND('',#5047,.T.);
#3516=FACE_OUTER_BOUND('',#5048,.T.);
#3517=FACE_OUTER_BOUND('',#5049,.T.);
#3518=FACE_OUTER_BOUND('',#5050,.T.);
#3519=FACE_OUTER_BOUND('',#5051,.T.);
#3520=FACE_OUTER_BOUND('',#5052,.T.);
#3521=FACE_OUTER_BOUND('',#5053,.T.);
#3522=FACE_OUTER_BOUND('',#5054,.T.);
#3523=FACE_OUTER_BOUND('',#5055,.T.);
#3524=FACE_OUTER_BOUND('',#5056,.T.);
#3525=FACE_OUTER_BOUND('',#5057,.T.);
#3526=FACE_OUTER_BOUND('',#5058,.T.);
#3527=FACE_OUTER_BOUND('',#5059,.T.);
#3528=FACE_OUTER_BOUND('',#5060,.T.);
#3529=FACE_OUTER_BOUND('',#5061,.T.);
#3530=FACE_OUTER_BOUND('',#5062,.T.);
#3531=FACE_OUTER_BOUND('',#5063,.T.);
#3532=FACE_OUTER_BOUND('',#5064,.T.);
#3533=FACE_OUTER_BOUND('',#5065,.T.);
#3534=FACE_OUTER_BOUND('',#5066,.T.);
#3535=FACE_OUTER_BOUND('',#5067,.T.);
#3536=FACE_OUTER_BOUND('',#5068,.T.);
#3537=FACE_OUTER_BOUND('',#5069,.T.);
#3538=FACE_OUTER_BOUND('',#5070,.T.);
#3539=FACE_OUTER_BOUND('',#5071,.T.);
#3540=FACE_OUTER_BOUND('',#5072,.T.);
#3541=FACE_OUTER_BOUND('',#5073,.T.);
#3542=FACE_OUTER_BOUND('',#5074,.T.);
#3543=FACE_OUTER_BOUND('',#5075,.T.);
#3544=FACE_OUTER_BOUND('',#5076,.T.);
#3545=FACE_OUTER_BOUND('',#5077,.T.);
#3546=FACE_OUTER_BOUND('',#5078,.T.);
#3547=FACE_OUTER_BOUND('',#5079,.T.);
#3548=FACE_OUTER_BOUND('',#5081,.T.);
#3549=FACE_OUTER_BOUND('',#5082,.T.);
#3550=FACE_OUTER_BOUND('',#5083,.T.);
#3551=FACE_OUTER_BOUND('',#5084,.T.);
#3552=FACE_OUTER_BOUND('',#5085,.T.);
#3553=FACE_OUTER_BOUND('',#5086,.T.);
#3554=FACE_OUTER_BOUND('',#5087,.T.);
#3555=FACE_OUTER_BOUND('',#5088,.T.);
#3556=FACE_OUTER_BOUND('',#5089,.T.);
#3557=FACE_OUTER_BOUND('',#5090,.T.);
#3558=FACE_OUTER_BOUND('',#5091,.T.);
#3559=FACE_OUTER_BOUND('',#5092,.T.);
#3560=FACE_OUTER_BOUND('',#5093,.T.);
#4949=EDGE_LOOP('',(#23500,#23501,#23502,#23503));
#4950=EDGE_LOOP('',(#23504,#23505,#23506,#23507,#23508,#23509));
#4951=EDGE_LOOP('',(#23510,#23511,#23512,#23513,#23514));
#4952=EDGE_LOOP('',(#23515,#23516,#23517,#23518,#23519,#23520));
#4953=EDGE_LOOP('',(#23521,#23522,#23523,#23524,#23525,#23526));
#4954=EDGE_LOOP('',(#23527,#23528,#23529,#23530,#23531));
#4955=EDGE_LOOP('',(#23532,#23533,#23534,#23535,#23536));
#4956=EDGE_LOOP('',(#23537,#23538,#23539,#23540,#23541));
#4957=EDGE_LOOP('',(#23542,#23543,#23544,#23545,#23546));
#4958=EDGE_LOOP('',(#23547,#23548,#23549,#23550,#23551,#23552,#23553,#23554,
#23555,#23556,#23557,#23558,#23559,#23560,#23561,#23562,#23563,#23564,#23565,
#23566,#23567,#23568,#23569,#23570));
#4959=EDGE_LOOP('',(#23571,#23572,#23573,#23574,#23575,#23576));
#4960=EDGE_LOOP('',(#23577,#23578,#23579,#23580,#23581));
#4961=EDGE_LOOP('',(#23582,#23583,#23584,#23585,#23586,#23587,#23588,#23589,
#23590,#23591,#23592,#23593,#23594,#23595,#23596,#23597,#23598,#23599,#23600,
#23601,#23602,#23603,#23604,#23605,#23606,#23607,#23608,#23609,#23610,#23611,
#23612));
#4962=EDGE_LOOP('',(#23613,#23614,#23615,#23616,#23617));
#4963=EDGE_LOOP('',(#23618,#23619,#23620,#23621,#23622,#23623,#23624,#23625,
#23626,#23627,#23628,#23629,#23630,#23631,#23632,#23633,#23634,#23635,#23636,
#23637,#23638,#23639,#23640,#23641,#23642,#23643,#23644,#23645,#23646,#23647));
#4964=EDGE_LOOP('',(#23648,#23649,#23650,#23651,#23652,#23653,#23654));
#4965=EDGE_LOOP('',(#23655));
#4966=EDGE_LOOP('',(#23656));
#4967=EDGE_LOOP('',(#23657,#23658,#23659,#23660,#23661,#23662,#23663));
#4968=EDGE_LOOP('',(#23664));
#4969=EDGE_LOOP('',(#23665,#23666,#23667,#23668));
#4970=EDGE_LOOP('',(#23669,#23670,#23671,#23672));
#4971=EDGE_LOOP('',(#23673,#23674,#23675));
#4972=EDGE_LOOP('',(#23676,#23677,#23678,#23679,#23680,#23681,#23682,#23683,
#23684,#23685,#23686,#23687,#23688,#23689,#23690,#23691,#23692,#23693,#23694,
#23695,#23696,#23697,#23698,#23699,#23700,#23701,#23702,#23703,#23704,#23705,
#23706,#23707,#23708,#23709,#23710,#23711,#23712,#23713,#23714,#23715,#23716,
#23717,#23718,#23719,#23720,#23721,#23722,#23723,#23724,#23725,#23726,#23727,
#23728,#23729,#23730,#23731,#23732,#23733,#23734,#23735,#23736,#23737,#23738,
#23739,#23740,#23741,#23742,#23743,#23744,#23745,#23746,#23747,#23748,#23749,
#23750,#23751,#23752,#23753,#23754,#23755,#23756,#23757,#23758,#23759,#23760,
#23761,#23762,#23763,#23764,#23765,#23766,#23767,#23768,#23769,#23770,#23771,
#23772,#23773,#23774,#23775,#23776,#23777,#23778,#23779,#23780,#23781,#23782,
#23783,#23784,#23785,#23786));
#4973=EDGE_LOOP('',(#23787,#23788,#23789,#23790));
#4974=EDGE_LOOP('',(#23791,#23792,#23793,#23794));
#4975=EDGE_LOOP('',(#23795,#23796,#23797));
#4976=EDGE_LOOP('',(#23798,#23799,#23800,#23801));
#4977=EDGE_LOOP('',(#23802,#23803,#23804,#23805));
#4978=EDGE_LOOP('',(#23806,#23807,#23808));
#4979=EDGE_LOOP('',(#23809,#23810,#23811,#23812));
#4980=EDGE_LOOP('',(#23813,#23814,#23815,#23816));
#4981=EDGE_LOOP('',(#23817,#23818,#23819));
#4982=EDGE_LOOP('',(#23820,#23821,#23822,#23823));
#4983=EDGE_LOOP('',(#23824,#23825,#23826,#23827));
#4984=EDGE_LOOP('',(#23828,#23829,#23830));
#4985=EDGE_LOOP('',(#23831,#23832,#23833,#23834));
#4986=EDGE_LOOP('',(#23835,#23836,#23837,#23838));
#4987=EDGE_LOOP('',(#23839,#23840,#23841));
#4988=EDGE_LOOP('',(#23842,#23843,#23844,#23845));
#4989=EDGE_LOOP('',(#23846,#23847,#23848,#23849));
#4990=EDGE_LOOP('',(#23850,#23851,#23852));
#4991=EDGE_LOOP('',(#23853,#23854,#23855,#23856));
#4992=EDGE_LOOP('',(#23857,#23858,#23859,#23860));
#4993=EDGE_LOOP('',(#23861,#23862,#23863));
#4994=EDGE_LOOP('',(#23864,#23865,#23866,#23867));
#4995=EDGE_LOOP('',(#23868,#23869,#23870,#23871));
#4996=EDGE_LOOP('',(#23872,#23873,#23874));
#4997=EDGE_LOOP('',(#23875,#23876,#23877,#23878));
#4998=EDGE_LOOP('',(#23879,#23880,#23881,#23882));
#4999=EDGE_LOOP('',(#23883,#23884,#23885));
#5000=EDGE_LOOP('',(#23886,#23887,#23888,#23889));
#5001=EDGE_LOOP('',(#23890,#23891,#23892,#23893));
#5002=EDGE_LOOP('',(#23894,#23895,#23896));
#5003=EDGE_LOOP('',(#23897,#23898,#23899,#23900));
#5004=EDGE_LOOP('',(#23901,#23902,#23903,#23904));
#5005=EDGE_LOOP('',(#23905,#23906,#23907));
#5006=EDGE_LOOP('',(#23908,#23909,#23910,#23911));
#5007=EDGE_LOOP('',(#23912,#23913,#23914,#23915));
#5008=EDGE_LOOP('',(#23916,#23917,#23918));
#5009=EDGE_LOOP('',(#23919,#23920,#23921,#23922));
#5010=EDGE_LOOP('',(#23923,#23924,#23925,#23926));
#5011=EDGE_LOOP('',(#23927,#23928,#23929));
#5012=EDGE_LOOP('',(#23930,#23931,#23932,#23933));
#5013=EDGE_LOOP('',(#23934,#23935,#23936,#23937));
#5014=EDGE_LOOP('',(#23938,#23939,#23940));
#5015=EDGE_LOOP('',(#23941,#23942,#23943,#23944));
#5016=EDGE_LOOP('',(#23945,#23946,#23947,#23948));
#5017=EDGE_LOOP('',(#23949,#23950,#23951));
#5018=EDGE_LOOP('',(#23952,#23953,#23954,#23955));
#5019=EDGE_LOOP('',(#23956,#23957,#23958,#23959));
#5020=EDGE_LOOP('',(#23960,#23961,#23962));
#5021=EDGE_LOOP('',(#23963,#23964,#23965,#23966));
#5022=EDGE_LOOP('',(#23967,#23968,#23969,#23970));
#5023=EDGE_LOOP('',(#23971,#23972,#23973,#23974));
#5024=EDGE_LOOP('',(#23975,#23976,#23977,#23978));
#5025=EDGE_LOOP('',(#23979,#23980,#23981,#23982));
#5026=EDGE_LOOP('',(#23983,#23984,#23985));
#5027=EDGE_LOOP('',(#23986,#23987,#23988,#23989));
#5028=EDGE_LOOP('',(#23990,#23991,#23992,#23993));
#5029=EDGE_LOOP('',(#23994,#23995,#23996));
#5030=EDGE_LOOP('',(#23997,#23998,#23999,#24000));
#5031=EDGE_LOOP('',(#24001,#24002,#24003,#24004));
#5032=EDGE_LOOP('',(#24005,#24006,#24007));
#5033=EDGE_LOOP('',(#24008,#24009,#24010,#24011));
#5034=EDGE_LOOP('',(#24012,#24013,#24014,#24015));
#5035=EDGE_LOOP('',(#24016,#24017,#24018));
#5036=EDGE_LOOP('',(#24019,#24020,#24021,#24022));
#5037=EDGE_LOOP('',(#24023,#24024,#24025,#24026));
#5038=EDGE_LOOP('',(#24027,#24028,#24029));
#5039=EDGE_LOOP('',(#24030,#24031,#24032,#24033));
#5040=EDGE_LOOP('',(#24034,#24035,#24036,#24037));
#5041=EDGE_LOOP('',(#24038,#24039,#24040));
#5042=EDGE_LOOP('',(#24041,#24042,#24043,#24044));
#5043=EDGE_LOOP('',(#24045,#24046,#24047,#24048));
#5044=EDGE_LOOP('',(#24049,#24050,#24051));
#5045=EDGE_LOOP('',(#24052,#24053,#24054,#24055));
#5046=EDGE_LOOP('',(#24056,#24057,#24058,#24059));
#5047=EDGE_LOOP('',(#24060,#24061,#24062));
#5048=EDGE_LOOP('',(#24063,#24064,#24065,#24066));
#5049=EDGE_LOOP('',(#24067,#24068,#24069,#24070));
#5050=EDGE_LOOP('',(#24071,#24072,#24073));
#5051=EDGE_LOOP('',(#24074,#24075,#24076,#24077));
#5052=EDGE_LOOP('',(#24078,#24079,#24080,#24081));
#5053=EDGE_LOOP('',(#24082,#24083,#24084));
#5054=EDGE_LOOP('',(#24085,#24086,#24087,#24088));
#5055=EDGE_LOOP('',(#24089,#24090,#24091,#24092));
#5056=EDGE_LOOP('',(#24093,#24094,#24095));
#5057=EDGE_LOOP('',(#24096,#24097,#24098,#24099));
#5058=EDGE_LOOP('',(#24100,#24101,#24102,#24103));
#5059=EDGE_LOOP('',(#24104,#24105,#24106));
#5060=EDGE_LOOP('',(#24107,#24108,#24109,#24110));
#5061=EDGE_LOOP('',(#24111,#24112,#24113,#24114));
#5062=EDGE_LOOP('',(#24115,#24116,#24117));
#5063=EDGE_LOOP('',(#24118,#24119,#24120,#24121));
#5064=EDGE_LOOP('',(#24122,#24123,#24124,#24125));
#5065=EDGE_LOOP('',(#24126,#24127,#24128));
#5066=EDGE_LOOP('',(#24129,#24130,#24131,#24132));
#5067=EDGE_LOOP('',(#24133,#24134,#24135,#24136));
#5068=EDGE_LOOP('',(#24137,#24138,#24139));
#5069=EDGE_LOOP('',(#24140,#24141,#24142,#24143));
#5070=EDGE_LOOP('',(#24144,#24145,#24146,#24147));
#5071=EDGE_LOOP('',(#24148,#24149,#24150));
#5072=EDGE_LOOP('',(#24151,#24152,#24153,#24154));
#5073=EDGE_LOOP('',(#24155,#24156,#24157,#24158));
#5074=EDGE_LOOP('',(#24159,#24160,#24161));
#5075=EDGE_LOOP('',(#24162,#24163,#24164,#24165));
#5076=EDGE_LOOP('',(#24166,#24167,#24168,#24169));
#5077=EDGE_LOOP('',(#24170,#24171,#24172));
#5078=EDGE_LOOP('',(#24173,#24174,#24175,#24176,#24177,#24178,#24179,#24180,
#24181,#24182,#24183,#24184,#24185,#24186,#24187,#24188,#24189,#24190,#24191,
#24192,#24193,#24194,#24195,#24196,#24197,#24198,#24199,#24200,#24201,#24202,
#24203,#24204,#24205,#24206,#24207,#24208,#24209,#24210,#24211,#24212,#24213,
#24214,#24215,#24216,#24217,#24218,#24219,#24220,#24221,#24222,#24223,#24224,
#24225,#24226,#24227,#24228,#24229,#24230,#24231,#24232,#24233,#24234,#24235,
#24236,#24237,#24238,#24239,#24240,#24241,#24242,#24243,#24244,#24245,#24246,
#24247,#24248,#24249,#24250,#24251,#24252,#24253,#24254,#24255,#24256,#24257,
#24258,#24259,#24260,#24261,#24262,#24263,#24264,#24265,#24266,#24267,#24268,
#24269,#24270,#24271,#24272,#24273,#24274,#24275,#24276,#24277,#24278,#24279,
#24280,#24281,#24282,#24283,#24284,#24285,#24286,#24287,#24288,#24289,#24290,
#24291,#24292,#24293,#24294,#24295,#24296,#24297,#24298,#24299,#24300,#24301,
#24302,#24303,#24304,#24305,#24306,#24307,#24308,#24309,#24310,#24311,#24312,
#24313,#24314,#24315,#24316,#24317,#24318,#24319,#24320));
#5079=EDGE_LOOP('',(#24321));
#5080=EDGE_LOOP('',(#24322,#24323,#24324,#24325,#24326,#24327));
#5081=EDGE_LOOP('',(#24328,#24329));
#5082=EDGE_LOOP('',(#24330,#24331));
#5083=EDGE_LOOP('',(#24332,#24333));
#5084=EDGE_LOOP('',(#24334,#24335));
#5085=EDGE_LOOP('',(#24336,#24337));
#5086=EDGE_LOOP('',(#24338,#24339));
#5087=EDGE_LOOP('',(#24340,#24341,#24342,#24343,#24344,#24345,#24346,#24347));
#5088=EDGE_LOOP('',(#24348,#24349,#24350,#24351));
#5089=EDGE_LOOP('',(#24352,#24353,#24354,#24355));
#5090=EDGE_LOOP('',(#24356,#24357,#24358,#24359));
#5091=EDGE_LOOP('',(#24360,#24361,#24362,#24363));
#5092=EDGE_LOOP('',(#24364,#24365,#24366,#24367));
#5093=EDGE_LOOP('',(#24368,#24369,#24370,#24371));
#7334=LINE('',#59387,#9845);
#7335=LINE('',#59609,#9846);
#7336=LINE('',#59942,#9847);
#7337=LINE('',#60138,#9848);
#7338=LINE('',#60335,#9849);
#7339=LINE('',#60514,#9850);
#7340=LINE('',#60814,#9851);
#7341=LINE('',#61133,#9852);
#7342=LINE('',#61454,#9853);
#7343=LINE('',#65981,#9854);
#7344=LINE('',#65987,#9855);
#7345=LINE('',#65989,#9856);
#7346=LINE('',#65991,#9857);
#7347=LINE('',#65998,#9858);
#7348=LINE('',#66002,#9859);
#7349=LINE('',#66358,#9860);
#7350=LINE('',#66362,#9861);
#7351=LINE('',#66364,#9862);
#7352=LINE('',#66365,#9863);
#7353=LINE('',#66368,#9864);
#7354=LINE('',#66369,#9865);
#7355=LINE('',#66374,#9866);
#7356=LINE('',#66376,#9867);
#7357=LINE('',#66377,#9868);
#7358=LINE('',#66380,#9869);
#7359=LINE('',#66381,#9870);
#7360=LINE('',#66386,#9871);
#7361=LINE('',#66388,#9872);
#7362=LINE('',#66389,#9873);
#7363=LINE('',#66392,#9874);
#7364=LINE('',#66393,#9875);
#7365=LINE('',#66398,#9876);
#7366=LINE('',#66400,#9877);
#7367=LINE('',#66401,#9878);
#7368=LINE('',#66404,#9879);
#7369=LINE('',#66405,#9880);
#7370=LINE('',#66410,#9881);
#7371=LINE('',#66412,#9882);
#7372=LINE('',#66413,#9883);
#7373=LINE('',#66416,#9884);
#7374=LINE('',#66417,#9885);
#7375=LINE('',#66422,#9886);
#7376=LINE('',#66424,#9887);
#7377=LINE('',#66425,#9888);
#7378=LINE('',#66428,#9889);
#7379=LINE('',#66429,#9890);
#7380=LINE('',#66434,#9891);
#7381=LINE('',#66436,#9892);
#7382=LINE('',#66437,#9893);
#7383=LINE('',#66440,#9894);
#7384=LINE('',#66441,#9895);
#7385=LINE('',#66446,#9896);
#7386=LINE('',#66448,#9897);
#7387=LINE('',#66449,#9898);
#7388=LINE('',#66452,#9899);
#7389=LINE('',#66453,#9900);
#7390=LINE('',#66458,#9901);
#7391=LINE('',#66460,#9902);
#7392=LINE('',#66461,#9903);
#7393=LINE('',#66464,#9904);
#7394=LINE('',#66465,#9905);
#7395=LINE('',#66470,#9906);
#7396=LINE('',#66472,#9907);
#7397=LINE('',#66473,#9908);
#7398=LINE('',#66476,#9909);
#7399=LINE('',#66477,#9910);
#7400=LINE('',#66482,#9911);
#7401=LINE('',#66484,#9912);
#7402=LINE('',#66485,#9913);
#7403=LINE('',#66488,#9914);
#7404=LINE('',#66489,#9915);
#7405=LINE('',#66494,#9916);
#7406=LINE('',#66496,#9917);
#7407=LINE('',#66497,#9918);
#7408=LINE('',#66500,#9919);
#7409=LINE('',#66501,#9920);
#7410=LINE('',#66506,#9921);
#7411=LINE('',#66508,#9922);
#7412=LINE('',#66509,#9923);
#7413=LINE('',#66512,#9924);
#7414=LINE('',#66513,#9925);
#7415=LINE('',#66518,#9926);
#7416=LINE('',#66520,#9927);
#7417=LINE('',#66521,#9928);
#7418=LINE('',#66524,#9929);
#7419=LINE('',#66525,#9930);
#7420=LINE('',#66530,#9931);
#7421=LINE('',#66532,#9932);
#7422=LINE('',#66533,#9933);
#7423=LINE('',#66536,#9934);
#7424=LINE('',#66537,#9935);
#7425=LINE('',#66542,#9936);
#7426=LINE('',#66544,#9937);
#7427=LINE('',#66545,#9938);
#7428=LINE('',#66548,#9939);
#7429=LINE('',#66549,#9940);
#7430=LINE('',#66554,#9941);
#7431=LINE('',#66556,#9942);
#7432=LINE('',#66557,#9943);
#7433=LINE('',#66560,#9944);
#7434=LINE('',#66561,#9945);
#7435=LINE('',#66568,#9946);
#7436=LINE('',#66570,#9947);
#7437=LINE('',#66571,#9948);
#7438=LINE('',#66574,#9949);
#7439=LINE('',#66575,#9950);
#7440=LINE('',#66580,#9951);
#7441=LINE('',#66582,#9952);
#7442=LINE('',#66583,#9953);
#7443=LINE('',#66586,#9954);
#7444=LINE('',#66587,#9955);
#7445=LINE('',#66592,#9956);
#7446=LINE('',#66594,#9957);
#7447=LINE('',#66595,#9958);
#7448=LINE('',#66598,#9959);
#7449=LINE('',#66599,#9960);
#7450=LINE('',#66604,#9961);
#7451=LINE('',#66606,#9962);
#7452=LINE('',#66607,#9963);
#7453=LINE('',#66610,#9964);
#7454=LINE('',#66611,#9965);
#7455=LINE('',#66616,#9966);
#7456=LINE('',#66618,#9967);
#7457=LINE('',#66619,#9968);
#7458=LINE('',#66622,#9969);
#7459=LINE('',#66623,#9970);
#7460=LINE('',#66628,#9971);
#7461=LINE('',#66630,#9972);
#7462=LINE('',#66631,#9973);
#7463=LINE('',#66634,#9974);
#7464=LINE('',#66635,#9975);
#7465=LINE('',#66640,#9976);
#7466=LINE('',#66642,#9977);
#7467=LINE('',#66643,#9978);
#7468=LINE('',#66646,#9979);
#7469=LINE('',#66647,#9980);
#7470=LINE('',#66652,#9981);
#7471=LINE('',#66654,#9982);
#7472=LINE('',#66655,#9983);
#7473=LINE('',#66658,#9984);
#7474=LINE('',#66659,#9985);
#7475=LINE('',#66664,#9986);
#7476=LINE('',#66666,#9987);
#7477=LINE('',#66667,#9988);
#7478=LINE('',#66670,#9989);
#7479=LINE('',#66671,#9990);
#7480=LINE('',#66676,#9991);
#7481=LINE('',#66678,#9992);
#7482=LINE('',#66679,#9993);
#7483=LINE('',#66682,#9994);
#7484=LINE('',#66683,#9995);
#7485=LINE('',#66688,#9996);
#7486=LINE('',#66690,#9997);
#7487=LINE('',#66691,#9998);
#7488=LINE('',#66694,#9999);
#7489=LINE('',#66695,#10000);
#7490=LINE('',#66700,#10001);
#7491=LINE('',#66702,#10002);
#7492=LINE('',#66703,#10003);
#7493=LINE('',#66706,#10004);
#7494=LINE('',#66707,#10005);
#7495=LINE('',#66712,#10006);
#7496=LINE('',#66714,#10007);
#7497=LINE('',#66715,#10008);
#7498=LINE('',#66718,#10009);
#7499=LINE('',#66719,#10010);
#7500=LINE('',#66724,#10011);
#7501=LINE('',#66726,#10012);
#7502=LINE('',#66727,#10013);
#7503=LINE('',#66730,#10014);
#7504=LINE('',#66731,#10015);
#7505=LINE('',#66736,#10016);
#7506=LINE('',#66738,#10017);
#7507=LINE('',#66739,#10018);
#7508=LINE('',#66742,#10019);
#7509=LINE('',#66743,#10020);
#7510=LINE('',#66748,#10021);
#7511=LINE('',#66750,#10022);
#7512=LINE('',#66751,#10023);
#7513=LINE('',#66754,#10024);
#7514=LINE('',#66755,#10025);
#7515=LINE('',#66760,#10026);
#7516=LINE('',#66762,#10027);
#7517=LINE('',#66763,#10028);
#7518=LINE('',#66766,#10029);
#7519=LINE('',#66767,#10030);
#7520=LINE('',#66772,#10031);
#7521=LINE('',#66774,#10032);
#7522=LINE('',#66775,#10033);
#7523=LINE('',#66778,#10034);
#7524=LINE('',#66779,#10035);
#7525=LINE('',#66783,#10036);
#7526=LINE('',#66787,#10037);
#7527=LINE('',#66789,#10038);
#7528=LINE('',#66791,#10039);
#7529=LINE('',#66793,#10040);
#7530=LINE('',#66795,#10041);
#7531=LINE('',#66796,#10042);
#7532=LINE('',#66800,#10043);
#7533=LINE('',#66804,#10044);
#7534=LINE('',#66808,#10045);
#7535=LINE('',#66812,#10046);
#7536=LINE('',#66816,#10047);
#7537=LINE('',#66819,#10048);
#7538=LINE('',#66823,#10049);
#7539=LINE('',#66825,#10050);
#7540=LINE('',#66826,#10051);
#7541=LINE('',#66828,#10052);
#7542=LINE('',#66830,#10053);
#7543=LINE('',#66832,#10054);
#7544=LINE('',#66834,#10055);
#9845=VECTOR('',#34506,1.27);
#9846=VECTOR('',#34511,1.27);
#9847=VECTOR('',#34514,1.27);
#9848=VECTOR('',#34517,1.27);
#9849=VECTOR('',#34520,1.27);
#9850=VECTOR('',#34523,1.27);
#9851=VECTOR('',#34526,1.27);
#9852=VECTOR('',#34529,1.27);
#9853=VECTOR('',#34532,1.27);
#9854=VECTOR('',#34567,1.52934);
#9855=VECTOR('',#34574,10.);
#9856=VECTOR('',#34575,10.);
#9857=VECTOR('',#34576,10.);
#9858=VECTOR('',#34579,10.);
#9859=VECTOR('',#34580,10.);
#9860=VECTOR('',#34659,2.7202);
#9861=VECTOR('',#34664,10.);
#9862=VECTOR('',#34665,10.);
#9863=VECTOR('',#34666,10.);
#9864=VECTOR('',#34669,10.);
#9865=VECTOR('',#34670,10.);
#9866=VECTOR('',#34677,10.);
#9867=VECTOR('',#34678,10.);
#9868=VECTOR('',#34679,10.);
#9869=VECTOR('',#34682,10.);
#9870=VECTOR('',#34683,10.);
#9871=VECTOR('',#34690,10.);
#9872=VECTOR('',#34691,10.);
#9873=VECTOR('',#34692,10.);
#9874=VECTOR('',#34695,10.);
#9875=VECTOR('',#34696,10.);
#9876=VECTOR('',#34703,10.);
#9877=VECTOR('',#34704,10.);
#9878=VECTOR('',#34705,10.);
#9879=VECTOR('',#34708,10.);
#9880=VECTOR('',#34709,10.);
#9881=VECTOR('',#34716,10.);
#9882=VECTOR('',#34717,10.);
#9883=VECTOR('',#34718,10.);
#9884=VECTOR('',#34721,10.);
#9885=VECTOR('',#34722,10.);
#9886=VECTOR('',#34729,10.);
#9887=VECTOR('',#34730,10.);
#9888=VECTOR('',#34731,10.);
#9889=VECTOR('',#34734,10.);
#9890=VECTOR('',#34735,10.);
#9891=VECTOR('',#34742,10.);
#9892=VECTOR('',#34743,10.);
#9893=VECTOR('',#34744,10.);
#9894=VECTOR('',#34747,10.);
#9895=VECTOR('',#34748,10.);
#9896=VECTOR('',#34755,10.);
#9897=VECTOR('',#34756,10.);
#9898=VECTOR('',#34757,10.);
#9899=VECTOR('',#34760,10.);
#9900=VECTOR('',#34761,10.);
#9901=VECTOR('',#34768,10.);
#9902=VECTOR('',#34769,10.);
#9903=VECTOR('',#34770,10.);
#9904=VECTOR('',#34773,10.);
#9905=VECTOR('',#34774,10.);
#9906=VECTOR('',#34781,10.);
#9907=VECTOR('',#34782,9.99999999999999);
#9908=VECTOR('',#34783,10.);
#9909=VECTOR('',#34786,10.);
#9910=VECTOR('',#34787,10.);
#9911=VECTOR('',#34794,10.);
#9912=VECTOR('',#34795,10.);
#9913=VECTOR('',#34796,10.);
#9914=VECTOR('',#34799,10.);
#9915=VECTOR('',#34800,10.);
#9916=VECTOR('',#34807,10.);
#9917=VECTOR('',#34808,10.);
#9918=VECTOR('',#34809,10.);
#9919=VECTOR('',#34812,10.);
#9920=VECTOR('',#34813,10.);
#9921=VECTOR('',#34820,10.);
#9922=VECTOR('',#34821,10.);
#9923=VECTOR('',#34822,10.);
#9924=VECTOR('',#34825,10.);
#9925=VECTOR('',#34826,10.);
#9926=VECTOR('',#34833,10.);
#9927=VECTOR('',#34834,10.);
#9928=VECTOR('',#34835,10.);
#9929=VECTOR('',#34838,10.);
#9930=VECTOR('',#34839,10.);
#9931=VECTOR('',#34846,10.);
#9932=VECTOR('',#34847,10.);
#9933=VECTOR('',#34848,10.);
#9934=VECTOR('',#34851,10.);
#9935=VECTOR('',#34852,10.);
#9936=VECTOR('',#34859,10.);
#9937=VECTOR('',#34860,10.);
#9938=VECTOR('',#34861,10.);
#9939=VECTOR('',#34864,10.);
#9940=VECTOR('',#34865,10.);
#9941=VECTOR('',#34872,10.);
#9942=VECTOR('',#34873,10.);
#9943=VECTOR('',#34874,10.);
#9944=VECTOR('',#34877,10.);
#9945=VECTOR('',#34878,10.);
#9946=VECTOR('',#34887,10.);
#9947=VECTOR('',#34888,10.);
#9948=VECTOR('',#34889,10.);
#9949=VECTOR('',#34892,10.);
#9950=VECTOR('',#34893,10.);
#9951=VECTOR('',#34900,10.);
#9952=VECTOR('',#34901,10.);
#9953=VECTOR('',#34902,10.);
#9954=VECTOR('',#34905,10.);
#9955=VECTOR('',#34906,10.);
#9956=VECTOR('',#34913,10.);
#9957=VECTOR('',#34914,10.);
#9958=VECTOR('',#34915,10.);
#9959=VECTOR('',#34918,10.);
#9960=VECTOR('',#34919,10.);
#9961=VECTOR('',#34926,10.);
#9962=VECTOR('',#34927,10.);
#9963=VECTOR('',#34928,10.);
#9964=VECTOR('',#34931,10.);
#9965=VECTOR('',#34932,10.);
#9966=VECTOR('',#34939,10.);
#9967=VECTOR('',#34940,10.);
#9968=VECTOR('',#34941,10.);
#9969=VECTOR('',#34944,10.);
#9970=VECTOR('',#34945,10.);
#9971=VECTOR('',#34952,10.);
#9972=VECTOR('',#34953,10.);
#9973=VECTOR('',#34954,10.);
#9974=VECTOR('',#34957,10.);
#9975=VECTOR('',#34958,10.);
#9976=VECTOR('',#34965,10.);
#9977=VECTOR('',#34966,10.);
#9978=VECTOR('',#34967,10.);
#9979=VECTOR('',#34970,10.);
#9980=VECTOR('',#34971,10.);
#9981=VECTOR('',#34978,10.);
#9982=VECTOR('',#34979,10.);
#9983=VECTOR('',#34980,10.);
#9984=VECTOR('',#34983,10.);
#9985=VECTOR('',#34984,10.);
#9986=VECTOR('',#34991,10.);
#9987=VECTOR('',#34992,10.);
#9988=VECTOR('',#34993,10.);
#9989=VECTOR('',#34996,10.);
#9990=VECTOR('',#34997,10.);
#9991=VECTOR('',#35004,10.);
#9992=VECTOR('',#35005,10.);
#9993=VECTOR('',#35006,10.);
#9994=VECTOR('',#35009,10.);
#9995=VECTOR('',#35010,10.);
#9996=VECTOR('',#35017,10.);
#9997=VECTOR('',#35018,9.99999999999999);
#9998=VECTOR('',#35019,10.);
#9999=VECTOR('',#35022,10.);
#10000=VECTOR('',#35023,10.);
#10001=VECTOR('',#35030,10.);
#10002=VECTOR('',#35031,10.);
#10003=VECTOR('',#35032,10.);
#10004=VECTOR('',#35035,10.);
#10005=VECTOR('',#35036,10.);
#10006=VECTOR('',#35043,10.);
#10007=VECTOR('',#35044,10.);
#10008=VECTOR('',#35045,10.);
#10009=VECTOR('',#35048,10.);
#10010=VECTOR('',#35049,10.);
#10011=VECTOR('',#35056,10.);
#10012=VECTOR('',#35057,10.);
#10013=VECTOR('',#35058,10.);
#10014=VECTOR('',#35061,10.);
#10015=VECTOR('',#35062,10.);
#10016=VECTOR('',#35069,10.);
#10017=VECTOR('',#35070,10.);
#10018=VECTOR('',#35071,10.);
#10019=VECTOR('',#35074,10.);
#10020=VECTOR('',#35075,10.);
#10021=VECTOR('',#35082,10.);
#10022=VECTOR('',#35083,10.);
#10023=VECTOR('',#35084,10.);
#10024=VECTOR('',#35087,10.);
#10025=VECTOR('',#35088,10.);
#10026=VECTOR('',#35095,10.);
#10027=VECTOR('',#35096,9.99999999999999);
#10028=VECTOR('',#35097,10.);
#10029=VECTOR('',#35100,10.);
#10030=VECTOR('',#35101,10.);
#10031=VECTOR('',#35108,10.);
#10032=VECTOR('',#35109,10.);
#10033=VECTOR('',#35110,10.);
#10034=VECTOR('',#35113,10.);
#10035=VECTOR('',#35114,10.);
#10036=VECTOR('',#35121,2.8702);
#10037=VECTOR('',#35124,10.);
#10038=VECTOR('',#35125,10.);
#10039=VECTOR('',#35126,10.);
#10040=VECTOR('',#35127,10.);
#10041=VECTOR('',#35128,10.);
#10042=VECTOR('',#35129,10.);
#10043=VECTOR('',#35132,10.);
#10044=VECTOR('',#35137,10.);
#10045=VECTOR('',#35142,10.);
#10046=VECTOR('',#35147,10.);
#10047=VECTOR('',#35152,10.);
#10048=VECTOR('',#35157,10.);
#10049=VECTOR('',#35162,1.60395121659243);
#10050=VECTOR('',#35165,10.);
#10051=VECTOR('',#35166,10.);
#10052=VECTOR('',#35169,10.);
#10053=VECTOR('',#35172,10.);
#10054=VECTOR('',#35175,10.);
#10055=VECTOR('',#35178,10.);
#10852=CIRCLE('',#28695,1.27);
#10853=CIRCLE('',#28705,1.70434);
#10854=CIRCLE('',#28706,1.70434);
#10855=CIRCLE('',#28708,1.27);
#10856=CIRCLE('',#28710,1.70434);
#10857=CIRCLE('',#28711,1.70434);
#10858=CIRCLE('',#28713,1.70434);
#10859=CIRCLE('',#28714,1.70434);
#10860=CIRCLE('',#28716,1.85434);
#10861=CIRCLE('',#28717,0.15);
#10862=CIRCLE('',#28719,2.8702);
#10863=CIRCLE('',#28721,1.35434);
#10864=CIRCLE('',#28726,2.8702);
#10865=CIRCLE('',#28728,2.8702);
#10866=CIRCLE('',#28729,2.8702);
#10867=CIRCLE('',#28730,2.8702);
#10868=CIRCLE('',#28731,2.8702);
#10869=CIRCLE('',#28732,2.8702);
#10870=CIRCLE('',#28733,2.8702);
#10871=CIRCLE('',#28734,2.8702);
#10872=CIRCLE('',#28735,2.8702);
#10873=CIRCLE('',#28736,2.8702);
#10874=CIRCLE('',#28737,2.8702);
#10875=CIRCLE('',#28738,2.8702);
#10876=CIRCLE('',#28739,2.8702);
#10877=CIRCLE('',#28740,2.8702);
#10878=CIRCLE('',#28741,2.8702);
#10879=CIRCLE('',#28742,2.8702);
#10880=CIRCLE('',#28743,2.8702);
#10881=CIRCLE('',#28744,2.8702);
#10882=CIRCLE('',#28745,2.8702);
#10883=CIRCLE('',#28746,2.8702);
#10884=CIRCLE('',#28747,2.8702);
#10885=CIRCLE('',#28748,2.8702);
#10886=CIRCLE('',#28749,2.8702);
#10887=CIRCLE('',#28750,2.8702);
#10888=CIRCLE('',#28751,2.8702);
#10889=CIRCLE('',#28752,2.8702);
#10890=CIRCLE('',#28753,2.8702);
#10891=CIRCLE('',#28754,2.8702);
#10892=CIRCLE('',#28755,2.8702);
#10893=CIRCLE('',#28756,2.8702);
#10894=CIRCLE('',#28757,2.8702);
#10895=CIRCLE('',#28758,2.8702);
#10896=CIRCLE('',#28759,2.8702);
#10897=CIRCLE('',#28760,2.8702);
#10898=CIRCLE('',#28761,2.8702);
#10899=CIRCLE('',#28762,2.8702);
#10900=CIRCLE('',#28763,2.8702);
#10901=CIRCLE('',#28764,2.5702);
#10902=CIRCLE('',#28768,2.8702);
#10903=CIRCLE('',#28772,2.8702);
#10904=CIRCLE('',#28776,2.8702);
#10905=CIRCLE('',#28780,2.8702);
#10906=CIRCLE('',#28784,2.8702);
#10907=CIRCLE('',#28788,2.8702);
#10908=CIRCLE('',#28792,2.8702);
#10909=CIRCLE('',#28796,2.8702);
#10910=CIRCLE('',#28800,2.8702);
#10911=CIRCLE('',#28804,2.8702);
#10912=CIRCLE('',#28808,2.8702);
#10913=CIRCLE('',#28812,2.8702);
#10914=CIRCLE('',#28816,2.8702);
#10915=CIRCLE('',#28820,2.8702);
#10916=CIRCLE('',#28824,2.8702);
#10917=CIRCLE('',#28828,2.8702);
#10918=CIRCLE('',#28832,2.8702);
#10919=CIRCLE('',#28833,2.8702);
#10920=CIRCLE('',#28837,2.8702);
#10921=CIRCLE('',#28841,2.8702);
#10922=CIRCLE('',#28845,2.8702);
#10923=CIRCLE('',#28849,2.8702);
#10924=CIRCLE('',#28853,2.8702);
#10925=CIRCLE('',#28857,2.8702);
#10926=CIRCLE('',#28861,2.8702);
#10927=CIRCLE('',#28865,2.8702);
#10928=CIRCLE('',#28869,2.8702);
#10929=CIRCLE('',#28873,2.8702);
#10930=CIRCLE('',#28877,2.8702);
#10931=CIRCLE('',#28881,2.8702);
#10932=CIRCLE('',#28885,2.8702);
#10933=CIRCLE('',#28889,2.8702);
#10934=CIRCLE('',#28893,2.8702);
#10935=CIRCLE('',#28897,2.8702);
#10936=CIRCLE('',#28901,2.8702);
#10937=CIRCLE('',#28905,2.8702);
#10938=CIRCLE('',#28909,1.60395121659243);
#10939=CIRCLE('',#28911,1.60395121659243);
#10940=CIRCLE('',#28913,1.60395121659243);
#10941=CIRCLE('',#28915,1.60395121659243);
#10942=CIRCLE('',#28917,1.60395121659243);
#10943=CIRCLE('',#28919,1.60395121659243);
#12983=VERTEX_POINT('',#59385);
#12984=VERTEX_POINT('',#59386);
#12985=VERTEX_POINT('',#59388);
#12986=VERTEX_POINT('',#59516);
#12987=VERTEX_POINT('',#59607);
#12988=VERTEX_POINT('',#59608);
#12989=VERTEX_POINT('',#59610);
#12990=VERTEX_POINT('',#59781);
#12991=VERTEX_POINT('',#59940);
#12992=VERTEX_POINT('',#59941);
#12993=VERTEX_POINT('',#59943);
#12994=VERTEX_POINT('',#60136);
#12995=VERTEX_POINT('',#60137);
#12996=VERTEX_POINT('',#60139);
#12997=VERTEX_POINT('',#60295);
#12998=VERTEX_POINT('',#60333);
#12999=VERTEX_POINT('',#60334);
#13000=VERTEX_POINT('',#60336);
#13001=VERTEX_POINT('',#60368);
#13002=VERTEX_POINT('',#60512);
#13003=VERTEX_POINT('',#60513);
#13004=VERTEX_POINT('',#60515);
#13005=VERTEX_POINT('',#60812);
#13006=VERTEX_POINT('',#60813);
#13007=VERTEX_POINT('',#60971);
#13008=VERTEX_POINT('',#61131);
#13009=VERTEX_POINT('',#61132);
#13010=VERTEX_POINT('',#61134);
#13011=VERTEX_POINT('',#61452);
#13012=VERTEX_POINT('',#61453);
#13013=VERTEX_POINT('',#61605);
#13014=VERTEX_POINT('',#61781);
#13015=VERTEX_POINT('',#61782);
#13016=VERTEX_POINT('',#61844);
#13017=VERTEX_POINT('',#61846);
#13018=VERTEX_POINT('',#61852);
#13019=VERTEX_POINT('',#62031);
#13020=VERTEX_POINT('',#62207);
#13021=VERTEX_POINT('',#62380);
#13022=VERTEX_POINT('',#62553);
#13023=VERTEX_POINT('',#62729);
#13024=VERTEX_POINT('',#62902);
#13025=VERTEX_POINT('',#63072);
#13026=VERTEX_POINT('',#63245);
#13027=VERTEX_POINT('',#63421);
#13028=VERTEX_POINT('',#63459);
#13029=VERTEX_POINT('',#63461);
#13030=VERTEX_POINT('',#63469);
#13031=VERTEX_POINT('',#63480);
#13032=VERTEX_POINT('',#63653);
#13033=VERTEX_POINT('',#63823);
#13034=VERTEX_POINT('',#63996);
#13035=VERTEX_POINT('',#64169);
#13036=VERTEX_POINT('',#64342);
#13037=VERTEX_POINT('',#64515);
#13038=VERTEX_POINT('',#64861);
#13039=VERTEX_POINT('',#64887);
#13040=VERTEX_POINT('',#65015);
#13041=VERTEX_POINT('',#65017);
#13042=VERTEX_POINT('',#65133);
#13043=VERTEX_POINT('',#65134);
#13044=VERTEX_POINT('',#65632);
#13045=VERTEX_POINT('',#65633);
#13046=VERTEX_POINT('',#65973);
#13047=VERTEX_POINT('',#65977);
#13048=VERTEX_POINT('',#65980);
#13049=VERTEX_POINT('',#65985);
#13050=VERTEX_POINT('',#65986);
#13051=VERTEX_POINT('',#65988);
#13052=VERTEX_POINT('',#65990);
#13053=VERTEX_POINT('',#65996);
#13054=VERTEX_POINT('',#65997);
#13055=VERTEX_POINT('',#66006);
#13056=VERTEX_POINT('',#66007);
#13057=VERTEX_POINT('',#66011);
#13058=VERTEX_POINT('',#66013);
#13059=VERTEX_POINT('',#66017);
#13060=VERTEX_POINT('',#66021);
#13061=VERTEX_POINT('',#66023);
#13062=VERTEX_POINT('',#66027);
#13063=VERTEX_POINT('',#66031);
#13064=VERTEX_POINT('',#66033);
#13065=VERTEX_POINT('',#66037);
#13066=VERTEX_POINT('',#66041);
#13067=VERTEX_POINT('',#66043);
#13068=VERTEX_POINT('',#66047);
#13069=VERTEX_POINT('',#66051);
#13070=VERTEX_POINT('',#66053);
#13071=VERTEX_POINT('',#66057);
#13072=VERTEX_POINT('',#66061);
#13073=VERTEX_POINT('',#66063);
#13074=VERTEX_POINT('',#66067);
#13075=VERTEX_POINT('',#66071);
#13076=VERTEX_POINT('',#66073);
#13077=VERTEX_POINT('',#66077);
#13078=VERTEX_POINT('',#66081);
#13079=VERTEX_POINT('',#66083);
#13080=VERTEX_POINT('',#66087);
#13081=VERTEX_POINT('',#66091);
#13082=VERTEX_POINT('',#66093);
#13083=VERTEX_POINT('',#66097);
#13084=VERTEX_POINT('',#66101);
#13085=VERTEX_POINT('',#66103);
#13086=VERTEX_POINT('',#66107);
#13087=VERTEX_POINT('',#66111);
#13088=VERTEX_POINT('',#66113);
#13089=VERTEX_POINT('',#66117);
#13090=VERTEX_POINT('',#66121);
#13091=VERTEX_POINT('',#66123);
#13092=VERTEX_POINT('',#66127);
#13093=VERTEX_POINT('',#66131);
#13094=VERTEX_POINT('',#66133);
#13095=VERTEX_POINT('',#66137);
#13096=VERTEX_POINT('',#66141);
#13097=VERTEX_POINT('',#66143);
#13098=VERTEX_POINT('',#66147);
#13099=VERTEX_POINT('',#66151);
#13100=VERTEX_POINT('',#66153);
#13101=VERTEX_POINT('',#66157);
#13102=VERTEX_POINT('',#66161);
#13103=VERTEX_POINT('',#66163);
#13104=VERTEX_POINT('',#66167);
#13105=VERTEX_POINT('',#66171);
#13106=VERTEX_POINT('',#66173);
#13107=VERTEX_POINT('',#66177);
#13108=VERTEX_POINT('',#66181);
#13109=VERTEX_POINT('',#66183);
#13110=VERTEX_POINT('',#66187);
#13111=VERTEX_POINT('',#66192);
#13112=VERTEX_POINT('',#66194);
#13113=VERTEX_POINT('',#66198);
#13114=VERTEX_POINT('',#66202);
#13115=VERTEX_POINT('',#66204);
#13116=VERTEX_POINT('',#66208);
#13117=VERTEX_POINT('',#66212);
#13118=VERTEX_POINT('',#66214);
#13119=VERTEX_POINT('',#66218);
#13120=VERTEX_POINT('',#66222);
#13121=VERTEX_POINT('',#66224);
#13122=VERTEX_POINT('',#66228);
#13123=VERTEX_POINT('',#66232);
#13124=VERTEX_POINT('',#66234);
#13125=VERTEX_POINT('',#66238);
#13126=VERTEX_POINT('',#66242);
#13127=VERTEX_POINT('',#66244);
#13128=VERTEX_POINT('',#66248);
#13129=VERTEX_POINT('',#66252);
#13130=VERTEX_POINT('',#66254);
#13131=VERTEX_POINT('',#66258);
#13132=VERTEX_POINT('',#66262);
#13133=VERTEX_POINT('',#66264);
#13134=VERTEX_POINT('',#66268);
#13135=VERTEX_POINT('',#66272);
#13136=VERTEX_POINT('',#66274);
#13137=VERTEX_POINT('',#66278);
#13138=VERTEX_POINT('',#66282);
#13139=VERTEX_POINT('',#66284);
#13140=VERTEX_POINT('',#66288);
#13141=VERTEX_POINT('',#66292);
#13142=VERTEX_POINT('',#66294);
#13143=VERTEX_POINT('',#66298);
#13144=VERTEX_POINT('',#66302);
#13145=VERTEX_POINT('',#66304);
#13146=VERTEX_POINT('',#66308);
#13147=VERTEX_POINT('',#66312);
#13148=VERTEX_POINT('',#66314);
#13149=VERTEX_POINT('',#66318);
#13150=VERTEX_POINT('',#66322);
#13151=VERTEX_POINT('',#66324);
#13152=VERTEX_POINT('',#66328);
#13153=VERTEX_POINT('',#66332);
#13154=VERTEX_POINT('',#66334);
#13155=VERTEX_POINT('',#66338);
#13156=VERTEX_POINT('',#66342);
#13157=VERTEX_POINT('',#66344);
#13158=VERTEX_POINT('',#66348);
#13159=VERTEX_POINT('',#66352);
#13160=VERTEX_POINT('',#66357);
#13161=VERTEX_POINT('',#66361);
#13162=VERTEX_POINT('',#66363);
#13163=VERTEX_POINT('',#66367);
#13164=VERTEX_POINT('',#66373);
#13165=VERTEX_POINT('',#66375);
#13166=VERTEX_POINT('',#66379);
#13167=VERTEX_POINT('',#66385);
#13168=VERTEX_POINT('',#66387);
#13169=VERTEX_POINT('',#66391);
#13170=VERTEX_POINT('',#66397);
#13171=VERTEX_POINT('',#66399);
#13172=VERTEX_POINT('',#66403);
#13173=VERTEX_POINT('',#66409);
#13174=VERTEX_POINT('',#66411);
#13175=VERTEX_POINT('',#66415);
#13176=VERTEX_POINT('',#66421);
#13177=VERTEX_POINT('',#66423);
#13178=VERTEX_POINT('',#66427);
#13179=VERTEX_POINT('',#66433);
#13180=VERTEX_POINT('',#66435);
#13181=VERTEX_POINT('',#66439);
#13182=VERTEX_POINT('',#66445);
#13183=VERTEX_POINT('',#66447);
#13184=VERTEX_POINT('',#66451);
#13185=VERTEX_POINT('',#66457);
#13186=VERTEX_POINT('',#66459);
#13187=VERTEX_POINT('',#66463);
#13188=VERTEX_POINT('',#66469);
#13189=VERTEX_POINT('',#66471);
#13190=VERTEX_POINT('',#66475);
#13191=VERTEX_POINT('',#66481);
#13192=VERTEX_POINT('',#66483);
#13193=VERTEX_POINT('',#66487);
#13194=VERTEX_POINT('',#66493);
#13195=VERTEX_POINT('',#66495);
#13196=VERTEX_POINT('',#66499);
#13197=VERTEX_POINT('',#66505);
#13198=VERTEX_POINT('',#66507);
#13199=VERTEX_POINT('',#66511);
#13200=VERTEX_POINT('',#66517);
#13201=VERTEX_POINT('',#66519);
#13202=VERTEX_POINT('',#66523);
#13203=VERTEX_POINT('',#66529);
#13204=VERTEX_POINT('',#66531);
#13205=VERTEX_POINT('',#66535);
#13206=VERTEX_POINT('',#66541);
#13207=VERTEX_POINT('',#66543);
#13208=VERTEX_POINT('',#66547);
#13209=VERTEX_POINT('',#66553);
#13210=VERTEX_POINT('',#66555);
#13211=VERTEX_POINT('',#66559);
#13212=VERTEX_POINT('',#66563);
#13213=VERTEX_POINT('',#66567);
#13214=VERTEX_POINT('',#66569);
#13215=VERTEX_POINT('',#66573);
#13216=VERTEX_POINT('',#66579);
#13217=VERTEX_POINT('',#66581);
#13218=VERTEX_POINT('',#66585);
#13219=VERTEX_POINT('',#66591);
#13220=VERTEX_POINT('',#66593);
#13221=VERTEX_POINT('',#66597);
#13222=VERTEX_POINT('',#66603);
#13223=VERTEX_POINT('',#66605);
#13224=VERTEX_POINT('',#66609);
#13225=VERTEX_POINT('',#66615);
#13226=VERTEX_POINT('',#66617);
#13227=VERTEX_POINT('',#66621);
#13228=VERTEX_POINT('',#66627);
#13229=VERTEX_POINT('',#66629);
#13230=VERTEX_POINT('',#66633);
#13231=VERTEX_POINT('',#66639);
#13232=VERTEX_POINT('',#66641);
#13233=VERTEX_POINT('',#66645);
#13234=VERTEX_POINT('',#66651);
#13235=VERTEX_POINT('',#66653);
#13236=VERTEX_POINT('',#66657);
#13237=VERTEX_POINT('',#66663);
#13238=VERTEX_POINT('',#66665);
#13239=VERTEX_POINT('',#66669);
#13240=VERTEX_POINT('',#66675);
#13241=VERTEX_POINT('',#66677);
#13242=VERTEX_POINT('',#66681);
#13243=VERTEX_POINT('',#66687);
#13244=VERTEX_POINT('',#66689);
#13245=VERTEX_POINT('',#66693);
#13246=VERTEX_POINT('',#66699);
#13247=VERTEX_POINT('',#66701);
#13248=VERTEX_POINT('',#66705);
#13249=VERTEX_POINT('',#66711);
#13250=VERTEX_POINT('',#66713);
#13251=VERTEX_POINT('',#66717);
#13252=VERTEX_POINT('',#66723);
#13253=VERTEX_POINT('',#66725);
#13254=VERTEX_POINT('',#66729);
#13255=VERTEX_POINT('',#66735);
#13256=VERTEX_POINT('',#66737);
#13257=VERTEX_POINT('',#66741);
#13258=VERTEX_POINT('',#66747);
#13259=VERTEX_POINT('',#66749);
#13260=VERTEX_POINT('',#66753);
#13261=VERTEX_POINT('',#66759);
#13262=VERTEX_POINT('',#66761);
#13263=VERTEX_POINT('',#66765);
#13264=VERTEX_POINT('',#66771);
#13265=VERTEX_POINT('',#66773);
#13266=VERTEX_POINT('',#66777);
#13267=VERTEX_POINT('',#66785);
#13268=VERTEX_POINT('',#66786);
#13269=VERTEX_POINT('',#66788);
#13270=VERTEX_POINT('',#66790);
#13271=VERTEX_POINT('',#66792);
#13272=VERTEX_POINT('',#66794);
#13273=VERTEX_POINT('',#66798);
#13274=VERTEX_POINT('',#66799);
#13275=VERTEX_POINT('',#66803);
#13276=VERTEX_POINT('',#66807);
#13277=VERTEX_POINT('',#66811);
#13278=VERTEX_POINT('',#66815);
#13279=VERTEX_POINT('',#66822);
#16611=EDGE_CURVE('',#12983,#12984,#7334,.T.);
#16612=EDGE_CURVE('',#12985,#12983,#693,.T.);
#16613=EDGE_CURVE('',#12986,#12985,#10852,.T.);
#16614=EDGE_CURVE('',#12986,#12984,#694,.T.);
#16615=EDGE_CURVE('',#12987,#12988,#7335,.T.);
#16616=EDGE_CURVE('',#12989,#12987,#695,.T.);
#16617=EDGE_CURVE('',#12983,#12989,#696,.T.);
#16618=EDGE_CURVE('',#12984,#12990,#697,.T.);
#16619=EDGE_CURVE('',#12990,#12988,#698,.T.);
#16620=EDGE_CURVE('',#12991,#12992,#7336,.T.);
#16621=EDGE_CURVE('',#12993,#12991,#699,.T.);
#16622=EDGE_CURVE('',#12987,#12993,#700,.T.);
#16623=EDGE_CURVE('',#12988,#12992,#701,.T.);
#16624=EDGE_CURVE('',#12994,#12995,#7337,.T.);
#16625=EDGE_CURVE('',#12996,#12994,#702,.T.);
#16626=EDGE_CURVE('',#12991,#12996,#703,.T.);
#16627=EDGE_CURVE('',#12992,#12997,#704,.T.);
#16628=EDGE_CURVE('',#12997,#12995,#705,.T.);
#16629=EDGE_CURVE('',#12998,#12999,#7338,.T.);
#16630=EDGE_CURVE('',#13000,#12998,#706,.T.);
#16631=EDGE_CURVE('',#12994,#13000,#707,.T.);
#16632=EDGE_CURVE('',#12995,#13001,#708,.T.);
#16633=EDGE_CURVE('',#13001,#12999,#709,.T.);
#16634=EDGE_CURVE('',#13002,#13003,#7339,.T.);
#16635=EDGE_CURVE('',#13004,#13002,#710,.F.);
#16636=EDGE_CURVE('',#12998,#13004,#711,.T.);
#16637=EDGE_CURVE('',#12999,#13003,#712,.T.);
#16638=EDGE_CURVE('',#13005,#13006,#7340,.T.);
#16639=EDGE_CURVE('',#13002,#13005,#713,.F.);
#16640=EDGE_CURVE('',#13003,#13007,#714,.T.);
#16641=EDGE_CURVE('',#13007,#13006,#715,.T.);
#16642=EDGE_CURVE('',#13008,#13009,#7341,.T.);
#16643=EDGE_CURVE('',#13010,#13008,#716,.F.);
#16644=EDGE_CURVE('',#13005,#13010,#717,.F.);
#16645=EDGE_CURVE('',#13006,#13009,#718,.T.);
#16646=EDGE_CURVE('',#13011,#13012,#7342,.T.);
#16647=EDGE_CURVE('',#13008,#13011,#719,.F.);
#16648=EDGE_CURVE('',#13009,#13013,#720,.T.);
#16649=EDGE_CURVE('',#13013,#13012,#721,.T.);
#16650=EDGE_CURVE('',#13014,#13015,#722,.T.);
#16651=EDGE_CURVE('',#13016,#13015,#10853,.T.);
#16652=EDGE_CURVE('',#13016,#13017,#723,.T.);
#16653=EDGE_CURVE('',#13017,#13018,#724,.T.);
#16654=EDGE_CURVE('',#13018,#13019,#725,.T.);
#16655=EDGE_CURVE('',#13019,#13020,#726,.T.);
#16656=EDGE_CURVE('',#13020,#13021,#727,.T.);
#16657=EDGE_CURVE('',#13021,#13022,#728,.T.);
#16658=EDGE_CURVE('',#13022,#13023,#729,.T.);
#16659=EDGE_CURVE('',#13023,#13024,#730,.T.);
#16660=EDGE_CURVE('',#13024,#13025,#731,.T.);
#16661=EDGE_CURVE('',#13025,#13026,#732,.T.);
#16662=EDGE_CURVE('',#13026,#13027,#733,.T.);
#16663=EDGE_CURVE('',#13028,#13027,#10854,.T.);
#16664=EDGE_CURVE('',#13028,#13029,#734,.T.);
#16665=EDGE_CURVE('',#13029,#13030,#735,.T.);
#16666=EDGE_CURVE('',#13030,#13031,#736,.T.);
#16667=EDGE_CURVE('',#13031,#13032,#737,.T.);
#16668=EDGE_CURVE('',#13032,#13033,#738,.T.);
#16669=EDGE_CURVE('',#13033,#13034,#739,.T.);
#16670=EDGE_CURVE('',#13034,#13035,#740,.T.);
#16671=EDGE_CURVE('',#13035,#13036,#741,.T.);
#16672=EDGE_CURVE('',#13036,#13037,#742,.T.);
#16673=EDGE_CURVE('',#13037,#13014,#743,.T.);
#16674=EDGE_CURVE('',#13012,#13038,#744,.T.);
#16675=EDGE_CURVE('',#13038,#13039,#745,.T.);
#16676=EDGE_CURVE('',#13040,#13039,#10855,.T.);
#16677=EDGE_CURVE('',#13041,#13040,#746,.T.);
#16678=EDGE_CURVE('',#13011,#13041,#747,.F.);
#16679=EDGE_CURVE('',#13042,#13043,#10856,.T.);
#16680=EDGE_CURVE('',#13042,#13040,#748,.T.);
#16681=EDGE_CURVE('',#13039,#13028,#749,.T.);
#16682=EDGE_CURVE('',#13043,#13028,#10857,.T.);
#16683=EDGE_CURVE('',#13027,#13042,#750,.T.);
#16684=EDGE_CURVE('',#12985,#13016,#751,.T.);
#16685=EDGE_CURVE('',#13044,#13045,#10858,.T.);
#16686=EDGE_CURVE('',#13044,#12986,#752,.T.);
#16687=EDGE_CURVE('',#13045,#13016,#10859,.T.);
#16688=EDGE_CURVE('',#13015,#13044,#753,.T.);
#16689=EDGE_CURVE('',#13046,#13046,#10860,.T.);
#16690=EDGE_CURVE('',#13046,#13045,#10861,.T.);
#16691=EDGE_CURVE('',#13047,#13047,#10862,.T.);
#16692=EDGE_CURVE('',#13043,#13048,#7343,.T.);
#16693=EDGE_CURVE('',#13048,#13048,#10863,.T.);
#16694=EDGE_CURVE('',#13049,#13050,#7344,.T.);
#16695=EDGE_CURVE('',#13049,#13051,#7345,.T.);
#16696=EDGE_CURVE('',#13052,#13051,#7346,.T.);
#16697=EDGE_CURVE('',#13050,#13052,#353,.T.);
#16698=EDGE_CURVE('',#13053,#13054,#7347,.T.);
#16699=EDGE_CURVE('',#13052,#13053,#354,.T.);
#16700=EDGE_CURVE('',#13051,#13054,#7348,.T.);
#16701=EDGE_CURVE('',#13054,#13049,#10864,.T.);
#16702=EDGE_CURVE('',#13055,#13056,#355,.T.);
#16703=EDGE_CURVE('',#13056,#13057,#10865,.T.);
#16704=EDGE_CURVE('',#13057,#13058,#356,.T.);
#16705=EDGE_CURVE('',#13058,#13059,#357,.T.);
#16706=EDGE_CURVE('',#13059,#13060,#10866,.T.);
#16707=EDGE_CURVE('',#13060,#13061,#358,.T.);
#16708=EDGE_CURVE('',#13061,#13062,#359,.T.);
#16709=EDGE_CURVE('',#13062,#13063,#10867,.T.);
#16710=EDGE_CURVE('',#13063,#13064,#360,.T.);
#16711=EDGE_CURVE('',#13064,#13065,#361,.T.);
#16712=EDGE_CURVE('',#13065,#13066,#10868,.T.);
#16713=EDGE_CURVE('',#13066,#13067,#362,.T.);
#16714=EDGE_CURVE('',#13067,#13068,#363,.T.);
#16715=EDGE_CURVE('',#13068,#13069,#10869,.T.);
#16716=EDGE_CURVE('',#13069,#13070,#364,.T.);
#16717=EDGE_CURVE('',#13070,#13071,#365,.T.);
#16718=EDGE_CURVE('',#13071,#13072,#10870,.T.);
#16719=EDGE_CURVE('',#13072,#13073,#366,.T.);
#16720=EDGE_CURVE('',#13073,#13074,#367,.T.);
#16721=EDGE_CURVE('',#13074,#13075,#10871,.T.);
#16722=EDGE_CURVE('',#13075,#13076,#368,.T.);
#16723=EDGE_CURVE('',#13076,#13077,#369,.T.);
#16724=EDGE_CURVE('',#13077,#13078,#10872,.T.);
#16725=EDGE_CURVE('',#13078,#13079,#370,.T.);
#16726=EDGE_CURVE('',#13079,#13080,#371,.T.);
#16727=EDGE_CURVE('',#13080,#13081,#10873,.T.);
#16728=EDGE_CURVE('',#13081,#13082,#372,.T.);
#16729=EDGE_CURVE('',#13082,#13083,#373,.T.);
#16730=EDGE_CURVE('',#13083,#13084,#10874,.T.);
#16731=EDGE_CURVE('',#13084,#13085,#374,.T.);
#16732=EDGE_CURVE('',#13085,#13086,#375,.T.);
#16733=EDGE_CURVE('',#13086,#13087,#10875,.T.);
#16734=EDGE_CURVE('',#13087,#13088,#376,.T.);
#16735=EDGE_CURVE('',#13088,#13089,#377,.T.);
#16736=EDGE_CURVE('',#13089,#13090,#10876,.T.);
#16737=EDGE_CURVE('',#13090,#13091,#378,.T.);
#16738=EDGE_CURVE('',#13091,#13092,#379,.T.);
#16739=EDGE_CURVE('',#13092,#13093,#10877,.T.);
#16740=EDGE_CURVE('',#13093,#13094,#380,.T.);
#16741=EDGE_CURVE('',#13094,#13095,#381,.T.);
#16742=EDGE_CURVE('',#13095,#13096,#10878,.T.);
#16743=EDGE_CURVE('',#13096,#13097,#382,.T.);
#16744=EDGE_CURVE('',#13097,#13098,#383,.T.);
#16745=EDGE_CURVE('',#13098,#13099,#10879,.T.);
#16746=EDGE_CURVE('',#13099,#13100,#384,.T.);
#16747=EDGE_CURVE('',#13100,#13101,#385,.T.);
#16748=EDGE_CURVE('',#13101,#13102,#10880,.T.);
#16749=EDGE_CURVE('',#13102,#13103,#386,.T.);
#16750=EDGE_CURVE('',#13103,#13104,#387,.T.);
#16751=EDGE_CURVE('',#13104,#13105,#10881,.T.);
#16752=EDGE_CURVE('',#13105,#13106,#388,.T.);
#16753=EDGE_CURVE('',#13106,#13107,#389,.T.);
#16754=EDGE_CURVE('',#13107,#13108,#10882,.T.);
#16755=EDGE_CURVE('',#13108,#13109,#390,.T.);
#16756=EDGE_CURVE('',#13109,#13110,#391,.T.);
#16757=EDGE_CURVE('',#13110,#13050,#10883,.T.);
#16758=EDGE_CURVE('',#13053,#13111,#10884,.T.);
#16759=EDGE_CURVE('',#13111,#13112,#392,.T.);
#16760=EDGE_CURVE('',#13112,#13113,#393,.T.);
#16761=EDGE_CURVE('',#13113,#13114,#10885,.T.);
#16762=EDGE_CURVE('',#13114,#13115,#394,.T.);
#16763=EDGE_CURVE('',#13115,#13116,#395,.T.);
#16764=EDGE_CURVE('',#13116,#13117,#10886,.T.);
#16765=EDGE_CURVE('',#13117,#13118,#396,.T.);
#16766=EDGE_CURVE('',#13118,#13119,#397,.T.);
#16767=EDGE_CURVE('',#13119,#13120,#10887,.T.);
#16768=EDGE_CURVE('',#13120,#13121,#398,.T.);
#16769=EDGE_CURVE('',#13121,#13122,#399,.T.);
#16770=EDGE_CURVE('',#13122,#13123,#10888,.T.);
#16771=EDGE_CURVE('',#13123,#13124,#400,.T.);
#16772=EDGE_CURVE('',#13124,#13125,#401,.T.);
#16773=EDGE_CURVE('',#13125,#13126,#10889,.T.);
#16774=EDGE_CURVE('',#13126,#13127,#402,.T.);
#16775=EDGE_CURVE('',#13127,#13128,#403,.T.);
#16776=EDGE_CURVE('',#13128,#13129,#10890,.T.);
#16777=EDGE_CURVE('',#13129,#13130,#404,.T.);
#16778=EDGE_CURVE('',#13130,#13131,#405,.T.);
#16779=EDGE_CURVE('',#13131,#13132,#10891,.T.);
#16780=EDGE_CURVE('',#13132,#13133,#406,.T.);
#16781=EDGE_CURVE('',#13133,#13134,#407,.T.);
#16782=EDGE_CURVE('',#13134,#13135,#10892,.T.);
#16783=EDGE_CURVE('',#13135,#13136,#408,.T.);
#16784=EDGE_CURVE('',#13136,#13137,#409,.T.);
#16785=EDGE_CURVE('',#13137,#13138,#10893,.T.);
#16786=EDGE_CURVE('',#13138,#13139,#410,.T.);
#16787=EDGE_CURVE('',#13139,#13140,#411,.T.);
#16788=EDGE_CURVE('',#13140,#13141,#10894,.T.);
#16789=EDGE_CURVE('',#13141,#13142,#412,.T.);
#16790=EDGE_CURVE('',#13142,#13143,#413,.T.);
#16791=EDGE_CURVE('',#13143,#13144,#10895,.T.);
#16792=EDGE_CURVE('',#13144,#13145,#414,.T.);
#16793=EDGE_CURVE('',#13145,#13146,#415,.T.);
#16794=EDGE_CURVE('',#13146,#13147,#10896,.T.);
#16795=EDGE_CURVE('',#13147,#13148,#416,.T.);
#16796=EDGE_CURVE('',#13148,#13149,#417,.T.);
#16797=EDGE_CURVE('',#13149,#13150,#10897,.T.);
#16798=EDGE_CURVE('',#13150,#13151,#418,.T.);
#16799=EDGE_CURVE('',#13151,#13152,#419,.T.);
#16800=EDGE_CURVE('',#13152,#13153,#10898,.T.);
#16801=EDGE_CURVE('',#13153,#13154,#420,.T.);
#16802=EDGE_CURVE('',#13154,#13155,#421,.T.);
#16803=EDGE_CURVE('',#13155,#13156,#10899,.T.);
#16804=EDGE_CURVE('',#13156,#13157,#422,.T.);
#16805=EDGE_CURVE('',#13157,#13158,#423,.T.);
#16806=EDGE_CURVE('',#13158,#13159,#10900,.T.);
#16807=EDGE_CURVE('',#13159,#13055,#424,.T.);
#16808=EDGE_CURVE('',#13055,#13160,#7349,.T.);
#16809=EDGE_CURVE('',#13160,#13160,#10901,.T.);
#16810=EDGE_CURVE('',#13161,#13111,#7350,.T.);
#16811=EDGE_CURVE('',#13161,#13162,#7351,.T.);
#16812=EDGE_CURVE('',#13112,#13162,#7352,.T.);
#16813=EDGE_CURVE('',#13113,#13163,#7353,.T.);
#16814=EDGE_CURVE('',#13162,#13163,#7354,.T.);
#16815=EDGE_CURVE('',#13163,#13161,#10902,.T.);
#16816=EDGE_CURVE('',#13164,#13114,#7355,.T.);
#16817=EDGE_CURVE('',#13164,#13165,#7356,.T.);
#16818=EDGE_CURVE('',#13115,#13165,#7357,.T.);
#16819=EDGE_CURVE('',#13116,#13166,#7358,.T.);
#16820=EDGE_CURVE('',#13165,#13166,#7359,.T.);
#16821=EDGE_CURVE('',#13166,#13164,#10903,.T.);
#16822=EDGE_CURVE('',#13167,#13117,#7360,.T.);
#16823=EDGE_CURVE('',#13167,#13168,#7361,.T.);
#16824=EDGE_CURVE('',#13118,#13168,#7362,.T.);
#16825=EDGE_CURVE('',#13119,#13169,#7363,.T.);
#16826=EDGE_CURVE('',#13168,#13169,#7364,.T.);
#16827=EDGE_CURVE('',#13169,#13167,#10904,.T.);
#16828=EDGE_CURVE('',#13170,#13120,#7365,.T.);
#16829=EDGE_CURVE('',#13170,#13171,#7366,.T.);
#16830=EDGE_CURVE('',#13121,#13171,#7367,.T.);
#16831=EDGE_CURVE('',#13122,#13172,#7368,.T.);
#16832=EDGE_CURVE('',#13171,#13172,#7369,.T.);
#16833=EDGE_CURVE('',#13172,#13170,#10905,.T.);
#16834=EDGE_CURVE('',#13173,#13123,#7370,.T.);
#16835=EDGE_CURVE('',#13173,#13174,#7371,.T.);
#16836=EDGE_CURVE('',#13124,#13174,#7372,.T.);
#16837=EDGE_CURVE('',#13125,#13175,#7373,.T.);
#16838=EDGE_CURVE('',#13174,#13175,#7374,.T.);
#16839=EDGE_CURVE('',#13175,#13173,#10906,.T.);
#16840=EDGE_CURVE('',#13176,#13126,#7375,.T.);
#16841=EDGE_CURVE('',#13176,#13177,#7376,.T.);
#16842=EDGE_CURVE('',#13127,#13177,#7377,.T.);
#16843=EDGE_CURVE('',#13128,#13178,#7378,.T.);
#16844=EDGE_CURVE('',#13177,#13178,#7379,.T.);
#16845=EDGE_CURVE('',#13178,#13176,#10907,.T.);
#16846=EDGE_CURVE('',#13179,#13129,#7380,.T.);
#16847=EDGE_CURVE('',#13179,#13180,#7381,.T.);
#16848=EDGE_CURVE('',#13130,#13180,#7382,.T.);
#16849=EDGE_CURVE('',#13131,#13181,#7383,.T.);
#16850=EDGE_CURVE('',#13180,#13181,#7384,.T.);
#16851=EDGE_CURVE('',#13181,#13179,#10908,.T.);
#16852=EDGE_CURVE('',#13182,#13132,#7385,.T.);
#16853=EDGE_CURVE('',#13182,#13183,#7386,.T.);
#16854=EDGE_CURVE('',#13133,#13183,#7387,.T.);
#16855=EDGE_CURVE('',#13134,#13184,#7388,.T.);
#16856=EDGE_CURVE('',#13183,#13184,#7389,.T.);
#16857=EDGE_CURVE('',#13184,#13182,#10909,.T.);
#16858=EDGE_CURVE('',#13185,#13135,#7390,.T.);
#16859=EDGE_CURVE('',#13185,#13186,#7391,.T.);
#16860=EDGE_CURVE('',#13136,#13186,#7392,.T.);
#16861=EDGE_CURVE('',#13137,#13187,#7393,.T.);
#16862=EDGE_CURVE('',#13186,#13187,#7394,.T.);
#16863=EDGE_CURVE('',#13187,#13185,#10910,.T.);
#16864=EDGE_CURVE('',#13188,#13138,#7395,.T.);
#16865=EDGE_CURVE('',#13188,#13189,#7396,.T.);
#16866=EDGE_CURVE('',#13139,#13189,#7397,.T.);
#16867=EDGE_CURVE('',#13140,#13190,#7398,.T.);
#16868=EDGE_CURVE('',#13189,#13190,#7399,.T.);
#16869=EDGE_CURVE('',#13190,#13188,#10911,.T.);
#16870=EDGE_CURVE('',#13191,#13141,#7400,.T.);
#16871=EDGE_CURVE('',#13191,#13192,#7401,.T.);
#16872=EDGE_CURVE('',#13142,#13192,#7402,.T.);
#16873=EDGE_CURVE('',#13143,#13193,#7403,.T.);
#16874=EDGE_CURVE('',#13192,#13193,#7404,.T.);
#16875=EDGE_CURVE('',#13193,#13191,#10912,.T.);
#16876=EDGE_CURVE('',#13194,#13144,#7405,.T.);
#16877=EDGE_CURVE('',#13194,#13195,#7406,.T.);
#16878=EDGE_CURVE('',#13145,#13195,#7407,.T.);
#16879=EDGE_CURVE('',#13146,#13196,#7408,.T.);
#16880=EDGE_CURVE('',#13195,#13196,#7409,.T.);
#16881=EDGE_CURVE('',#13196,#13194,#10913,.T.);
#16882=EDGE_CURVE('',#13197,#13147,#7410,.T.);
#16883=EDGE_CURVE('',#13197,#13198,#7411,.T.);
#16884=EDGE_CURVE('',#13148,#13198,#7412,.T.);
#16885=EDGE_CURVE('',#13149,#13199,#7413,.T.);
#16886=EDGE_CURVE('',#13198,#13199,#7414,.T.);
#16887=EDGE_CURVE('',#13199,#13197,#10914,.T.);
#16888=EDGE_CURVE('',#13200,#13150,#7415,.T.);
#16889=EDGE_CURVE('',#13200,#13201,#7416,.T.);
#16890=EDGE_CURVE('',#13151,#13201,#7417,.T.);
#16891=EDGE_CURVE('',#13152,#13202,#7418,.T.);
#16892=EDGE_CURVE('',#13201,#13202,#7419,.T.);
#16893=EDGE_CURVE('',#13202,#13200,#10915,.T.);
#16894=EDGE_CURVE('',#13203,#13153,#7420,.T.);
#16895=EDGE_CURVE('',#13203,#13204,#7421,.T.);
#16896=EDGE_CURVE('',#13154,#13204,#7422,.T.);
#16897=EDGE_CURVE('',#13155,#13205,#7423,.T.);
#16898=EDGE_CURVE('',#13204,#13205,#7424,.T.);
#16899=EDGE_CURVE('',#13205,#13203,#10916,.T.);
#16900=EDGE_CURVE('',#13206,#13156,#7425,.T.);
#16901=EDGE_CURVE('',#13206,#13207,#7426,.T.);
#16902=EDGE_CURVE('',#13157,#13207,#7427,.T.);
#16903=EDGE_CURVE('',#13158,#13208,#7428,.T.);
#16904=EDGE_CURVE('',#13207,#13208,#7429,.T.);
#16905=EDGE_CURVE('',#13208,#13206,#10917,.T.);
#16906=EDGE_CURVE('',#13209,#13159,#7430,.T.);
#16907=EDGE_CURVE('',#13209,#13210,#7431,.T.);
#16908=EDGE_CURVE('',#13055,#13210,#7432,.T.);
#16909=EDGE_CURVE('',#13056,#13211,#7433,.T.);
#16910=EDGE_CURVE('',#13210,#13211,#7434,.T.);
#16911=EDGE_CURVE('',#13211,#13212,#10918,.T.);
#16912=EDGE_CURVE('',#13212,#13209,#10919,.T.);
#16913=EDGE_CURVE('',#13213,#13057,#7435,.T.);
#16914=EDGE_CURVE('',#13213,#13214,#7436,.T.);
#16915=EDGE_CURVE('',#13058,#13214,#7437,.T.);
#16916=EDGE_CURVE('',#13059,#13215,#7438,.T.);
#16917=EDGE_CURVE('',#13214,#13215,#7439,.T.);
#16918=EDGE_CURVE('',#13215,#13213,#10920,.T.);
#16919=EDGE_CURVE('',#13216,#13060,#7440,.T.);
#16920=EDGE_CURVE('',#13216,#13217,#7441,.T.);
#16921=EDGE_CURVE('',#13061,#13217,#7442,.T.);
#16922=EDGE_CURVE('',#13062,#13218,#7443,.T.);
#16923=EDGE_CURVE('',#13217,#13218,#7444,.T.);
#16924=EDGE_CURVE('',#13218,#13216,#10921,.T.);
#16925=EDGE_CURVE('',#13219,#13063,#7445,.T.);
#16926=EDGE_CURVE('',#13219,#13220,#7446,.T.);
#16927=EDGE_CURVE('',#13064,#13220,#7447,.T.);
#16928=EDGE_CURVE('',#13065,#13221,#7448,.T.);
#16929=EDGE_CURVE('',#13220,#13221,#7449,.T.);
#16930=EDGE_CURVE('',#13221,#13219,#10922,.T.);
#16931=EDGE_CURVE('',#13222,#13066,#7450,.T.);
#16932=EDGE_CURVE('',#13222,#13223,#7451,.T.);
#16933=EDGE_CURVE('',#13067,#13223,#7452,.T.);
#16934=EDGE_CURVE('',#13068,#13224,#7453,.T.);
#16935=EDGE_CURVE('',#13223,#13224,#7454,.T.);
#16936=EDGE_CURVE('',#13224,#13222,#10923,.T.);
#16937=EDGE_CURVE('',#13225,#13069,#7455,.T.);
#16938=EDGE_CURVE('',#13225,#13226,#7456,.T.);
#16939=EDGE_CURVE('',#13070,#13226,#7457,.T.);
#16940=EDGE_CURVE('',#13071,#13227,#7458,.T.);
#16941=EDGE_CURVE('',#13226,#13227,#7459,.T.);
#16942=EDGE_CURVE('',#13227,#13225,#10924,.T.);
#16943=EDGE_CURVE('',#13228,#13072,#7460,.T.);
#16944=EDGE_CURVE('',#13228,#13229,#7461,.T.);
#16945=EDGE_CURVE('',#13073,#13229,#7462,.T.);
#16946=EDGE_CURVE('',#13074,#13230,#7463,.T.);
#16947=EDGE_CURVE('',#13229,#13230,#7464,.T.);
#16948=EDGE_CURVE('',#13230,#13228,#10925,.T.);
#16949=EDGE_CURVE('',#13231,#13075,#7465,.T.);
#16950=EDGE_CURVE('',#13231,#13232,#7466,.T.);
#16951=EDGE_CURVE('',#13076,#13232,#7467,.T.);
#16952=EDGE_CURVE('',#13077,#13233,#7468,.T.);
#16953=EDGE_CURVE('',#13232,#13233,#7469,.T.);
#16954=EDGE_CURVE('',#13233,#13231,#10926,.T.);
#16955=EDGE_CURVE('',#13234,#13078,#7470,.T.);
#16956=EDGE_CURVE('',#13234,#13235,#7471,.T.);
#16957=EDGE_CURVE('',#13079,#13235,#7472,.T.);
#16958=EDGE_CURVE('',#13080,#13236,#7473,.T.);
#16959=EDGE_CURVE('',#13235,#13236,#7474,.T.);
#16960=EDGE_CURVE('',#13236,#13234,#10927,.T.);
#16961=EDGE_CURVE('',#13237,#13081,#7475,.T.);
#16962=EDGE_CURVE('',#13237,#13238,#7476,.T.);
#16963=EDGE_CURVE('',#13082,#13238,#7477,.T.);
#16964=EDGE_CURVE('',#13083,#13239,#7478,.T.);
#16965=EDGE_CURVE('',#13238,#13239,#7479,.T.);
#16966=EDGE_CURVE('',#13239,#13237,#10928,.T.);
#16967=EDGE_CURVE('',#13240,#13084,#7480,.T.);
#16968=EDGE_CURVE('',#13240,#13241,#7481,.T.);
#16969=EDGE_CURVE('',#13085,#13241,#7482,.T.);
#16970=EDGE_CURVE('',#13086,#13242,#7483,.T.);
#16971=EDGE_CURVE('',#13241,#13242,#7484,.T.);
#16972=EDGE_CURVE('',#13242,#13240,#10929,.T.);
#16973=EDGE_CURVE('',#13243,#13087,#7485,.T.);
#16974=EDGE_CURVE('',#13243,#13244,#7486,.T.);
#16975=EDGE_CURVE('',#13088,#13244,#7487,.T.);
#16976=EDGE_CURVE('',#13089,#13245,#7488,.T.);
#16977=EDGE_CURVE('',#13244,#13245,#7489,.T.);
#16978=EDGE_CURVE('',#13245,#13243,#10930,.T.);
#16979=EDGE_CURVE('',#13246,#13090,#7490,.T.);
#16980=EDGE_CURVE('',#13246,#13247,#7491,.T.);
#16981=EDGE_CURVE('',#13091,#13247,#7492,.T.);
#16982=EDGE_CURVE('',#13092,#13248,#7493,.T.);
#16983=EDGE_CURVE('',#13247,#13248,#7494,.T.);
#16984=EDGE_CURVE('',#13248,#13246,#10931,.T.);
#16985=EDGE_CURVE('',#13249,#13093,#7495,.T.);
#16986=EDGE_CURVE('',#13249,#13250,#7496,.T.);
#16987=EDGE_CURVE('',#13094,#13250,#7497,.T.);
#16988=EDGE_CURVE('',#13095,#13251,#7498,.T.);
#16989=EDGE_CURVE('',#13250,#13251,#7499,.T.);
#16990=EDGE_CURVE('',#13251,#13249,#10932,.T.);
#16991=EDGE_CURVE('',#13252,#13096,#7500,.T.);
#16992=EDGE_CURVE('',#13252,#13253,#7501,.T.);
#16993=EDGE_CURVE('',#13097,#13253,#7502,.T.);
#16994=EDGE_CURVE('',#13098,#13254,#7503,.T.);
#16995=EDGE_CURVE('',#13253,#13254,#7504,.T.);
#16996=EDGE_CURVE('',#13254,#13252,#10933,.T.);
#16997=EDGE_CURVE('',#13255,#13099,#7505,.T.);
#16998=EDGE_CURVE('',#13255,#13256,#7506,.T.);
#16999=EDGE_CURVE('',#13100,#13256,#7507,.T.);
#17000=EDGE_CURVE('',#13101,#13257,#7508,.T.);
#17001=EDGE_CURVE('',#13256,#13257,#7509,.T.);
#17002=EDGE_CURVE('',#13257,#13255,#10934,.T.);
#17003=EDGE_CURVE('',#13258,#13102,#7510,.T.);
#17004=EDGE_CURVE('',#13258,#13259,#7511,.T.);
#17005=EDGE_CURVE('',#13103,#13259,#7512,.T.);
#17006=EDGE_CURVE('',#13104,#13260,#7513,.T.);
#17007=EDGE_CURVE('',#13259,#13260,#7514,.T.);
#17008=EDGE_CURVE('',#13260,#13258,#10935,.T.);
#17009=EDGE_CURVE('',#13261,#13105,#7515,.T.);
#17010=EDGE_CURVE('',#13261,#13262,#7516,.T.);
#17011=EDGE_CURVE('',#13106,#13262,#7517,.T.);
#17012=EDGE_CURVE('',#13107,#13263,#7518,.T.);
#17013=EDGE_CURVE('',#13262,#13263,#7519,.T.);
#17014=EDGE_CURVE('',#13263,#13261,#10936,.T.);
#17015=EDGE_CURVE('',#13264,#13108,#7520,.T.);
#17016=EDGE_CURVE('',#13264,#13265,#7521,.T.);
#17017=EDGE_CURVE('',#13109,#13265,#7522,.T.);
#17018=EDGE_CURVE('',#13110,#13266,#7523,.T.);
#17019=EDGE_CURVE('',#13265,#13266,#7524,.T.);
#17020=EDGE_CURVE('',#13266,#13264,#10937,.T.);
#17021=EDGE_CURVE('',#13212,#13047,#7525,.T.);
#17022=EDGE_CURVE('',#13267,#13268,#7526,.T.);
#17023=EDGE_CURVE('',#13268,#13269,#7527,.T.);
#17024=EDGE_CURVE('',#13269,#13270,#7528,.T.);
#17025=EDGE_CURVE('',#13270,#13271,#7529,.T.);
#17026=EDGE_CURVE('',#13271,#13272,#7530,.T.);
#17027=EDGE_CURVE('',#13272,#13267,#7531,.T.);
#17028=EDGE_CURVE('',#13273,#13274,#7532,.T.);
#17029=EDGE_CURVE('',#13273,#13274,#10938,.T.);
#17030=EDGE_CURVE('',#13274,#13275,#7533,.T.);
#17031=EDGE_CURVE('',#13274,#13275,#10939,.T.);
#17032=EDGE_CURVE('',#13275,#13276,#7534,.T.);
#17033=EDGE_CURVE('',#13275,#13276,#10940,.T.);
#17034=EDGE_CURVE('',#13276,#13277,#7535,.T.);
#17035=EDGE_CURVE('',#13276,#13277,#10941,.T.);
#17036=EDGE_CURVE('',#13277,#13278,#7536,.T.);
#17037=EDGE_CURVE('',#13277,#13278,#10942,.T.);
#17038=EDGE_CURVE('',#13278,#13273,#7537,.T.);
#17039=EDGE_CURVE('',#13278,#13273,#10943,.T.);
#17040=EDGE_CURVE('',#13279,#13273,#7538,.T.);
#17041=EDGE_CURVE('',#13267,#13273,#7539,.T.);
#17042=EDGE_CURVE('',#13268,#13274,#7540,.T.);
#17043=EDGE_CURVE('',#13272,#13278,#7541,.T.);
#17044=EDGE_CURVE('',#13271,#13277,#7542,.T.);
#17045=EDGE_CURVE('',#13270,#13276,#7543,.T.);
#17046=EDGE_CURVE('',#13269,#13275,#7544,.T.);
#23500=ORIENTED_EDGE('',*,*,#16611,.F.);
#23501=ORIENTED_EDGE('',*,*,#16612,.F.);
#23502=ORIENTED_EDGE('',*,*,#16613,.F.);
#23503=ORIENTED_EDGE('',*,*,#16614,.T.);
#23504=ORIENTED_EDGE('',*,*,#16615,.F.);
#23505=ORIENTED_EDGE('',*,*,#16616,.F.);
#23506=ORIENTED_EDGE('',*,*,#16617,.F.);
#23507=ORIENTED_EDGE('',*,*,#16611,.T.);
#23508=ORIENTED_EDGE('',*,*,#16618,.T.);
#23509=ORIENTED_EDGE('',*,*,#16619,.T.);
#23510=ORIENTED_EDGE('',*,*,#16620,.F.);
#23511=ORIENTED_EDGE('',*,*,#16621,.F.);
#23512=ORIENTED_EDGE('',*,*,#16622,.F.);
#23513=ORIENTED_EDGE('',*,*,#16615,.T.);
#23514=ORIENTED_EDGE('',*,*,#16623,.T.);
#23515=ORIENTED_EDGE('',*,*,#16624,.F.);
#23516=ORIENTED_EDGE('',*,*,#16625,.F.);
#23517=ORIENTED_EDGE('',*,*,#16626,.F.);
#23518=ORIENTED_EDGE('',*,*,#16620,.T.);
#23519=ORIENTED_EDGE('',*,*,#16627,.T.);
#23520=ORIENTED_EDGE('',*,*,#16628,.T.);
#23521=ORIENTED_EDGE('',*,*,#16629,.F.);
#23522=ORIENTED_EDGE('',*,*,#16630,.F.);
#23523=ORIENTED_EDGE('',*,*,#16631,.F.);
#23524=ORIENTED_EDGE('',*,*,#16624,.T.);
#23525=ORIENTED_EDGE('',*,*,#16632,.T.);
#23526=ORIENTED_EDGE('',*,*,#16633,.T.);
#23527=ORIENTED_EDGE('',*,*,#16634,.F.);
#23528=ORIENTED_EDGE('',*,*,#16635,.F.);
#23529=ORIENTED_EDGE('',*,*,#16636,.F.);
#23530=ORIENTED_EDGE('',*,*,#16629,.T.);
#23531=ORIENTED_EDGE('',*,*,#16637,.T.);
#23532=ORIENTED_EDGE('',*,*,#16638,.F.);
#23533=ORIENTED_EDGE('',*,*,#16639,.F.);
#23534=ORIENTED_EDGE('',*,*,#16634,.T.);
#23535=ORIENTED_EDGE('',*,*,#16640,.T.);
#23536=ORIENTED_EDGE('',*,*,#16641,.T.);
#23537=ORIENTED_EDGE('',*,*,#16642,.F.);
#23538=ORIENTED_EDGE('',*,*,#16643,.F.);
#23539=ORIENTED_EDGE('',*,*,#16644,.F.);
#23540=ORIENTED_EDGE('',*,*,#16638,.T.);
#23541=ORIENTED_EDGE('',*,*,#16645,.T.);
#23542=ORIENTED_EDGE('',*,*,#16646,.F.);
#23543=ORIENTED_EDGE('',*,*,#16647,.F.);
#23544=ORIENTED_EDGE('',*,*,#16642,.T.);
#23545=ORIENTED_EDGE('',*,*,#16648,.T.);
#23546=ORIENTED_EDGE('',*,*,#16649,.T.);
#23547=ORIENTED_EDGE('',*,*,#16650,.T.);
#23548=ORIENTED_EDGE('',*,*,#16651,.F.);
#23549=ORIENTED_EDGE('',*,*,#16652,.T.);
#23550=ORIENTED_EDGE('',*,*,#16653,.T.);
#23551=ORIENTED_EDGE('',*,*,#16654,.T.);
#23552=ORIENTED_EDGE('',*,*,#16655,.T.);
#23553=ORIENTED_EDGE('',*,*,#16656,.T.);
#23554=ORIENTED_EDGE('',*,*,#16657,.T.);
#23555=ORIENTED_EDGE('',*,*,#16658,.T.);
#23556=ORIENTED_EDGE('',*,*,#16659,.T.);
#23557=ORIENTED_EDGE('',*,*,#16660,.T.);
#23558=ORIENTED_EDGE('',*,*,#16661,.T.);
#23559=ORIENTED_EDGE('',*,*,#16662,.T.);
#23560=ORIENTED_EDGE('',*,*,#16663,.F.);
#23561=ORIENTED_EDGE('',*,*,#16664,.T.);
#23562=ORIENTED_EDGE('',*,*,#16665,.T.);
#23563=ORIENTED_EDGE('',*,*,#16666,.T.);
#23564=ORIENTED_EDGE('',*,*,#16667,.T.);
#23565=ORIENTED_EDGE('',*,*,#16668,.T.);
#23566=ORIENTED_EDGE('',*,*,#16669,.T.);
#23567=ORIENTED_EDGE('',*,*,#16670,.T.);
#23568=ORIENTED_EDGE('',*,*,#16671,.T.);
#23569=ORIENTED_EDGE('',*,*,#16672,.T.);
#23570=ORIENTED_EDGE('',*,*,#16673,.T.);
#23571=ORIENTED_EDGE('',*,*,#16646,.T.);
#23572=ORIENTED_EDGE('',*,*,#16674,.T.);
#23573=ORIENTED_EDGE('',*,*,#16675,.T.);
#23574=ORIENTED_EDGE('',*,*,#16676,.F.);
#23575=ORIENTED_EDGE('',*,*,#16677,.F.);
#23576=ORIENTED_EDGE('',*,*,#16678,.F.);
#23577=ORIENTED_EDGE('',*,*,#16679,.F.);
#23578=ORIENTED_EDGE('',*,*,#16680,.T.);
#23579=ORIENTED_EDGE('',*,*,#16676,.T.);
#23580=ORIENTED_EDGE('',*,*,#16681,.T.);
#23581=ORIENTED_EDGE('',*,*,#16682,.F.);
#23582=ORIENTED_EDGE('',*,*,#16680,.F.);
#23583=ORIENTED_EDGE('',*,*,#16683,.F.);
#23584=ORIENTED_EDGE('',*,*,#16662,.F.);
#23585=ORIENTED_EDGE('',*,*,#16661,.F.);
#23586=ORIENTED_EDGE('',*,*,#16660,.F.);
#23587=ORIENTED_EDGE('',*,*,#16659,.F.);
#23588=ORIENTED_EDGE('',*,*,#16658,.F.);
#23589=ORIENTED_EDGE('',*,*,#16657,.F.);
#23590=ORIENTED_EDGE('',*,*,#16656,.F.);
#23591=ORIENTED_EDGE('',*,*,#16655,.F.);
#23592=ORIENTED_EDGE('',*,*,#16654,.F.);
#23593=ORIENTED_EDGE('',*,*,#16653,.F.);
#23594=ORIENTED_EDGE('',*,*,#16652,.F.);
#23595=ORIENTED_EDGE('',*,*,#16684,.F.);
#23596=ORIENTED_EDGE('',*,*,#16612,.T.);
#23597=ORIENTED_EDGE('',*,*,#16617,.T.);
#23598=ORIENTED_EDGE('',*,*,#16616,.T.);
#23599=ORIENTED_EDGE('',*,*,#16622,.T.);
#23600=ORIENTED_EDGE('',*,*,#16621,.T.);
#23601=ORIENTED_EDGE('',*,*,#16626,.T.);
#23602=ORIENTED_EDGE('',*,*,#16625,.T.);
#23603=ORIENTED_EDGE('',*,*,#16631,.T.);
#23604=ORIENTED_EDGE('',*,*,#16630,.T.);
#23605=ORIENTED_EDGE('',*,*,#16636,.T.);
#23606=ORIENTED_EDGE('',*,*,#16635,.T.);
#23607=ORIENTED_EDGE('',*,*,#16639,.T.);
#23608=ORIENTED_EDGE('',*,*,#16644,.T.);
#23609=ORIENTED_EDGE('',*,*,#16643,.T.);
#23610=ORIENTED_EDGE('',*,*,#16647,.T.);
#23611=ORIENTED_EDGE('',*,*,#16678,.T.);
#23612=ORIENTED_EDGE('',*,*,#16677,.T.);
#23613=ORIENTED_EDGE('',*,*,#16685,.F.);
#23614=ORIENTED_EDGE('',*,*,#16686,.T.);
#23615=ORIENTED_EDGE('',*,*,#16613,.T.);
#23616=ORIENTED_EDGE('',*,*,#16684,.T.);
#23617=ORIENTED_EDGE('',*,*,#16687,.F.);
#23618=ORIENTED_EDGE('',*,*,#16681,.F.);
#23619=ORIENTED_EDGE('',*,*,#16675,.F.);
#23620=ORIENTED_EDGE('',*,*,#16674,.F.);
#23621=ORIENTED_EDGE('',*,*,#16649,.F.);
#23622=ORIENTED_EDGE('',*,*,#16648,.F.);
#23623=ORIENTED_EDGE('',*,*,#16645,.F.);
#23624=ORIENTED_EDGE('',*,*,#16641,.F.);
#23625=ORIENTED_EDGE('',*,*,#16640,.F.);
#23626=ORIENTED_EDGE('',*,*,#16637,.F.);
#23627=ORIENTED_EDGE('',*,*,#16633,.F.);
#23628=ORIENTED_EDGE('',*,*,#16632,.F.);
#23629=ORIENTED_EDGE('',*,*,#16628,.F.);
#23630=ORIENTED_EDGE('',*,*,#16627,.F.);
#23631=ORIENTED_EDGE('',*,*,#16623,.F.);
#23632=ORIENTED_EDGE('',*,*,#16619,.F.);
#23633=ORIENTED_EDGE('',*,*,#16618,.F.);
#23634=ORIENTED_EDGE('',*,*,#16614,.F.);
#23635=ORIENTED_EDGE('',*,*,#16686,.F.);
#23636=ORIENTED_EDGE('',*,*,#16688,.F.);
#23637=ORIENTED_EDGE('',*,*,#16650,.F.);
#23638=ORIENTED_EDGE('',*,*,#16673,.F.);
#23639=ORIENTED_EDGE('',*,*,#16672,.F.);
#23640=ORIENTED_EDGE('',*,*,#16671,.F.);
#23641=ORIENTED_EDGE('',*,*,#16670,.F.);
#23642=ORIENTED_EDGE('',*,*,#16669,.F.);
#23643=ORIENTED_EDGE('',*,*,#16668,.F.);
#23644=ORIENTED_EDGE('',*,*,#16667,.F.);
#23645=ORIENTED_EDGE('',*,*,#16666,.F.);
#23646=ORIENTED_EDGE('',*,*,#16665,.F.);
#23647=ORIENTED_EDGE('',*,*,#16664,.F.);
#23648=ORIENTED_EDGE('',*,*,#16689,.T.);
#23649=ORIENTED_EDGE('',*,*,#16690,.T.);
#23650=ORIENTED_EDGE('',*,*,#16687,.T.);
#23651=ORIENTED_EDGE('',*,*,#16651,.T.);
#23652=ORIENTED_EDGE('',*,*,#16688,.T.);
#23653=ORIENTED_EDGE('',*,*,#16685,.T.);
#23654=ORIENTED_EDGE('',*,*,#16690,.F.);
#23655=ORIENTED_EDGE('',*,*,#16691,.F.);
#23656=ORIENTED_EDGE('',*,*,#16689,.F.);
#23657=ORIENTED_EDGE('',*,*,#16679,.T.);
#23658=ORIENTED_EDGE('',*,*,#16692,.T.);
#23659=ORIENTED_EDGE('',*,*,#16693,.T.);
#23660=ORIENTED_EDGE('',*,*,#16692,.F.);
#23661=ORIENTED_EDGE('',*,*,#16682,.T.);
#23662=ORIENTED_EDGE('',*,*,#16663,.T.);
#23663=ORIENTED_EDGE('',*,*,#16683,.T.);
#23664=ORIENTED_EDGE('',*,*,#16693,.F.);
#23665=ORIENTED_EDGE('',*,*,#16694,.F.);
#23666=ORIENTED_EDGE('',*,*,#16695,.T.);
#23667=ORIENTED_EDGE('',*,*,#16696,.F.);
#23668=ORIENTED_EDGE('',*,*,#16697,.F.);
#23669=ORIENTED_EDGE('',*,*,#16698,.F.);
#23670=ORIENTED_EDGE('',*,*,#16699,.F.);
#23671=ORIENTED_EDGE('',*,*,#16696,.T.);
#23672=ORIENTED_EDGE('',*,*,#16700,.T.);
#23673=ORIENTED_EDGE('',*,*,#16701,.F.);
#23674=ORIENTED_EDGE('',*,*,#16700,.F.);
#23675=ORIENTED_EDGE('',*,*,#16695,.F.);
#23676=ORIENTED_EDGE('',*,*,#16702,.T.);
#23677=ORIENTED_EDGE('',*,*,#16703,.T.);
#23678=ORIENTED_EDGE('',*,*,#16704,.T.);
#23679=ORIENTED_EDGE('',*,*,#16705,.T.);
#23680=ORIENTED_EDGE('',*,*,#16706,.T.);
#23681=ORIENTED_EDGE('',*,*,#16707,.T.);
#23682=ORIENTED_EDGE('',*,*,#16708,.T.);
#23683=ORIENTED_EDGE('',*,*,#16709,.T.);
#23684=ORIENTED_EDGE('',*,*,#16710,.T.);
#23685=ORIENTED_EDGE('',*,*,#16711,.T.);
#23686=ORIENTED_EDGE('',*,*,#16712,.T.);
#23687=ORIENTED_EDGE('',*,*,#16713,.T.);
#23688=ORIENTED_EDGE('',*,*,#16714,.T.);
#23689=ORIENTED_EDGE('',*,*,#16715,.T.);
#23690=ORIENTED_EDGE('',*,*,#16716,.T.);
#23691=ORIENTED_EDGE('',*,*,#16717,.T.);
#23692=ORIENTED_EDGE('',*,*,#16718,.T.);
#23693=ORIENTED_EDGE('',*,*,#16719,.T.);
#23694=ORIENTED_EDGE('',*,*,#16720,.T.);
#23695=ORIENTED_EDGE('',*,*,#16721,.T.);
#23696=ORIENTED_EDGE('',*,*,#16722,.T.);
#23697=ORIENTED_EDGE('',*,*,#16723,.T.);
#23698=ORIENTED_EDGE('',*,*,#16724,.T.);
#23699=ORIENTED_EDGE('',*,*,#16725,.T.);
#23700=ORIENTED_EDGE('',*,*,#16726,.T.);
#23701=ORIENTED_EDGE('',*,*,#16727,.T.);
#23702=ORIENTED_EDGE('',*,*,#16728,.T.);
#23703=ORIENTED_EDGE('',*,*,#16729,.T.);
#23704=ORIENTED_EDGE('',*,*,#16730,.T.);
#23705=ORIENTED_EDGE('',*,*,#16731,.T.);
#23706=ORIENTED_EDGE('',*,*,#16732,.T.);
#23707=ORIENTED_EDGE('',*,*,#16733,.T.);
#23708=ORIENTED_EDGE('',*,*,#16734,.T.);
#23709=ORIENTED_EDGE('',*,*,#16735,.T.);
#23710=ORIENTED_EDGE('',*,*,#16736,.T.);
#23711=ORIENTED_EDGE('',*,*,#16737,.T.);
#23712=ORIENTED_EDGE('',*,*,#16738,.T.);
#23713=ORIENTED_EDGE('',*,*,#16739,.T.);
#23714=ORIENTED_EDGE('',*,*,#16740,.T.);
#23715=ORIENTED_EDGE('',*,*,#16741,.T.);
#23716=ORIENTED_EDGE('',*,*,#16742,.T.);
#23717=ORIENTED_EDGE('',*,*,#16743,.T.);
#23718=ORIENTED_EDGE('',*,*,#16744,.T.);
#23719=ORIENTED_EDGE('',*,*,#16745,.T.);
#23720=ORIENTED_EDGE('',*,*,#16746,.T.);
#23721=ORIENTED_EDGE('',*,*,#16747,.T.);
#23722=ORIENTED_EDGE('',*,*,#16748,.T.);
#23723=ORIENTED_EDGE('',*,*,#16749,.T.);
#23724=ORIENTED_EDGE('',*,*,#16750,.T.);
#23725=ORIENTED_EDGE('',*,*,#16751,.T.);
#23726=ORIENTED_EDGE('',*,*,#16752,.T.);
#23727=ORIENTED_EDGE('',*,*,#16753,.T.);
#23728=ORIENTED_EDGE('',*,*,#16754,.T.);
#23729=ORIENTED_EDGE('',*,*,#16755,.T.);
#23730=ORIENTED_EDGE('',*,*,#16756,.T.);
#23731=ORIENTED_EDGE('',*,*,#16757,.T.);
#23732=ORIENTED_EDGE('',*,*,#16697,.T.);
#23733=ORIENTED_EDGE('',*,*,#16699,.T.);
#23734=ORIENTED_EDGE('',*,*,#16758,.T.);
#23735=ORIENTED_EDGE('',*,*,#16759,.T.);
#23736=ORIENTED_EDGE('',*,*,#16760,.T.);
#23737=ORIENTED_EDGE('',*,*,#16761,.T.);
#23738=ORIENTED_EDGE('',*,*,#16762,.T.);
#23739=ORIENTED_EDGE('',*,*,#16763,.T.);
#23740=ORIENTED_EDGE('',*,*,#16764,.T.);
#23741=ORIENTED_EDGE('',*,*,#16765,.T.);
#23742=ORIENTED_EDGE('',*,*,#16766,.T.);
#23743=ORIENTED_EDGE('',*,*,#16767,.T.);
#23744=ORIENTED_EDGE('',*,*,#16768,.T.);
#23745=ORIENTED_EDGE('',*,*,#16769,.T.);
#23746=ORIENTED_EDGE('',*,*,#16770,.T.);
#23747=ORIENTED_EDGE('',*,*,#16771,.T.);
#23748=ORIENTED_EDGE('',*,*,#16772,.T.);
#23749=ORIENTED_EDGE('',*,*,#16773,.T.);
#23750=ORIENTED_EDGE('',*,*,#16774,.T.);
#23751=ORIENTED_EDGE('',*,*,#16775,.T.);
#23752=ORIENTED_EDGE('',*,*,#16776,.T.);
#23753=ORIENTED_EDGE('',*,*,#16777,.T.);
#23754=ORIENTED_EDGE('',*,*,#16778,.T.);
#23755=ORIENTED_EDGE('',*,*,#16779,.T.);
#23756=ORIENTED_EDGE('',*,*,#16780,.T.);
#23757=ORIENTED_EDGE('',*,*,#16781,.T.);
#23758=ORIENTED_EDGE('',*,*,#16782,.T.);
#23759=ORIENTED_EDGE('',*,*,#16783,.T.);
#23760=ORIENTED_EDGE('',*,*,#16784,.T.);
#23761=ORIENTED_EDGE('',*,*,#16785,.T.);
#23762=ORIENTED_EDGE('',*,*,#16786,.T.);
#23763=ORIENTED_EDGE('',*,*,#16787,.T.);
#23764=ORIENTED_EDGE('',*,*,#16788,.T.);
#23765=ORIENTED_EDGE('',*,*,#16789,.T.);
#23766=ORIENTED_EDGE('',*,*,#16790,.T.);
#23767=ORIENTED_EDGE('',*,*,#16791,.T.);
#23768=ORIENTED_EDGE('',*,*,#16792,.T.);
#23769=ORIENTED_EDGE('',*,*,#16793,.T.);
#23770=ORIENTED_EDGE('',*,*,#16794,.T.);
#23771=ORIENTED_EDGE('',*,*,#16795,.T.);
#23772=ORIENTED_EDGE('',*,*,#16796,.T.);
#23773=ORIENTED_EDGE('',*,*,#16797,.T.);
#23774=ORIENTED_EDGE('',*,*,#16798,.T.);
#23775=ORIENTED_EDGE('',*,*,#16799,.T.);
#23776=ORIENTED_EDGE('',*,*,#16800,.T.);
#23777=ORIENTED_EDGE('',*,*,#16801,.T.);
#23778=ORIENTED_EDGE('',*,*,#16802,.T.);
#23779=ORIENTED_EDGE('',*,*,#16803,.T.);
#23780=ORIENTED_EDGE('',*,*,#16804,.T.);
#23781=ORIENTED_EDGE('',*,*,#16805,.T.);
#23782=ORIENTED_EDGE('',*,*,#16806,.T.);
#23783=ORIENTED_EDGE('',*,*,#16807,.T.);
#23784=ORIENTED_EDGE('',*,*,#16808,.T.);
#23785=ORIENTED_EDGE('',*,*,#16809,.T.);
#23786=ORIENTED_EDGE('',*,*,#16808,.F.);
#23787=ORIENTED_EDGE('',*,*,#16810,.F.);
#23788=ORIENTED_EDGE('',*,*,#16811,.T.);
#23789=ORIENTED_EDGE('',*,*,#16812,.F.);
#23790=ORIENTED_EDGE('',*,*,#16759,.F.);
#23791=ORIENTED_EDGE('',*,*,#16813,.F.);
#23792=ORIENTED_EDGE('',*,*,#16760,.F.);
#23793=ORIENTED_EDGE('',*,*,#16812,.T.);
#23794=ORIENTED_EDGE('',*,*,#16814,.T.);
#23795=ORIENTED_EDGE('',*,*,#16815,.F.);
#23796=ORIENTED_EDGE('',*,*,#16814,.F.);
#23797=ORIENTED_EDGE('',*,*,#16811,.F.);
#23798=ORIENTED_EDGE('',*,*,#16816,.F.);
#23799=ORIENTED_EDGE('',*,*,#16817,.T.);
#23800=ORIENTED_EDGE('',*,*,#16818,.F.);
#23801=ORIENTED_EDGE('',*,*,#16762,.F.);
#23802=ORIENTED_EDGE('',*,*,#16819,.F.);
#23803=ORIENTED_EDGE('',*,*,#16763,.F.);
#23804=ORIENTED_EDGE('',*,*,#16818,.T.);
#23805=ORIENTED_EDGE('',*,*,#16820,.T.);
#23806=ORIENTED_EDGE('',*,*,#16821,.F.);
#23807=ORIENTED_EDGE('',*,*,#16820,.F.);
#23808=ORIENTED_EDGE('',*,*,#16817,.F.);
#23809=ORIENTED_EDGE('',*,*,#16822,.F.);
#23810=ORIENTED_EDGE('',*,*,#16823,.T.);
#23811=ORIENTED_EDGE('',*,*,#16824,.F.);
#23812=ORIENTED_EDGE('',*,*,#16765,.F.);
#23813=ORIENTED_EDGE('',*,*,#16825,.F.);
#23814=ORIENTED_EDGE('',*,*,#16766,.F.);
#23815=ORIENTED_EDGE('',*,*,#16824,.T.);
#23816=ORIENTED_EDGE('',*,*,#16826,.T.);
#23817=ORIENTED_EDGE('',*,*,#16827,.F.);
#23818=ORIENTED_EDGE('',*,*,#16826,.F.);
#23819=ORIENTED_EDGE('',*,*,#16823,.F.);
#23820=ORIENTED_EDGE('',*,*,#16828,.F.);
#23821=ORIENTED_EDGE('',*,*,#16829,.T.);
#23822=ORIENTED_EDGE('',*,*,#16830,.F.);
#23823=ORIENTED_EDGE('',*,*,#16768,.F.);
#23824=ORIENTED_EDGE('',*,*,#16831,.F.);
#23825=ORIENTED_EDGE('',*,*,#16769,.F.);
#23826=ORIENTED_EDGE('',*,*,#16830,.T.);
#23827=ORIENTED_EDGE('',*,*,#16832,.T.);
#23828=ORIENTED_EDGE('',*,*,#16833,.F.);
#23829=ORIENTED_EDGE('',*,*,#16832,.F.);
#23830=ORIENTED_EDGE('',*,*,#16829,.F.);
#23831=ORIENTED_EDGE('',*,*,#16834,.F.);
#23832=ORIENTED_EDGE('',*,*,#16835,.T.);
#23833=ORIENTED_EDGE('',*,*,#16836,.F.);
#23834=ORIENTED_EDGE('',*,*,#16771,.F.);
#23835=ORIENTED_EDGE('',*,*,#16837,.F.);
#23836=ORIENTED_EDGE('',*,*,#16772,.F.);
#23837=ORIENTED_EDGE('',*,*,#16836,.T.);
#23838=ORIENTED_EDGE('',*,*,#16838,.T.);
#23839=ORIENTED_EDGE('',*,*,#16839,.F.);
#23840=ORIENTED_EDGE('',*,*,#16838,.F.);
#23841=ORIENTED_EDGE('',*,*,#16835,.F.);
#23842=ORIENTED_EDGE('',*,*,#16840,.F.);
#23843=ORIENTED_EDGE('',*,*,#16841,.T.);
#23844=ORIENTED_EDGE('',*,*,#16842,.F.);
#23845=ORIENTED_EDGE('',*,*,#16774,.F.);
#23846=ORIENTED_EDGE('',*,*,#16843,.F.);
#23847=ORIENTED_EDGE('',*,*,#16775,.F.);
#23848=ORIENTED_EDGE('',*,*,#16842,.T.);
#23849=ORIENTED_EDGE('',*,*,#16844,.T.);
#23850=ORIENTED_EDGE('',*,*,#16845,.F.);
#23851=ORIENTED_EDGE('',*,*,#16844,.F.);
#23852=ORIENTED_EDGE('',*,*,#16841,.F.);
#23853=ORIENTED_EDGE('',*,*,#16846,.F.);
#23854=ORIENTED_EDGE('',*,*,#16847,.T.);
#23855=ORIENTED_EDGE('',*,*,#16848,.F.);
#23856=ORIENTED_EDGE('',*,*,#16777,.F.);
#23857=ORIENTED_EDGE('',*,*,#16849,.F.);
#23858=ORIENTED_EDGE('',*,*,#16778,.F.);
#23859=ORIENTED_EDGE('',*,*,#16848,.T.);
#23860=ORIENTED_EDGE('',*,*,#16850,.T.);
#23861=ORIENTED_EDGE('',*,*,#16851,.F.);
#23862=ORIENTED_EDGE('',*,*,#16850,.F.);
#23863=ORIENTED_EDGE('',*,*,#16847,.F.);
#23864=ORIENTED_EDGE('',*,*,#16852,.F.);
#23865=ORIENTED_EDGE('',*,*,#16853,.T.);
#23866=ORIENTED_EDGE('',*,*,#16854,.F.);
#23867=ORIENTED_EDGE('',*,*,#16780,.F.);
#23868=ORIENTED_EDGE('',*,*,#16855,.F.);
#23869=ORIENTED_EDGE('',*,*,#16781,.F.);
#23870=ORIENTED_EDGE('',*,*,#16854,.T.);
#23871=ORIENTED_EDGE('',*,*,#16856,.T.);
#23872=ORIENTED_EDGE('',*,*,#16857,.F.);
#23873=ORIENTED_EDGE('',*,*,#16856,.F.);
#23874=ORIENTED_EDGE('',*,*,#16853,.F.);
#23875=ORIENTED_EDGE('',*,*,#16858,.F.);
#23876=ORIENTED_EDGE('',*,*,#16859,.T.);
#23877=ORIENTED_EDGE('',*,*,#16860,.F.);
#23878=ORIENTED_EDGE('',*,*,#16783,.F.);
#23879=ORIENTED_EDGE('',*,*,#16861,.F.);
#23880=ORIENTED_EDGE('',*,*,#16784,.F.);
#23881=ORIENTED_EDGE('',*,*,#16860,.T.);
#23882=ORIENTED_EDGE('',*,*,#16862,.T.);
#23883=ORIENTED_EDGE('',*,*,#16863,.F.);
#23884=ORIENTED_EDGE('',*,*,#16862,.F.);
#23885=ORIENTED_EDGE('',*,*,#16859,.F.);
#23886=ORIENTED_EDGE('',*,*,#16864,.F.);
#23887=ORIENTED_EDGE('',*,*,#16865,.T.);
#23888=ORIENTED_EDGE('',*,*,#16866,.F.);
#23889=ORIENTED_EDGE('',*,*,#16786,.F.);
#23890=ORIENTED_EDGE('',*,*,#16867,.F.);
#23891=ORIENTED_EDGE('',*,*,#16787,.F.);
#23892=ORIENTED_EDGE('',*,*,#16866,.T.);
#23893=ORIENTED_EDGE('',*,*,#16868,.T.);
#23894=ORIENTED_EDGE('',*,*,#16869,.F.);
#23895=ORIENTED_EDGE('',*,*,#16868,.F.);
#23896=ORIENTED_EDGE('',*,*,#16865,.F.);
#23897=ORIENTED_EDGE('',*,*,#16870,.F.);
#23898=ORIENTED_EDGE('',*,*,#16871,.T.);
#23899=ORIENTED_EDGE('',*,*,#16872,.F.);
#23900=ORIENTED_EDGE('',*,*,#16789,.F.);
#23901=ORIENTED_EDGE('',*,*,#16873,.F.);
#23902=ORIENTED_EDGE('',*,*,#16790,.F.);
#23903=ORIENTED_EDGE('',*,*,#16872,.T.);
#23904=ORIENTED_EDGE('',*,*,#16874,.T.);
#23905=ORIENTED_EDGE('',*,*,#16875,.F.);
#23906=ORIENTED_EDGE('',*,*,#16874,.F.);
#23907=ORIENTED_EDGE('',*,*,#16871,.F.);
#23908=ORIENTED_EDGE('',*,*,#16876,.F.);
#23909=ORIENTED_EDGE('',*,*,#16877,.T.);
#23910=ORIENTED_EDGE('',*,*,#16878,.F.);
#23911=ORIENTED_EDGE('',*,*,#16792,.F.);
#23912=ORIENTED_EDGE('',*,*,#16879,.F.);
#23913=ORIENTED_EDGE('',*,*,#16793,.F.);
#23914=ORIENTED_EDGE('',*,*,#16878,.T.);
#23915=ORIENTED_EDGE('',*,*,#16880,.T.);
#23916=ORIENTED_EDGE('',*,*,#16881,.F.);
#23917=ORIENTED_EDGE('',*,*,#16880,.F.);
#23918=ORIENTED_EDGE('',*,*,#16877,.F.);
#23919=ORIENTED_EDGE('',*,*,#16882,.F.);
#23920=ORIENTED_EDGE('',*,*,#16883,.T.);
#23921=ORIENTED_EDGE('',*,*,#16884,.F.);
#23922=ORIENTED_EDGE('',*,*,#16795,.F.);
#23923=ORIENTED_EDGE('',*,*,#16885,.F.);
#23924=ORIENTED_EDGE('',*,*,#16796,.F.);
#23925=ORIENTED_EDGE('',*,*,#16884,.T.);
#23926=ORIENTED_EDGE('',*,*,#16886,.T.);
#23927=ORIENTED_EDGE('',*,*,#16887,.F.);
#23928=ORIENTED_EDGE('',*,*,#16886,.F.);
#23929=ORIENTED_EDGE('',*,*,#16883,.F.);
#23930=ORIENTED_EDGE('',*,*,#16888,.F.);
#23931=ORIENTED_EDGE('',*,*,#16889,.T.);
#23932=ORIENTED_EDGE('',*,*,#16890,.F.);
#23933=ORIENTED_EDGE('',*,*,#16798,.F.);
#23934=ORIENTED_EDGE('',*,*,#16891,.F.);
#23935=ORIENTED_EDGE('',*,*,#16799,.F.);
#23936=ORIENTED_EDGE('',*,*,#16890,.T.);
#23937=ORIENTED_EDGE('',*,*,#16892,.T.);
#23938=ORIENTED_EDGE('',*,*,#16893,.F.);
#23939=ORIENTED_EDGE('',*,*,#16892,.F.);
#23940=ORIENTED_EDGE('',*,*,#16889,.F.);
#23941=ORIENTED_EDGE('',*,*,#16894,.F.);
#23942=ORIENTED_EDGE('',*,*,#16895,.T.);
#23943=ORIENTED_EDGE('',*,*,#16896,.F.);
#23944=ORIENTED_EDGE('',*,*,#16801,.F.);
#23945=ORIENTED_EDGE('',*,*,#16897,.F.);
#23946=ORIENTED_EDGE('',*,*,#16802,.F.);
#23947=ORIENTED_EDGE('',*,*,#16896,.T.);
#23948=ORIENTED_EDGE('',*,*,#16898,.T.);
#23949=ORIENTED_EDGE('',*,*,#16899,.F.);
#23950=ORIENTED_EDGE('',*,*,#16898,.F.);
#23951=ORIENTED_EDGE('',*,*,#16895,.F.);
#23952=ORIENTED_EDGE('',*,*,#16900,.F.);
#23953=ORIENTED_EDGE('',*,*,#16901,.T.);
#23954=ORIENTED_EDGE('',*,*,#16902,.F.);
#23955=ORIENTED_EDGE('',*,*,#16804,.F.);
#23956=ORIENTED_EDGE('',*,*,#16903,.F.);
#23957=ORIENTED_EDGE('',*,*,#16805,.F.);
#23958=ORIENTED_EDGE('',*,*,#16902,.T.);
#23959=ORIENTED_EDGE('',*,*,#16904,.T.);
#23960=ORIENTED_EDGE('',*,*,#16905,.F.);
#23961=ORIENTED_EDGE('',*,*,#16904,.F.);
#23962=ORIENTED_EDGE('',*,*,#16901,.F.);
#23963=ORIENTED_EDGE('',*,*,#16906,.F.);
#23964=ORIENTED_EDGE('',*,*,#16907,.T.);
#23965=ORIENTED_EDGE('',*,*,#16908,.F.);
#23966=ORIENTED_EDGE('',*,*,#16807,.F.);
#23967=ORIENTED_EDGE('',*,*,#16909,.F.);
#23968=ORIENTED_EDGE('',*,*,#16702,.F.);
#23969=ORIENTED_EDGE('',*,*,#16908,.T.);
#23970=ORIENTED_EDGE('',*,*,#16910,.T.);
#23971=ORIENTED_EDGE('',*,*,#16911,.F.);
#23972=ORIENTED_EDGE('',*,*,#16910,.F.);
#23973=ORIENTED_EDGE('',*,*,#16907,.F.);
#23974=ORIENTED_EDGE('',*,*,#16912,.F.);
#23975=ORIENTED_EDGE('',*,*,#16913,.F.);
#23976=ORIENTED_EDGE('',*,*,#16914,.T.);
#23977=ORIENTED_EDGE('',*,*,#16915,.F.);
#23978=ORIENTED_EDGE('',*,*,#16704,.F.);
#23979=ORIENTED_EDGE('',*,*,#16916,.F.);
#23980=ORIENTED_EDGE('',*,*,#16705,.F.);
#23981=ORIENTED_EDGE('',*,*,#16915,.T.);
#23982=ORIENTED_EDGE('',*,*,#16917,.T.);
#23983=ORIENTED_EDGE('',*,*,#16918,.F.);
#23984=ORIENTED_EDGE('',*,*,#16917,.F.);
#23985=ORIENTED_EDGE('',*,*,#16914,.F.);
#23986=ORIENTED_EDGE('',*,*,#16919,.F.);
#23987=ORIENTED_EDGE('',*,*,#16920,.T.);
#23988=ORIENTED_EDGE('',*,*,#16921,.F.);
#23989=ORIENTED_EDGE('',*,*,#16707,.F.);
#23990=ORIENTED_EDGE('',*,*,#16922,.F.);
#23991=ORIENTED_EDGE('',*,*,#16708,.F.);
#23992=ORIENTED_EDGE('',*,*,#16921,.T.);
#23993=ORIENTED_EDGE('',*,*,#16923,.T.);
#23994=ORIENTED_EDGE('',*,*,#16924,.F.);
#23995=ORIENTED_EDGE('',*,*,#16923,.F.);
#23996=ORIENTED_EDGE('',*,*,#16920,.F.);
#23997=ORIENTED_EDGE('',*,*,#16925,.F.);
#23998=ORIENTED_EDGE('',*,*,#16926,.T.);
#23999=ORIENTED_EDGE('',*,*,#16927,.F.);
#24000=ORIENTED_EDGE('',*,*,#16710,.F.);
#24001=ORIENTED_EDGE('',*,*,#16928,.F.);
#24002=ORIENTED_EDGE('',*,*,#16711,.F.);
#24003=ORIENTED_EDGE('',*,*,#16927,.T.);
#24004=ORIENTED_EDGE('',*,*,#16929,.T.);
#24005=ORIENTED_EDGE('',*,*,#16930,.F.);
#24006=ORIENTED_EDGE('',*,*,#16929,.F.);
#24007=ORIENTED_EDGE('',*,*,#16926,.F.);
#24008=ORIENTED_EDGE('',*,*,#16931,.F.);
#24009=ORIENTED_EDGE('',*,*,#16932,.T.);
#24010=ORIENTED_EDGE('',*,*,#16933,.F.);
#24011=ORIENTED_EDGE('',*,*,#16713,.F.);
#24012=ORIENTED_EDGE('',*,*,#16934,.F.);
#24013=ORIENTED_EDGE('',*,*,#16714,.F.);
#24014=ORIENTED_EDGE('',*,*,#16933,.T.);
#24015=ORIENTED_EDGE('',*,*,#16935,.T.);
#24016=ORIENTED_EDGE('',*,*,#16936,.F.);
#24017=ORIENTED_EDGE('',*,*,#16935,.F.);
#24018=ORIENTED_EDGE('',*,*,#16932,.F.);
#24019=ORIENTED_EDGE('',*,*,#16937,.F.);
#24020=ORIENTED_EDGE('',*,*,#16938,.T.);
#24021=ORIENTED_EDGE('',*,*,#16939,.F.);
#24022=ORIENTED_EDGE('',*,*,#16716,.F.);
#24023=ORIENTED_EDGE('',*,*,#16940,.F.);
#24024=ORIENTED_EDGE('',*,*,#16717,.F.);
#24025=ORIENTED_EDGE('',*,*,#16939,.T.);
#24026=ORIENTED_EDGE('',*,*,#16941,.T.);
#24027=ORIENTED_EDGE('',*,*,#16942,.F.);
#24028=ORIENTED_EDGE('',*,*,#16941,.F.);
#24029=ORIENTED_EDGE('',*,*,#16938,.F.);
#24030=ORIENTED_EDGE('',*,*,#16943,.F.);
#24031=ORIENTED_EDGE('',*,*,#16944,.T.);
#24032=ORIENTED_EDGE('',*,*,#16945,.F.);
#24033=ORIENTED_EDGE('',*,*,#16719,.F.);
#24034=ORIENTED_EDGE('',*,*,#16946,.F.);
#24035=ORIENTED_EDGE('',*,*,#16720,.F.);
#24036=ORIENTED_EDGE('',*,*,#16945,.T.);
#24037=ORIENTED_EDGE('',*,*,#16947,.T.);
#24038=ORIENTED_EDGE('',*,*,#16948,.F.);
#24039=ORIENTED_EDGE('',*,*,#16947,.F.);
#24040=ORIENTED_EDGE('',*,*,#16944,.F.);
#24041=ORIENTED_EDGE('',*,*,#16949,.F.);
#24042=ORIENTED_EDGE('',*,*,#16950,.T.);
#24043=ORIENTED_EDGE('',*,*,#16951,.F.);
#24044=ORIENTED_EDGE('',*,*,#16722,.F.);
#24045=ORIENTED_EDGE('',*,*,#16952,.F.);
#24046=ORIENTED_EDGE('',*,*,#16723,.F.);
#24047=ORIENTED_EDGE('',*,*,#16951,.T.);
#24048=ORIENTED_EDGE('',*,*,#16953,.T.);
#24049=ORIENTED_EDGE('',*,*,#16954,.F.);
#24050=ORIENTED_EDGE('',*,*,#16953,.F.);
#24051=ORIENTED_EDGE('',*,*,#16950,.F.);
#24052=ORIENTED_EDGE('',*,*,#16955,.F.);
#24053=ORIENTED_EDGE('',*,*,#16956,.T.);
#24054=ORIENTED_EDGE('',*,*,#16957,.F.);
#24055=ORIENTED_EDGE('',*,*,#16725,.F.);
#24056=ORIENTED_EDGE('',*,*,#16958,.F.);
#24057=ORIENTED_EDGE('',*,*,#16726,.F.);
#24058=ORIENTED_EDGE('',*,*,#16957,.T.);
#24059=ORIENTED_EDGE('',*,*,#16959,.T.);
#24060=ORIENTED_EDGE('',*,*,#16960,.F.);
#24061=ORIENTED_EDGE('',*,*,#16959,.F.);
#24062=ORIENTED_EDGE('',*,*,#16956,.F.);
#24063=ORIENTED_EDGE('',*,*,#16961,.F.);
#24064=ORIENTED_EDGE('',*,*,#16962,.T.);
#24065=ORIENTED_EDGE('',*,*,#16963,.F.);
#24066=ORIENTED_EDGE('',*,*,#16728,.F.);
#24067=ORIENTED_EDGE('',*,*,#16964,.F.);
#24068=ORIENTED_EDGE('',*,*,#16729,.F.);
#24069=ORIENTED_EDGE('',*,*,#16963,.T.);
#24070=ORIENTED_EDGE('',*,*,#16965,.T.);
#24071=ORIENTED_EDGE('',*,*,#16966,.F.);
#24072=ORIENTED_EDGE('',*,*,#16965,.F.);
#24073=ORIENTED_EDGE('',*,*,#16962,.F.);
#24074=ORIENTED_EDGE('',*,*,#16967,.F.);
#24075=ORIENTED_EDGE('',*,*,#16968,.T.);
#24076=ORIENTED_EDGE('',*,*,#16969,.F.);
#24077=ORIENTED_EDGE('',*,*,#16731,.F.);
#24078=ORIENTED_EDGE('',*,*,#16970,.F.);
#24079=ORIENTED_EDGE('',*,*,#16732,.F.);
#24080=ORIENTED_EDGE('',*,*,#16969,.T.);
#24081=ORIENTED_EDGE('',*,*,#16971,.T.);
#24082=ORIENTED_EDGE('',*,*,#16972,.F.);
#24083=ORIENTED_EDGE('',*,*,#16971,.F.);
#24084=ORIENTED_EDGE('',*,*,#16968,.F.);
#24085=ORIENTED_EDGE('',*,*,#16973,.F.);
#24086=ORIENTED_EDGE('',*,*,#16974,.T.);
#24087=ORIENTED_EDGE('',*,*,#16975,.F.);
#24088=ORIENTED_EDGE('',*,*,#16734,.F.);
#24089=ORIENTED_EDGE('',*,*,#16976,.F.);
#24090=ORIENTED_EDGE('',*,*,#16735,.F.);
#24091=ORIENTED_EDGE('',*,*,#16975,.T.);
#24092=ORIENTED_EDGE('',*,*,#16977,.T.);
#24093=ORIENTED_EDGE('',*,*,#16978,.F.);
#24094=ORIENTED_EDGE('',*,*,#16977,.F.);
#24095=ORIENTED_EDGE('',*,*,#16974,.F.);
#24096=ORIENTED_EDGE('',*,*,#16979,.F.);
#24097=ORIENTED_EDGE('',*,*,#16980,.T.);
#24098=ORIENTED_EDGE('',*,*,#16981,.F.);
#24099=ORIENTED_EDGE('',*,*,#16737,.F.);
#24100=ORIENTED_EDGE('',*,*,#16982,.F.);
#24101=ORIENTED_EDGE('',*,*,#16738,.F.);
#24102=ORIENTED_EDGE('',*,*,#16981,.T.);
#24103=ORIENTED_EDGE('',*,*,#16983,.T.);
#24104=ORIENTED_EDGE('',*,*,#16984,.F.);
#24105=ORIENTED_EDGE('',*,*,#16983,.F.);
#24106=ORIENTED_EDGE('',*,*,#16980,.F.);
#24107=ORIENTED_EDGE('',*,*,#16985,.F.);
#24108=ORIENTED_EDGE('',*,*,#16986,.T.);
#24109=ORIENTED_EDGE('',*,*,#16987,.F.);
#24110=ORIENTED_EDGE('',*,*,#16740,.F.);
#24111=ORIENTED_EDGE('',*,*,#16988,.F.);
#24112=ORIENTED_EDGE('',*,*,#16741,.F.);
#24113=ORIENTED_EDGE('',*,*,#16987,.T.);
#24114=ORIENTED_EDGE('',*,*,#16989,.T.);
#24115=ORIENTED_EDGE('',*,*,#16990,.F.);
#24116=ORIENTED_EDGE('',*,*,#16989,.F.);
#24117=ORIENTED_EDGE('',*,*,#16986,.F.);
#24118=ORIENTED_EDGE('',*,*,#16991,.F.);
#24119=ORIENTED_EDGE('',*,*,#16992,.T.);
#24120=ORIENTED_EDGE('',*,*,#16993,.F.);
#24121=ORIENTED_EDGE('',*,*,#16743,.F.);
#24122=ORIENTED_EDGE('',*,*,#16994,.F.);
#24123=ORIENTED_EDGE('',*,*,#16744,.F.);
#24124=ORIENTED_EDGE('',*,*,#16993,.T.);
#24125=ORIENTED_EDGE('',*,*,#16995,.T.);
#24126=ORIENTED_EDGE('',*,*,#16996,.F.);
#24127=ORIENTED_EDGE('',*,*,#16995,.F.);
#24128=ORIENTED_EDGE('',*,*,#16992,.F.);
#24129=ORIENTED_EDGE('',*,*,#16997,.F.);
#24130=ORIENTED_EDGE('',*,*,#16998,.T.);
#24131=ORIENTED_EDGE('',*,*,#16999,.F.);
#24132=ORIENTED_EDGE('',*,*,#16746,.F.);
#24133=ORIENTED_EDGE('',*,*,#17000,.F.);
#24134=ORIENTED_EDGE('',*,*,#16747,.F.);
#24135=ORIENTED_EDGE('',*,*,#16999,.T.);
#24136=ORIENTED_EDGE('',*,*,#17001,.T.);
#24137=ORIENTED_EDGE('',*,*,#17002,.F.);
#24138=ORIENTED_EDGE('',*,*,#17001,.F.);
#24139=ORIENTED_EDGE('',*,*,#16998,.F.);
#24140=ORIENTED_EDGE('',*,*,#17003,.F.);
#24141=ORIENTED_EDGE('',*,*,#17004,.T.);
#24142=ORIENTED_EDGE('',*,*,#17005,.F.);
#24143=ORIENTED_EDGE('',*,*,#16749,.F.);
#24144=ORIENTED_EDGE('',*,*,#17006,.F.);
#24145=ORIENTED_EDGE('',*,*,#16750,.F.);
#24146=ORIENTED_EDGE('',*,*,#17005,.T.);
#24147=ORIENTED_EDGE('',*,*,#17007,.T.);
#24148=ORIENTED_EDGE('',*,*,#17008,.F.);
#24149=ORIENTED_EDGE('',*,*,#17007,.F.);
#24150=ORIENTED_EDGE('',*,*,#17004,.F.);
#24151=ORIENTED_EDGE('',*,*,#17009,.F.);
#24152=ORIENTED_EDGE('',*,*,#17010,.T.);
#24153=ORIENTED_EDGE('',*,*,#17011,.F.);
#24154=ORIENTED_EDGE('',*,*,#16752,.F.);
#24155=ORIENTED_EDGE('',*,*,#17012,.F.);
#24156=ORIENTED_EDGE('',*,*,#16753,.F.);
#24157=ORIENTED_EDGE('',*,*,#17011,.T.);
#24158=ORIENTED_EDGE('',*,*,#17013,.T.);
#24159=ORIENTED_EDGE('',*,*,#17014,.F.);
#24160=ORIENTED_EDGE('',*,*,#17013,.F.);
#24161=ORIENTED_EDGE('',*,*,#17010,.F.);
#24162=ORIENTED_EDGE('',*,*,#17015,.F.);
#24163=ORIENTED_EDGE('',*,*,#17016,.T.);
#24164=ORIENTED_EDGE('',*,*,#17017,.F.);
#24165=ORIENTED_EDGE('',*,*,#16755,.F.);
#24166=ORIENTED_EDGE('',*,*,#17018,.F.);
#24167=ORIENTED_EDGE('',*,*,#16756,.F.);
#24168=ORIENTED_EDGE('',*,*,#17017,.T.);
#24169=ORIENTED_EDGE('',*,*,#17019,.T.);
#24170=ORIENTED_EDGE('',*,*,#17020,.F.);
#24171=ORIENTED_EDGE('',*,*,#17019,.F.);
#24172=ORIENTED_EDGE('',*,*,#17016,.F.);
#24173=ORIENTED_EDGE('',*,*,#16911,.T.);
#24174=ORIENTED_EDGE('',*,*,#17021,.T.);
#24175=ORIENTED_EDGE('',*,*,#16691,.T.);
#24176=ORIENTED_EDGE('',*,*,#17021,.F.);
#24177=ORIENTED_EDGE('',*,*,#16912,.T.);
#24178=ORIENTED_EDGE('',*,*,#16906,.T.);
#24179=ORIENTED_EDGE('',*,*,#16806,.F.);
#24180=ORIENTED_EDGE('',*,*,#16903,.T.);
#24181=ORIENTED_EDGE('',*,*,#16905,.T.);
#24182=ORIENTED_EDGE('',*,*,#16900,.T.);
#24183=ORIENTED_EDGE('',*,*,#16803,.F.);
#24184=ORIENTED_EDGE('',*,*,#16897,.T.);
#24185=ORIENTED_EDGE('',*,*,#16899,.T.);
#24186=ORIENTED_EDGE('',*,*,#16894,.T.);
#24187=ORIENTED_EDGE('',*,*,#16800,.F.);
#24188=ORIENTED_EDGE('',*,*,#16891,.T.);
#24189=ORIENTED_EDGE('',*,*,#16893,.T.);
#24190=ORIENTED_EDGE('',*,*,#16888,.T.);
#24191=ORIENTED_EDGE('',*,*,#16797,.F.);
#24192=ORIENTED_EDGE('',*,*,#16885,.T.);
#24193=ORIENTED_EDGE('',*,*,#16887,.T.);
#24194=ORIENTED_EDGE('',*,*,#16882,.T.);
#24195=ORIENTED_EDGE('',*,*,#16794,.F.);
#24196=ORIENTED_EDGE('',*,*,#16879,.T.);
#24197=ORIENTED_EDGE('',*,*,#16881,.T.);
#24198=ORIENTED_EDGE('',*,*,#16876,.T.);
#24199=ORIENTED_EDGE('',*,*,#16791,.F.);
#24200=ORIENTED_EDGE('',*,*,#16873,.T.);
#24201=ORIENTED_EDGE('',*,*,#16875,.T.);
#24202=ORIENTED_EDGE('',*,*,#16870,.T.);
#24203=ORIENTED_EDGE('',*,*,#16788,.F.);
#24204=ORIENTED_EDGE('',*,*,#16867,.T.);
#24205=ORIENTED_EDGE('',*,*,#16869,.T.);
#24206=ORIENTED_EDGE('',*,*,#16864,.T.);
#24207=ORIENTED_EDGE('',*,*,#16785,.F.);
#24208=ORIENTED_EDGE('',*,*,#16861,.T.);
#24209=ORIENTED_EDGE('',*,*,#16863,.T.);
#24210=ORIENTED_EDGE('',*,*,#16858,.T.);
#24211=ORIENTED_EDGE('',*,*,#16782,.F.);
#24212=ORIENTED_EDGE('',*,*,#16855,.T.);
#24213=ORIENTED_EDGE('',*,*,#16857,.T.);
#24214=ORIENTED_EDGE('',*,*,#16852,.T.);
#24215=ORIENTED_EDGE('',*,*,#16779,.F.);
#24216=ORIENTED_EDGE('',*,*,#16849,.T.);
#24217=ORIENTED_EDGE('',*,*,#16851,.T.);
#24218=ORIENTED_EDGE('',*,*,#16846,.T.);
#24219=ORIENTED_EDGE('',*,*,#16776,.F.);
#24220=ORIENTED_EDGE('',*,*,#16843,.T.);
#24221=ORIENTED_EDGE('',*,*,#16845,.T.);
#24222=ORIENTED_EDGE('',*,*,#16840,.T.);
#24223=ORIENTED_EDGE('',*,*,#16773,.F.);
#24224=ORIENTED_EDGE('',*,*,#16837,.T.);
#24225=ORIENTED_EDGE('',*,*,#16839,.T.);
#24226=ORIENTED_EDGE('',*,*,#16834,.T.);
#24227=ORIENTED_EDGE('',*,*,#16770,.F.);
#24228=ORIENTED_EDGE('',*,*,#16831,.T.);
#24229=ORIENTED_EDGE('',*,*,#16833,.T.);
#24230=ORIENTED_EDGE('',*,*,#16828,.T.);
#24231=ORIENTED_EDGE('',*,*,#16767,.F.);
#24232=ORIENTED_EDGE('',*,*,#16825,.T.);
#24233=ORIENTED_EDGE('',*,*,#16827,.T.);
#24234=ORIENTED_EDGE('',*,*,#16822,.T.);
#24235=ORIENTED_EDGE('',*,*,#16764,.F.);
#24236=ORIENTED_EDGE('',*,*,#16819,.T.);
#24237=ORIENTED_EDGE('',*,*,#16821,.T.);
#24238=ORIENTED_EDGE('',*,*,#16816,.T.);
#24239=ORIENTED_EDGE('',*,*,#16761,.F.);
#24240=ORIENTED_EDGE('',*,*,#16813,.T.);
#24241=ORIENTED_EDGE('',*,*,#16815,.T.);
#24242=ORIENTED_EDGE('',*,*,#16810,.T.);
#24243=ORIENTED_EDGE('',*,*,#16758,.F.);
#24244=ORIENTED_EDGE('',*,*,#16698,.T.);
#24245=ORIENTED_EDGE('',*,*,#16701,.T.);
#24246=ORIENTED_EDGE('',*,*,#16694,.T.);
#24247=ORIENTED_EDGE('',*,*,#16757,.F.);
#24248=ORIENTED_EDGE('',*,*,#17018,.T.);
#24249=ORIENTED_EDGE('',*,*,#17020,.T.);
#24250=ORIENTED_EDGE('',*,*,#17015,.T.);
#24251=ORIENTED_EDGE('',*,*,#16754,.F.);
#24252=ORIENTED_EDGE('',*,*,#17012,.T.);
#24253=ORIENTED_EDGE('',*,*,#17014,.T.);
#24254=ORIENTED_EDGE('',*,*,#17009,.T.);
#24255=ORIENTED_EDGE('',*,*,#16751,.F.);
#24256=ORIENTED_EDGE('',*,*,#17006,.T.);
#24257=ORIENTED_EDGE('',*,*,#17008,.T.);
#24258=ORIENTED_EDGE('',*,*,#17003,.T.);
#24259=ORIENTED_EDGE('',*,*,#16748,.F.);
#24260=ORIENTED_EDGE('',*,*,#17000,.T.);
#24261=ORIENTED_EDGE('',*,*,#17002,.T.);
#24262=ORIENTED_EDGE('',*,*,#16997,.T.);
#24263=ORIENTED_EDGE('',*,*,#16745,.F.);
#24264=ORIENTED_EDGE('',*,*,#16994,.T.);
#24265=ORIENTED_EDGE('',*,*,#16996,.T.);
#24266=ORIENTED_EDGE('',*,*,#16991,.T.);
#24267=ORIENTED_EDGE('',*,*,#16742,.F.);
#24268=ORIENTED_EDGE('',*,*,#16988,.T.);
#24269=ORIENTED_EDGE('',*,*,#16990,.T.);
#24270=ORIENTED_EDGE('',*,*,#16985,.T.);
#24271=ORIENTED_EDGE('',*,*,#16739,.F.);
#24272=ORIENTED_EDGE('',*,*,#16982,.T.);
#24273=ORIENTED_EDGE('',*,*,#16984,.T.);
#24274=ORIENTED_EDGE('',*,*,#16979,.T.);
#24275=ORIENTED_EDGE('',*,*,#16736,.F.);
#24276=ORIENTED_EDGE('',*,*,#16976,.T.);
#24277=ORIENTED_EDGE('',*,*,#16978,.T.);
#24278=ORIENTED_EDGE('',*,*,#16973,.T.);
#24279=ORIENTED_EDGE('',*,*,#16733,.F.);
#24280=ORIENTED_EDGE('',*,*,#16970,.T.);
#24281=ORIENTED_EDGE('',*,*,#16972,.T.);
#24282=ORIENTED_EDGE('',*,*,#16967,.T.);
#24283=ORIENTED_EDGE('',*,*,#16730,.F.);
#24284=ORIENTED_EDGE('',*,*,#16964,.T.);
#24285=ORIENTED_EDGE('',*,*,#16966,.T.);
#24286=ORIENTED_EDGE('',*,*,#16961,.T.);
#24287=ORIENTED_EDGE('',*,*,#16727,.F.);
#24288=ORIENTED_EDGE('',*,*,#16958,.T.);
#24289=ORIENTED_EDGE('',*,*,#16960,.T.);
#24290=ORIENTED_EDGE('',*,*,#16955,.T.);
#24291=ORIENTED_EDGE('',*,*,#16724,.F.);
#24292=ORIENTED_EDGE('',*,*,#16952,.T.);
#24293=ORIENTED_EDGE('',*,*,#16954,.T.);
#24294=ORIENTED_EDGE('',*,*,#16949,.T.);
#24295=ORIENTED_EDGE('',*,*,#16721,.F.);
#24296=ORIENTED_EDGE('',*,*,#16946,.T.);
#24297=ORIENTED_EDGE('',*,*,#16948,.T.);
#24298=ORIENTED_EDGE('',*,*,#16943,.T.);
#24299=ORIENTED_EDGE('',*,*,#16718,.F.);
#24300=ORIENTED_EDGE('',*,*,#16940,.T.);
#24301=ORIENTED_EDGE('',*,*,#16942,.T.);
#24302=ORIENTED_EDGE('',*,*,#16937,.T.);
#24303=ORIENTED_EDGE('',*,*,#16715,.F.);
#24304=ORIENTED_EDGE('',*,*,#16934,.T.);
#24305=ORIENTED_EDGE('',*,*,#16936,.T.);
#24306=ORIENTED_EDGE('',*,*,#16931,.T.);
#24307=ORIENTED_EDGE('',*,*,#16712,.F.);
#24308=ORIENTED_EDGE('',*,*,#16928,.T.);
#24309=ORIENTED_EDGE('',*,*,#16930,.T.);
#24310=ORIENTED_EDGE('',*,*,#16925,.T.);
#24311=ORIENTED_EDGE('',*,*,#16709,.F.);
#24312=ORIENTED_EDGE('',*,*,#16922,.T.);
#24313=ORIENTED_EDGE('',*,*,#16924,.T.);
#24314=ORIENTED_EDGE('',*,*,#16919,.T.);
#24315=ORIENTED_EDGE('',*,*,#16706,.F.);
#24316=ORIENTED_EDGE('',*,*,#16916,.T.);
#24317=ORIENTED_EDGE('',*,*,#16918,.T.);
#24318=ORIENTED_EDGE('',*,*,#16913,.T.);
#24319=ORIENTED_EDGE('',*,*,#16703,.F.);
#24320=ORIENTED_EDGE('',*,*,#16909,.T.);
#24321=ORIENTED_EDGE('',*,*,#16809,.F.);
#24322=ORIENTED_EDGE('',*,*,#17022,.T.);
#24323=ORIENTED_EDGE('',*,*,#17023,.T.);
#24324=ORIENTED_EDGE('',*,*,#17024,.T.);
#24325=ORIENTED_EDGE('',*,*,#17025,.T.);
#24326=ORIENTED_EDGE('',*,*,#17026,.T.);
#24327=ORIENTED_EDGE('',*,*,#17027,.T.);
#24328=ORIENTED_EDGE('',*,*,#17028,.F.);
#24329=ORIENTED_EDGE('',*,*,#17029,.T.);
#24330=ORIENTED_EDGE('',*,*,#17030,.F.);
#24331=ORIENTED_EDGE('',*,*,#17031,.T.);
#24332=ORIENTED_EDGE('',*,*,#17032,.F.);
#24333=ORIENTED_EDGE('',*,*,#17033,.T.);
#24334=ORIENTED_EDGE('',*,*,#17034,.F.);
#24335=ORIENTED_EDGE('',*,*,#17035,.T.);
#24336=ORIENTED_EDGE('',*,*,#17036,.F.);
#24337=ORIENTED_EDGE('',*,*,#17037,.T.);
#24338=ORIENTED_EDGE('',*,*,#17038,.F.);
#24339=ORIENTED_EDGE('',*,*,#17039,.T.);
#24340=ORIENTED_EDGE('',*,*,#17040,.T.);
#24341=ORIENTED_EDGE('',*,*,#17039,.F.);
#24342=ORIENTED_EDGE('',*,*,#17037,.F.);
#24343=ORIENTED_EDGE('',*,*,#17035,.F.);
#24344=ORIENTED_EDGE('',*,*,#17033,.F.);
#24345=ORIENTED_EDGE('',*,*,#17031,.F.);
#24346=ORIENTED_EDGE('',*,*,#17029,.F.);
#24347=ORIENTED_EDGE('',*,*,#17040,.F.);
#24348=ORIENTED_EDGE('',*,*,#17022,.F.);
#24349=ORIENTED_EDGE('',*,*,#17041,.T.);
#24350=ORIENTED_EDGE('',*,*,#17028,.T.);
#24351=ORIENTED_EDGE('',*,*,#17042,.F.);
#24352=ORIENTED_EDGE('',*,*,#17027,.F.);
#24353=ORIENTED_EDGE('',*,*,#17043,.T.);
#24354=ORIENTED_EDGE('',*,*,#17038,.T.);
#24355=ORIENTED_EDGE('',*,*,#17041,.F.);
#24356=ORIENTED_EDGE('',*,*,#17026,.F.);
#24357=ORIENTED_EDGE('',*,*,#17044,.T.);
#24358=ORIENTED_EDGE('',*,*,#17036,.T.);
#24359=ORIENTED_EDGE('',*,*,#17043,.F.);
#24360=ORIENTED_EDGE('',*,*,#17025,.F.);
#24361=ORIENTED_EDGE('',*,*,#17045,.T.);
#24362=ORIENTED_EDGE('',*,*,#17034,.T.);
#24363=ORIENTED_EDGE('',*,*,#17044,.F.);
#24364=ORIENTED_EDGE('',*,*,#17024,.F.);
#24365=ORIENTED_EDGE('',*,*,#17046,.T.);
#24366=ORIENTED_EDGE('',*,*,#17032,.T.);
#24367=ORIENTED_EDGE('',*,*,#17045,.F.);
#24368=ORIENTED_EDGE('',*,*,#17023,.F.);
#24369=ORIENTED_EDGE('',*,*,#17042,.T.);
#24370=ORIENTED_EDGE('',*,*,#17030,.T.);
#24371=ORIENTED_EDGE('',*,*,#17046,.F.);
#25539=CONICAL_SURFACE('',#28720,1.52934,0.785398163397445);
#25540=CONICAL_SURFACE('',#28727,2.7202,0.785398163397445);
#25541=CONICAL_SURFACE('',#28920,1.60395121659243,1.02974425867665);
#26611=ADVANCED_FACE('',(#3418),#2318,.T.);
#26612=ADVANCED_FACE('',(#3419),#2319,.T.);
#26613=ADVANCED_FACE('',(#3420),#2320,.T.);
#26614=ADVANCED_FACE('',(#3421),#2321,.T.);
#26615=ADVANCED_FACE('',(#3422),#2322,.T.);
#26616=ADVANCED_FACE('',(#3423),#2323,.T.);
#26617=ADVANCED_FACE('',(#3424),#2324,.T.);
#26618=ADVANCED_FACE('',(#3425),#2325,.T.);
#26619=ADVANCED_FACE('',(#3426),#2326,.T.);
#26620=ADVANCED_FACE('',(#3427),#2327,.T.);
#26621=ADVANCED_FACE('',(#3428),#2328,.T.);
#26622=ADVANCED_FACE('',(#3429),#1880,.T.);
#26623=ADVANCED_FACE('',(#3430),#901,.F.);
#26624=ADVANCED_FACE('',(#3431),#1881,.F.);
#26625=ADVANCED_FACE('',(#3432),#902,.F.);
#26626=ADVANCED_FACE('',(#3433),#506,.F.);
#26627=ADVANCED_FACE('',(#3434,#1113),#1882,.F.);
#26628=ADVANCED_FACE('',(#3435),#25539,.T.);
#26629=ADVANCED_FACE('',(#3436),#1883,.F.);
#26630=ADVANCED_FACE('',(#3437),#1884,.F.);
#26631=ADVANCED_FACE('',(#3438),#1885,.F.);
#26632=ADVANCED_FACE('',(#3439),#1886,.F.);
#26633=ADVANCED_FACE('',(#3440),#25540,.T.);
#26634=ADVANCED_FACE('',(#3441),#1887,.F.);
#26635=ADVANCED_FACE('',(#3442),#1888,.F.);
#26636=ADVANCED_FACE('',(#3443),#1889,.F.);
#26637=ADVANCED_FACE('',(#3444),#1890,.F.);
#26638=ADVANCED_FACE('',(#3445),#1891,.F.);
#26639=ADVANCED_FACE('',(#3446),#1892,.F.);
#26640=ADVANCED_FACE('',(#3447),#1893,.F.);
#26641=ADVANCED_FACE('',(#3448),#1894,.F.);
#26642=ADVANCED_FACE('',(#3449),#1895,.F.);
#26643=ADVANCED_FACE('',(#3450),#1896,.F.);
#26644=ADVANCED_FACE('',(#3451),#1897,.F.);
#26645=ADVANCED_FACE('',(#3452),#1898,.F.);
#26646=ADVANCED_FACE('',(#3453),#1899,.F.);
#26647=ADVANCED_FACE('',(#3454),#1900,.F.);
#26648=ADVANCED_FACE('',(#3455),#1901,.F.);
#26649=ADVANCED_FACE('',(#3456),#1902,.F.);
#26650=ADVANCED_FACE('',(#3457),#1903,.F.);
#26651=ADVANCED_FACE('',(#3458),#1904,.F.);
#26652=ADVANCED_FACE('',(#3459),#1905,.F.);
#26653=ADVANCED_FACE('',(#3460),#1906,.F.);
#26654=ADVANCED_FACE('',(#3461),#1907,.F.);
#26655=ADVANCED_FACE('',(#3462),#1908,.F.);
#26656=ADVANCED_FACE('',(#3463),#1909,.F.);
#26657=ADVANCED_FACE('',(#3464),#1910,.F.);
#26658=ADVANCED_FACE('',(#3465),#1911,.F.);
#26659=ADVANCED_FACE('',(#3466),#1912,.F.);
#26660=ADVANCED_FACE('',(#3467),#1913,.F.);
#26661=ADVANCED_FACE('',(#3468),#1914,.F.);
#26662=ADVANCED_FACE('',(#3469),#1915,.F.);
#26663=ADVANCED_FACE('',(#3470),#1916,.F.);
#26664=ADVANCED_FACE('',(#3471),#1917,.F.);
#26665=ADVANCED_FACE('',(#3472),#1918,.F.);
#26666=ADVANCED_FACE('',(#3473),#1919,.F.);
#26667=ADVANCED_FACE('',(#3474),#1920,.F.);
#26668=ADVANCED_FACE('',(#3475),#1921,.F.);
#26669=ADVANCED_FACE('',(#3476),#1922,.F.);
#26670=ADVANCED_FACE('',(#3477),#1923,.F.);
#26671=ADVANCED_FACE('',(#3478),#1924,.F.);
#26672=ADVANCED_FACE('',(#3479),#1925,.F.);
#26673=ADVANCED_FACE('',(#3480),#1926,.F.);
#26674=ADVANCED_FACE('',(#3481),#1927,.F.);
#26675=ADVANCED_FACE('',(#3482),#1928,.F.);
#26676=ADVANCED_FACE('',(#3483),#1929,.F.);
#26677=ADVANCED_FACE('',(#3484),#1930,.F.);
#26678=ADVANCED_FACE('',(#3485),#1931,.F.);
#26679=ADVANCED_FACE('',(#3486),#1932,.F.);
#26680=ADVANCED_FACE('',(#3487),#1933,.F.);
#26681=ADVANCED_FACE('',(#3488),#1934,.F.);
#26682=ADVANCED_FACE('',(#3489),#1935,.F.);
#26683=ADVANCED_FACE('',(#3490),#1936,.F.);
#26684=ADVANCED_FACE('',(#3491),#1937,.F.);
#26685=ADVANCED_FACE('',(#3492),#1938,.F.);
#26686=ADVANCED_FACE('',(#3493),#1939,.F.);
#26687=ADVANCED_FACE('',(#3494),#1940,.F.);
#26688=ADVANCED_FACE('',(#3495),#1941,.F.);
#26689=ADVANCED_FACE('',(#3496),#1942,.F.);
#26690=ADVANCED_FACE('',(#3497),#1943,.F.);
#26691=ADVANCED_FACE('',(#3498),#1944,.F.);
#26692=ADVANCED_FACE('',(#3499),#1945,.F.);
#26693=ADVANCED_FACE('',(#3500),#1946,.F.);
#26694=ADVANCED_FACE('',(#3501),#1947,.F.);
#26695=ADVANCED_FACE('',(#3502),#1948,.F.);
#26696=ADVANCED_FACE('',(#3503),#1949,.F.);
#26697=ADVANCED_FACE('',(#3504),#1950,.F.);
#26698=ADVANCED_FACE('',(#3505),#1951,.F.);
#26699=ADVANCED_FACE('',(#3506),#1952,.F.);
#26700=ADVANCED_FACE('',(#3507),#1953,.F.);
#26701=ADVANCED_FACE('',(#3508),#1954,.F.);
#26702=ADVANCED_FACE('',(#3509),#1955,.F.);
#26703=ADVANCED_FACE('',(#3510),#1956,.F.);
#26704=ADVANCED_FACE('',(#3511),#1957,.F.);
#26705=ADVANCED_FACE('',(#3512),#1958,.F.);
#26706=ADVANCED_FACE('',(#3513),#1959,.F.);
#26707=ADVANCED_FACE('',(#3514),#1960,.F.);
#26708=ADVANCED_FACE('',(#3515),#1961,.F.);
#26709=ADVANCED_FACE('',(#3516),#1962,.F.);
#26710=ADVANCED_FACE('',(#3517),#1963,.F.);
#26711=ADVANCED_FACE('',(#3518),#1964,.F.);
#26712=ADVANCED_FACE('',(#3519),#1965,.F.);
#26713=ADVANCED_FACE('',(#3520),#1966,.F.);
#26714=ADVANCED_FACE('',(#3521),#1967,.F.);
#26715=ADVANCED_FACE('',(#3522),#1968,.F.);
#26716=ADVANCED_FACE('',(#3523),#1969,.F.);
#26717=ADVANCED_FACE('',(#3524),#1970,.F.);
#26718=ADVANCED_FACE('',(#3525),#1971,.F.);
#26719=ADVANCED_FACE('',(#3526),#1972,.F.);
#26720=ADVANCED_FACE('',(#3527),#1973,.F.);
#26721=ADVANCED_FACE('',(#3528),#1974,.F.);
#26722=ADVANCED_FACE('',(#3529),#1975,.F.);
#26723=ADVANCED_FACE('',(#3530),#1976,.F.);
#26724=ADVANCED_FACE('',(#3531),#1977,.F.);
#26725=ADVANCED_FACE('',(#3532),#1978,.F.);
#26726=ADVANCED_FACE('',(#3533),#1979,.F.);
#26727=ADVANCED_FACE('',(#3534),#1980,.F.);
#26728=ADVANCED_FACE('',(#3535),#1981,.F.);
#26729=ADVANCED_FACE('',(#3536),#1982,.F.);
#26730=ADVANCED_FACE('',(#3537),#1983,.F.);
#26731=ADVANCED_FACE('',(#3538),#1984,.F.);
#26732=ADVANCED_FACE('',(#3539),#1985,.F.);
#26733=ADVANCED_FACE('',(#3540),#1986,.F.);
#26734=ADVANCED_FACE('',(#3541),#1987,.F.);
#26735=ADVANCED_FACE('',(#3542),#1988,.F.);
#26736=ADVANCED_FACE('',(#3543),#1989,.F.);
#26737=ADVANCED_FACE('',(#3544),#1990,.F.);
#26738=ADVANCED_FACE('',(#3545),#1991,.F.);
#26739=ADVANCED_FACE('',(#3546),#2329,.T.);
#26740=ADVANCED_FACE('',(#3547,#1114),#1992,.T.);
#26741=ADVANCED_FACE('',(#3548),#1993,.F.);
#26742=ADVANCED_FACE('',(#3549),#1994,.F.);
#26743=ADVANCED_FACE('',(#3550),#1995,.F.);
#26744=ADVANCED_FACE('',(#3551),#1996,.F.);
#26745=ADVANCED_FACE('',(#3552),#1997,.F.);
#26746=ADVANCED_FACE('',(#3553),#1998,.F.);
#26747=ADVANCED_FACE('',(#3554),#25541,.F.);
#26748=ADVANCED_FACE('',(#3555),#1999,.F.);
#26749=ADVANCED_FACE('',(#3556),#2000,.F.);
#26750=ADVANCED_FACE('',(#3557),#2001,.F.);
#26751=ADVANCED_FACE('',(#3558),#2002,.F.);
#26752=ADVANCED_FACE('',(#3559),#2003,.F.);
#26753=ADVANCED_FACE('',(#3560),#2004,.F.);
#26939=CLOSED_SHELL('',(#26611,#26612,#26613,#26614,#26615,#26616,#26617,
#26618,#26619,#26620,#26621,#26622,#26623,#26624,#26625,#26626,#26627,#26628,
#26629,#26630,#26631,#26632,#26633,#26634,#26635,#26636,#26637,#26638,#26639,
#26640,#26641,#26642,#26643,#26644,#26645,#26646,#26647,#26648,#26649,#26650,
#26651,#26652,#26653,#26654,#26655,#26656,#26657,#26658,#26659,#26660,#26661,
#26662,#26663,#26664,#26665,#26666,#26667,#26668,#26669,#26670,#26671,#26672,
#26673,#26674,#26675,#26676,#26677,#26678,#26679,#26680,#26681,#26682,#26683,
#26684,#26685,#26686,#26687,#26688,#26689,#26690,#26691,#26692,#26693,#26694,
#26695,#26696,#26697,#26698,#26699,#26700,#26701,#26702,#26703,#26704,#26705,
#26706,#26707,#26708,#26709,#26710,#26711,#26712,#26713,#26714,#26715,#26716,
#26717,#26718,#26719,#26720,#26721,#26722,#26723,#26724,#26725,#26726,#26727,
#26728,#26729,#26730,#26731,#26732,#26733,#26734,#26735,#26736,#26737,#26738,
#26739,#26740,#26741,#26742,#26743,#26744,#26745,#26746,#26747,#26748,#26749,
#26750,#26751,#26752,#26753));
#28693=AXIS2_PLACEMENT_3D('',#59383,#34502,#34503);
#28694=AXIS2_PLACEMENT_3D('',#59384,#34504,#34505);
#28695=AXIS2_PLACEMENT_3D('',#59517,#34507,#34508);
#28696=AXIS2_PLACEMENT_3D('',#59606,#34509,#34510);
#28697=AXIS2_PLACEMENT_3D('',#59939,#34512,#34513);
#28698=AXIS2_PLACEMENT_3D('',#60135,#34515,#34516);
#28699=AXIS2_PLACEMENT_3D('',#60332,#34518,#34519);
#28700=AXIS2_PLACEMENT_3D('',#60511,#34521,#34522);
#28701=AXIS2_PLACEMENT_3D('',#60811,#34524,#34525);
#28702=AXIS2_PLACEMENT_3D('',#61130,#34527,#34528);
#28703=AXIS2_PLACEMENT_3D('',#61451,#34530,#34531);
#28704=AXIS2_PLACEMENT_3D('',#61780,#34533,#34534);
#28705=AXIS2_PLACEMENT_3D('',#61845,#34535,#34536);
#28706=AXIS2_PLACEMENT_3D('',#63460,#34537,#34538);
#28707=AXIS2_PLACEMENT_3D('',#64860,#34539,#34540);
#28708=AXIS2_PLACEMENT_3D('',#65016,#34541,#34542);
#28709=AXIS2_PLACEMENT_3D('',#65132,#34543,#34544);
#28710=AXIS2_PLACEMENT_3D('',#65135,#34545,#34546);
#28711=AXIS2_PLACEMENT_3D('',#65291,#34547,#34548);
#28712=AXIS2_PLACEMENT_3D('',#65631,#34549,#34550);
#28713=AXIS2_PLACEMENT_3D('',#65634,#34551,#34552);
#28714=AXIS2_PLACEMENT_3D('',#65711,#34553,#34554);
#28715=AXIS2_PLACEMENT_3D('',#65972,#34555,#34556);
#28716=AXIS2_PLACEMENT_3D('',#65974,#34557,#34558);
#28717=AXIS2_PLACEMENT_3D('',#65975,#34559,#34560);
#28718=AXIS2_PLACEMENT_3D('',#65976,#34561,#34562);
#28719=AXIS2_PLACEMENT_3D('',#65978,#34563,#34564);
#28720=AXIS2_PLACEMENT_3D('',#65979,#34565,#34566);
#28721=AXIS2_PLACEMENT_3D('',#65982,#34568,#34569);
#28722=AXIS2_PLACEMENT_3D('',#65983,#34570,#34571);
#28723=AXIS2_PLACEMENT_3D('',#65984,#34572,#34573);
#28724=AXIS2_PLACEMENT_3D('',#65995,#34577,#34578);
#28725=AXIS2_PLACEMENT_3D('',#66003,#34581,#34582);
#28726=AXIS2_PLACEMENT_3D('',#66004,#34583,#34584);
#28727=AXIS2_PLACEMENT_3D('',#66005,#34585,#34586);
#28728=AXIS2_PLACEMENT_3D('',#66012,#34587,#34588);
#28729=AXIS2_PLACEMENT_3D('',#66022,#34589,#34590);
#28730=AXIS2_PLACEMENT_3D('',#66032,#34591,#34592);
#28731=AXIS2_PLACEMENT_3D('',#66042,#34593,#34594);
#28732=AXIS2_PLACEMENT_3D('',#66052,#34595,#34596);
#28733=AXIS2_PLACEMENT_3D('',#66062,#34597,#34598);
#28734=AXIS2_PLACEMENT_3D('',#66072,#34599,#34600);
#28735=AXIS2_PLACEMENT_3D('',#66082,#34601,#34602);
#28736=AXIS2_PLACEMENT_3D('',#66092,#34603,#34604);
#28737=AXIS2_PLACEMENT_3D('',#66102,#34605,#34606);
#28738=AXIS2_PLACEMENT_3D('',#66112,#34607,#34608);
#28739=AXIS2_PLACEMENT_3D('',#66122,#34609,#34610);
#28740=AXIS2_PLACEMENT_3D('',#66132,#34611,#34612);
#28741=AXIS2_PLACEMENT_3D('',#66142,#34613,#34614);
#28742=AXIS2_PLACEMENT_3D('',#66152,#34615,#34616);
#28743=AXIS2_PLACEMENT_3D('',#66162,#34617,#34618);
#28744=AXIS2_PLACEMENT_3D('',#66172,#34619,#34620);
#28745=AXIS2_PLACEMENT_3D('',#66182,#34621,#34622);
#28746=AXIS2_PLACEMENT_3D('',#66191,#34623,#34624);
#28747=AXIS2_PLACEMENT_3D('',#66193,#34625,#34626);
#28748=AXIS2_PLACEMENT_3D('',#66203,#34627,#34628);
#28749=AXIS2_PLACEMENT_3D('',#66213,#34629,#34630);
#28750=AXIS2_PLACEMENT_3D('',#66223,#34631,#34632);
#28751=AXIS2_PLACEMENT_3D('',#66233,#34633,#34634);
#28752=AXIS2_PLACEMENT_3D('',#66243,#34635,#34636);
#28753=AXIS2_PLACEMENT_3D('',#66253,#34637,#34638);
#28754=AXIS2_PLACEMENT_3D('',#66263,#34639,#34640);
#28755=AXIS2_PLACEMENT_3D('',#66273,#34641,#34642);
#28756=AXIS2_PLACEMENT_3D('',#66283,#34643,#34644);
#28757=AXIS2_PLACEMENT_3D('',#66293,#34645,#34646);
#28758=AXIS2_PLACEMENT_3D('',#66303,#34647,#34648);
#28759=AXIS2_PLACEMENT_3D('',#66313,#34649,#34650);
#28760=AXIS2_PLACEMENT_3D('',#66323,#34651,#34652);
#28761=AXIS2_PLACEMENT_3D('',#66333,#34653,#34654);
#28762=AXIS2_PLACEMENT_3D('',#66343,#34655,#34656);
#28763=AXIS2_PLACEMENT_3D('',#66353,#34657,#34658);
#28764=AXIS2_PLACEMENT_3D('',#66359,#34660,#34661);
#28765=AXIS2_PLACEMENT_3D('',#66360,#34662,#34663);
#28766=AXIS2_PLACEMENT_3D('',#66366,#34667,#34668);
#28767=AXIS2_PLACEMENT_3D('',#66370,#34671,#34672);
#28768=AXIS2_PLACEMENT_3D('',#66371,#34673,#34674);
#28769=AXIS2_PLACEMENT_3D('',#66372,#34675,#34676);
#28770=AXIS2_PLACEMENT_3D('',#66378,#34680,#34681);
#28771=AXIS2_PLACEMENT_3D('',#66382,#34684,#34685);
#28772=AXIS2_PLACEMENT_3D('',#66383,#34686,#34687);
#28773=AXIS2_PLACEMENT_3D('',#66384,#34688,#34689);
#28774=AXIS2_PLACEMENT_3D('',#66390,#34693,#34694);
#28775=AXIS2_PLACEMENT_3D('',#66394,#34697,#34698);
#28776=AXIS2_PLACEMENT_3D('',#66395,#34699,#34700);
#28777=AXIS2_PLACEMENT_3D('',#66396,#34701,#34702);
#28778=AXIS2_PLACEMENT_3D('',#66402,#34706,#34707);
#28779=AXIS2_PLACEMENT_3D('',#66406,#34710,#34711);
#28780=AXIS2_PLACEMENT_3D('',#66407,#34712,#34713);
#28781=AXIS2_PLACEMENT_3D('',#66408,#34714,#34715);
#28782=AXIS2_PLACEMENT_3D('',#66414,#34719,#34720);
#28783=AXIS2_PLACEMENT_3D('',#66418,#34723,#34724);
#28784=AXIS2_PLACEMENT_3D('',#66419,#34725,#34726);
#28785=AXIS2_PLACEMENT_3D('',#66420,#34727,#34728);
#28786=AXIS2_PLACEMENT_3D('',#66426,#34732,#34733);
#28787=AXIS2_PLACEMENT_3D('',#66430,#34736,#34737);
#28788=AXIS2_PLACEMENT_3D('',#66431,#34738,#34739);
#28789=AXIS2_PLACEMENT_3D('',#66432,#34740,#34741);
#28790=AXIS2_PLACEMENT_3D('',#66438,#34745,#34746);
#28791=AXIS2_PLACEMENT_3D('',#66442,#34749,#34750);
#28792=AXIS2_PLACEMENT_3D('',#66443,#34751,#34752);
#28793=AXIS2_PLACEMENT_3D('',#66444,#34753,#34754);
#28794=AXIS2_PLACEMENT_3D('',#66450,#34758,#34759);
#28795=AXIS2_PLACEMENT_3D('',#66454,#34762,#34763);
#28796=AXIS2_PLACEMENT_3D('',#66455,#34764,#34765);
#28797=AXIS2_PLACEMENT_3D('',#66456,#34766,#34767);
#28798=AXIS2_PLACEMENT_3D('',#66462,#34771,#34772);
#28799=AXIS2_PLACEMENT_3D('',#66466,#34775,#34776);
#28800=AXIS2_PLACEMENT_3D('',#66467,#34777,#34778);
#28801=AXIS2_PLACEMENT_3D('',#66468,#34779,#34780);
#28802=AXIS2_PLACEMENT_3D('',#66474,#34784,#34785);
#28803=AXIS2_PLACEMENT_3D('',#66478,#34788,#34789);
#28804=AXIS2_PLACEMENT_3D('',#66479,#34790,#34791);
#28805=AXIS2_PLACEMENT_3D('',#66480,#34792,#34793);
#28806=AXIS2_PLACEMENT_3D('',#66486,#34797,#34798);
#28807=AXIS2_PLACEMENT_3D('',#66490,#34801,#34802);
#28808=AXIS2_PLACEMENT_3D('',#66491,#34803,#34804);
#28809=AXIS2_PLACEMENT_3D('',#66492,#34805,#34806);
#28810=AXIS2_PLACEMENT_3D('',#66498,#34810,#34811);
#28811=AXIS2_PLACEMENT_3D('',#66502,#34814,#34815);
#28812=AXIS2_PLACEMENT_3D('',#66503,#34816,#34817);
#28813=AXIS2_PLACEMENT_3D('',#66504,#34818,#34819);
#28814=AXIS2_PLACEMENT_3D('',#66510,#34823,#34824);
#28815=AXIS2_PLACEMENT_3D('',#66514,#34827,#34828);
#28816=AXIS2_PLACEMENT_3D('',#66515,#34829,#34830);
#28817=AXIS2_PLACEMENT_3D('',#66516,#34831,#34832);
#28818=AXIS2_PLACEMENT_3D('',#66522,#34836,#34837);
#28819=AXIS2_PLACEMENT_3D('',#66526,#34840,#34841);
#28820=AXIS2_PLACEMENT_3D('',#66527,#34842,#34843);
#28821=AXIS2_PLACEMENT_3D('',#66528,#34844,#34845);
#28822=AXIS2_PLACEMENT_3D('',#66534,#34849,#34850);
#28823=AXIS2_PLACEMENT_3D('',#66538,#34853,#34854);
#28824=AXIS2_PLACEMENT_3D('',#66539,#34855,#34856);
#28825=AXIS2_PLACEMENT_3D('',#66540,#34857,#34858);
#28826=AXIS2_PLACEMENT_3D('',#66546,#34862,#34863);
#28827=AXIS2_PLACEMENT_3D('',#66550,#34866,#34867);
#28828=AXIS2_PLACEMENT_3D('',#66551,#34868,#34869);
#28829=AXIS2_PLACEMENT_3D('',#66552,#34870,#34871);
#28830=AXIS2_PLACEMENT_3D('',#66558,#34875,#34876);
#28831=AXIS2_PLACEMENT_3D('',#66562,#34879,#34880);
#28832=AXIS2_PLACEMENT_3D('',#66564,#34881,#34882);
#28833=AXIS2_PLACEMENT_3D('',#66565,#34883,#34884);
#28834=AXIS2_PLACEMENT_3D('',#66566,#34885,#34886);
#28835=AXIS2_PLACEMENT_3D('',#66572,#34890,#34891);
#28836=AXIS2_PLACEMENT_3D('',#66576,#34894,#34895);
#28837=AXIS2_PLACEMENT_3D('',#66577,#34896,#34897);
#28838=AXIS2_PLACEMENT_3D('',#66578,#34898,#34899);
#28839=AXIS2_PLACEMENT_3D('',#66584,#34903,#34904);
#28840=AXIS2_PLACEMENT_3D('',#66588,#34907,#34908);
#28841=AXIS2_PLACEMENT_3D('',#66589,#34909,#34910);
#28842=AXIS2_PLACEMENT_3D('',#66590,#34911,#34912);
#28843=AXIS2_PLACEMENT_3D('',#66596,#34916,#34917);
#28844=AXIS2_PLACEMENT_3D('',#66600,#34920,#34921);
#28845=AXIS2_PLACEMENT_3D('',#66601,#34922,#34923);
#28846=AXIS2_PLACEMENT_3D('',#66602,#34924,#34925);
#28847=AXIS2_PLACEMENT_3D('',#66608,#34929,#34930);
#28848=AXIS2_PLACEMENT_3D('',#66612,#34933,#34934);
#28849=AXIS2_PLACEMENT_3D('',#66613,#34935,#34936);
#28850=AXIS2_PLACEMENT_3D('',#66614,#34937,#34938);
#28851=AXIS2_PLACEMENT_3D('',#66620,#34942,#34943);
#28852=AXIS2_PLACEMENT_3D('',#66624,#34946,#34947);
#28853=AXIS2_PLACEMENT_3D('',#66625,#34948,#34949);
#28854=AXIS2_PLACEMENT_3D('',#66626,#34950,#34951);
#28855=AXIS2_PLACEMENT_3D('',#66632,#34955,#34956);
#28856=AXIS2_PLACEMENT_3D('',#66636,#34959,#34960);
#28857=AXIS2_PLACEMENT_3D('',#66637,#34961,#34962);
#28858=AXIS2_PLACEMENT_3D('',#66638,#34963,#34964);
#28859=AXIS2_PLACEMENT_3D('',#66644,#34968,#34969);
#28860=AXIS2_PLACEMENT_3D('',#66648,#34972,#34973);
#28861=AXIS2_PLACEMENT_3D('',#66649,#34974,#34975);
#28862=AXIS2_PLACEMENT_3D('',#66650,#34976,#34977);
#28863=AXIS2_PLACEMENT_3D('',#66656,#34981,#34982);
#28864=AXIS2_PLACEMENT_3D('',#66660,#34985,#34986);
#28865=AXIS2_PLACEMENT_3D('',#66661,#34987,#34988);
#28866=AXIS2_PLACEMENT_3D('',#66662,#34989,#34990);
#28867=AXIS2_PLACEMENT_3D('',#66668,#34994,#34995);
#28868=AXIS2_PLACEMENT_3D('',#66672,#34998,#34999);
#28869=AXIS2_PLACEMENT_3D('',#66673,#35000,#35001);
#28870=AXIS2_PLACEMENT_3D('',#66674,#35002,#35003);
#28871=AXIS2_PLACEMENT_3D('',#66680,#35007,#35008);
#28872=AXIS2_PLACEMENT_3D('',#66684,#35011,#35012);
#28873=AXIS2_PLACEMENT_3D('',#66685,#35013,#35014);
#28874=AXIS2_PLACEMENT_3D('',#66686,#35015,#35016);
#28875=AXIS2_PLACEMENT_3D('',#66692,#35020,#35021);
#28876=AXIS2_PLACEMENT_3D('',#66696,#35024,#35025);
#28877=AXIS2_PLACEMENT_3D('',#66697,#35026,#35027);
#28878=AXIS2_PLACEMENT_3D('',#66698,#35028,#35029);
#28879=AXIS2_PLACEMENT_3D('',#66704,#35033,#35034);
#28880=AXIS2_PLACEMENT_3D('',#66708,#35037,#35038);
#28881=AXIS2_PLACEMENT_3D('',#66709,#35039,#35040);
#28882=AXIS2_PLACEMENT_3D('',#66710,#35041,#35042);
#28883=AXIS2_PLACEMENT_3D('',#66716,#35046,#35047);
#28884=AXIS2_PLACEMENT_3D('',#66720,#35050,#35051);
#28885=AXIS2_PLACEMENT_3D('',#66721,#35052,#35053);
#28886=AXIS2_PLACEMENT_3D('',#66722,#35054,#35055);
#28887=AXIS2_PLACEMENT_3D('',#66728,#35059,#35060);
#28888=AXIS2_PLACEMENT_3D('',#66732,#35063,#35064);
#28889=AXIS2_PLACEMENT_3D('',#66733,#35065,#35066);
#28890=AXIS2_PLACEMENT_3D('',#66734,#35067,#35068);
#28891=AXIS2_PLACEMENT_3D('',#66740,#35072,#35073);
#28892=AXIS2_PLACEMENT_3D('',#66744,#35076,#35077);
#28893=AXIS2_PLACEMENT_3D('',#66745,#35078,#35079);
#28894=AXIS2_PLACEMENT_3D('',#66746,#35080,#35081);
#28895=AXIS2_PLACEMENT_3D('',#66752,#35085,#35086);
#28896=AXIS2_PLACEMENT_3D('',#66756,#35089,#35090);
#28897=AXIS2_PLACEMENT_3D('',#66757,#35091,#35092);
#28898=AXIS2_PLACEMENT_3D('',#66758,#35093,#35094);
#28899=AXIS2_PLACEMENT_3D('',#66764,#35098,#35099);
#28900=AXIS2_PLACEMENT_3D('',#66768,#35102,#35103);
#28901=AXIS2_PLACEMENT_3D('',#66769,#35104,#35105);
#28902=AXIS2_PLACEMENT_3D('',#66770,#35106,#35107);
#28903=AXIS2_PLACEMENT_3D('',#66776,#35111,#35112);
#28904=AXIS2_PLACEMENT_3D('',#66780,#35115,#35116);
#28905=AXIS2_PLACEMENT_3D('',#66781,#35117,#35118);
#28906=AXIS2_PLACEMENT_3D('',#66782,#35119,#35120);
#28907=AXIS2_PLACEMENT_3D('',#66784,#35122,#35123);
#28908=AXIS2_PLACEMENT_3D('',#66797,#35130,#35131);
#28909=AXIS2_PLACEMENT_3D('',#66801,#35133,#35134);
#28910=AXIS2_PLACEMENT_3D('',#66802,#35135,#35136);
#28911=AXIS2_PLACEMENT_3D('',#66805,#35138,#35139);
#28912=AXIS2_PLACEMENT_3D('',#66806,#35140,#35141);
#28913=AXIS2_PLACEMENT_3D('',#66809,#35143,#35144);
#28914=AXIS2_PLACEMENT_3D('',#66810,#35145,#35146);
#28915=AXIS2_PLACEMENT_3D('',#66813,#35148,#35149);
#28916=AXIS2_PLACEMENT_3D('',#66814,#35150,#35151);
#28917=AXIS2_PLACEMENT_3D('',#66817,#35153,#35154);
#28918=AXIS2_PLACEMENT_3D('',#66818,#35155,#35156);
#28919=AXIS2_PLACEMENT_3D('',#66820,#35158,#35159);
#28920=AXIS2_PLACEMENT_3D('',#66821,#35160,#35161);
#28921=AXIS2_PLACEMENT_3D('',#66824,#35163,#35164);
#28922=AXIS2_PLACEMENT_3D('',#66827,#35167,#35168);
#28923=AXIS2_PLACEMENT_3D('',#66829,#35170,#35171);
#28924=AXIS2_PLACEMENT_3D('',#66831,#35173,#35174);
#28925=AXIS2_PLACEMENT_3D('',#66833,#35176,#35177);
#28926=AXIS2_PLACEMENT_3D('',#66835,#35179,#35180);
#34502=DIRECTION('axis',(0.,0.,1.));
#34503=DIRECTION('refdir',(1.,0.,0.));
#34504=DIRECTION('center_axis',(0.,-1.,0.));
#34505=DIRECTION('ref_axis',(0.653826602794498,0.,-0.756644416802375));
#34506=DIRECTION('',(0.,1.,0.));
#34507=DIRECTION('center_axis',(0.,1.,0.));
#34508=DIRECTION('ref_axis',(1.,0.,6.03192037001069E-14));
#34509=DIRECTION('center_axis',(0.,-1.,0.));
#34510=DIRECTION('ref_axis',(0.653826602794498,0.,-0.756644416802375));
#34511=DIRECTION('',(0.,1.,0.));
#34512=DIRECTION('center_axis',(0.,-1.,0.));
#34513=DIRECTION('ref_axis',(0.653826602794498,0.,-0.756644416802375));
#34514=DIRECTION('',(0.,1.,0.));
#34515=DIRECTION('center_axis',(0.,-1.,0.));
#34516=DIRECTION('ref_axis',(0.653826602794498,0.,-0.756644416802375));
#34517=DIRECTION('',(0.,1.,0.));
#34518=DIRECTION('center_axis',(0.,-1.,0.));
#34519=DIRECTION('ref_axis',(0.653826602794498,0.,-0.756644416802375));
#34520=DIRECTION('',(0.,1.,0.));
#34521=DIRECTION('center_axis',(0.,-1.,0.));
#34522=DIRECTION('ref_axis',(0.653826602794498,0.,-0.756644416802375));
#34523=DIRECTION('',(0.,1.,0.));
#34524=DIRECTION('center_axis',(0.,-1.,0.));
#34525=DIRECTION('ref_axis',(0.653826602794498,0.,-0.756644416802375));
#34526=DIRECTION('',(0.,1.,0.));
#34527=DIRECTION('center_axis',(0.,-1.,0.));
#34528=DIRECTION('ref_axis',(0.653826602794498,0.,-0.756644416802375));
#34529=DIRECTION('',(0.,1.,0.));
#34530=DIRECTION('center_axis',(0.,-1.,0.));
#34531=DIRECTION('ref_axis',(0.653826602794498,0.,-0.756644416802375));
#34532=DIRECTION('',(0.,1.,0.));
#34533=DIRECTION('center_axis',(0.,-1.,0.));
#34534=DIRECTION('ref_axis',(1.,0.,0.));
#34535=DIRECTION('center_axis',(0.,1.,0.));
#34536=DIRECTION('ref_axis',(1.,0.,0.));
#34537=DIRECTION('center_axis',(0.,-1.,0.));
#34538=DIRECTION('ref_axis',(1.,0.,0.));
#34539=DIRECTION('center_axis',(0.,-1.,0.));
#34540=DIRECTION('ref_axis',(0.279895837868924,0.,-0.960030374490127));
#34541=DIRECTION('center_axis',(0.,-1.,0.));
#34542=DIRECTION('ref_axis',(1.,0.,6.03192037001069E-14));
#34543=DIRECTION('center_axis',(0.,1.,0.));
#34544=DIRECTION('ref_axis',(0.,0.,1.));
#34545=DIRECTION('center_axis',(0.,-1.,0.));
#34546=DIRECTION('ref_axis',(1.,0.,0.));
#34547=DIRECTION('center_axis',(0.,-1.,0.));
#34548=DIRECTION('ref_axis',(1.,0.,0.));
#34549=DIRECTION('center_axis',(0.,1.,0.));
#34550=DIRECTION('ref_axis',(0.,0.,1.));
#34551=DIRECTION('center_axis',(0.,1.,0.));
#34552=DIRECTION('ref_axis',(1.,0.,0.));
#34553=DIRECTION('center_axis',(0.,1.,0.));
#34554=DIRECTION('ref_axis',(1.,0.,0.));
#34555=DIRECTION('center_axis',(0.,1.,0.));
#34556=DIRECTION('ref_axis',(0.,0.,1.));
#34557=DIRECTION('center_axis',(0.,-1.,0.));
#34558=DIRECTION('ref_axis',(1.,0.,0.));
#34559=DIRECTION('center_axis',(1.,0.,0.));
#34560=DIRECTION('ref_axis',(0.,0.,-1.));
#34561=DIRECTION('center_axis',(0.,1.,0.));
#34562=DIRECTION('ref_axis',(1.,0.,0.));
#34563=DIRECTION('center_axis',(0.,1.,0.));
#34564=DIRECTION('ref_axis',(1.,0.,0.));
#34565=DIRECTION('center_axis',(0.,1.,0.));
#34566=DIRECTION('ref_axis',(1.,0.,0.));
#34567=DIRECTION('',(0.707106781186545,-0.70710678118655,-8.6595605623549E-17));
#34568=DIRECTION('center_axis',(0.,1.,0.));
#34569=DIRECTION('ref_axis',(1.,0.,0.));
#34570=DIRECTION('center_axis',(0.,1.,0.));
#34571=DIRECTION('ref_axis',(1.,0.,0.));
#34572=DIRECTION('center_axis',(-0.188314866426195,0.,0.982108706347156));
#34573=DIRECTION('ref_axis',(-0.982108706347156,0.,-0.188314866426195));
#34574=DIRECTION('',(0.,1.,0.));
#34575=DIRECTION('',(-0.982108706347156,0.,-0.188314866426195));
#34576=DIRECTION('',(0.,-1.,0.));
#34577=DIRECTION('center_axis',(-0.512859050871223,0.,-0.858472826558574));
#34578=DIRECTION('ref_axis',(0.858472826558574,0.,-0.512859050871223));
#34579=DIRECTION('',(0.,-1.,0.));
#34580=DIRECTION('',(0.858472826558574,0.,-0.512859050871223));
#34581=DIRECTION('center_axis',(0.,-1.,0.));
#34582=DIRECTION('ref_axis',(-0.17364817766693,0.,-0.984807753012208));
#34583=DIRECTION('center_axis',(0.,-1.,0.));
#34584=DIRECTION('ref_axis',(1.,0.,0.));
#34585=DIRECTION('center_axis',(0.,-1.,0.));
#34586=DIRECTION('ref_axis',(1.,0.,0.));
#34587=DIRECTION('center_axis',(0.,1.,0.));
#34588=DIRECTION('ref_axis',(1.,0.,0.));
#34589=DIRECTION('center_axis',(0.,1.,0.));
#34590=DIRECTION('ref_axis',(1.,0.,0.));
#34591=DIRECTION('center_axis',(0.,1.,0.));
#34592=DIRECTION('ref_axis',(1.,0.,0.));
#34593=DIRECTION('center_axis',(0.,1.,0.));
#34594=DIRECTION('ref_axis',(1.,0.,0.));
#34595=DIRECTION('center_axis',(0.,1.,0.));
#34596=DIRECTION('ref_axis',(1.,0.,0.));
#34597=DIRECTION('center_axis',(0.,1.,0.));
#34598=DIRECTION('ref_axis',(1.,0.,0.));
#34599=DIRECTION('center_axis',(0.,1.,0.));
#34600=DIRECTION('ref_axis',(1.,0.,0.));
#34601=DIRECTION('center_axis',(0.,1.,0.));
#34602=DIRECTION('ref_axis',(1.,0.,0.));
#34603=DIRECTION('center_axis',(0.,1.,0.));
#34604=DIRECTION('ref_axis',(1.,0.,0.));
#34605=DIRECTION('center_axis',(0.,1.,0.));
#34606=DIRECTION('ref_axis',(1.,0.,0.));
#34607=DIRECTION('center_axis',(0.,1.,0.));
#34608=DIRECTION('ref_axis',(1.,0.,0.));
#34609=DIRECTION('center_axis',(0.,1.,0.));
#34610=DIRECTION('ref_axis',(1.,0.,0.));
#34611=DIRECTION('center_axis',(0.,1.,0.));
#34612=DIRECTION('ref_axis',(1.,0.,0.));
#34613=DIRECTION('center_axis',(0.,1.,0.));
#34614=DIRECTION('ref_axis',(1.,0.,0.));
#34615=DIRECTION('center_axis',(0.,1.,0.));
#34616=DIRECTION('ref_axis',(1.,0.,0.));
#34617=DIRECTION('center_axis',(0.,1.,0.));
#34618=DIRECTION('ref_axis',(1.,0.,0.));
#34619=DIRECTION('center_axis',(0.,1.,0.));
#34620=DIRECTION('ref_axis',(1.,0.,0.));
#34621=DIRECTION('center_axis',(0.,1.,0.));
#34622=DIRECTION('ref_axis',(1.,0.,0.));
#34623=DIRECTION('center_axis',(0.,1.,0.));
#34624=DIRECTION('ref_axis',(1.,0.,0.));
#34625=DIRECTION('center_axis',(0.,1.,0.));
#34626=DIRECTION('ref_axis',(1.,0.,0.));
#34627=DIRECTION('center_axis',(0.,1.,0.));
#34628=DIRECTION('ref_axis',(1.,0.,0.));
#34629=DIRECTION('center_axis',(0.,1.,0.));
#34630=DIRECTION('ref_axis',(1.,0.,0.));
#34631=DIRECTION('center_axis',(0.,1.,0.));
#34632=DIRECTION('ref_axis',(1.,0.,0.));
#34633=DIRECTION('center_axis',(0.,1.,0.));
#34634=DIRECTION('ref_axis',(1.,0.,0.));
#34635=DIRECTION('center_axis',(0.,1.,0.));
#34636=DIRECTION('ref_axis',(1.,0.,0.));
#34637=DIRECTION('center_axis',(0.,1.,0.));
#34638=DIRECTION('ref_axis',(1.,0.,0.));
#34639=DIRECTION('center_axis',(0.,1.,0.));
#34640=DIRECTION('ref_axis',(1.,0.,0.));
#34641=DIRECTION('center_axis',(0.,1.,0.));
#34642=DIRECTION('ref_axis',(1.,0.,0.));
#34643=DIRECTION('center_axis',(0.,1.,0.));
#34644=DIRECTION('ref_axis',(1.,0.,0.));
#34645=DIRECTION('center_axis',(0.,1.,0.));
#34646=DIRECTION('ref_axis',(1.,0.,0.));
#34647=DIRECTION('center_axis',(0.,1.,0.));
#34648=DIRECTION('ref_axis',(1.,0.,0.));
#34649=DIRECTION('center_axis',(0.,1.,0.));
#34650=DIRECTION('ref_axis',(1.,0.,0.));
#34651=DIRECTION('center_axis',(0.,1.,0.));
#34652=DIRECTION('ref_axis',(1.,0.,0.));
#34653=DIRECTION('center_axis',(0.,1.,0.));
#34654=DIRECTION('ref_axis',(1.,0.,0.));
#34655=DIRECTION('center_axis',(0.,1.,0.));
#34656=DIRECTION('ref_axis',(1.,0.,0.));
#34657=DIRECTION('center_axis',(0.,1.,0.));
#34658=DIRECTION('ref_axis',(1.,0.,0.));
#34659=DIRECTION('',(0.707106781186545,0.70710678118655,8.6595605623549E-17));
#34660=DIRECTION('center_axis',(0.,-1.,0.));
#34661=DIRECTION('ref_axis',(1.,0.,0.));
#34662=DIRECTION('center_axis',(-0.0149125533359648,0.,0.999888801693969));
#34663=DIRECTION('ref_axis',(-0.999888801693969,0.,-0.0149125533359648));
#34664=DIRECTION('',(0.,1.,0.));
#34665=DIRECTION('',(-0.999888801693969,0.,-0.0149125533359648));
#34666=DIRECTION('',(0.,-1.,0.));
#34667=DIRECTION('center_axis',(-0.654139811408939,0.,-0.756373655761409));
#34668=DIRECTION('ref_axis',(0.756373655761409,0.,-0.654139811408939));
#34669=DIRECTION('',(0.,-1.,0.));
#34670=DIRECTION('',(0.756373655761409,0.,-0.654139811408939));
#34671=DIRECTION('center_axis',(0.,-1.,0.));
#34672=DIRECTION('ref_axis',(-0.342020143325669,0.,-0.939692620785908));
#34673=DIRECTION('center_axis',(0.,-1.,0.));
#34674=DIRECTION('ref_axis',(1.,0.,0.));
#34675=DIRECTION('center_axis',(0.158942870141262,0.,0.987287781769459));
#34676=DIRECTION('ref_axis',(-0.987287781769459,0.,0.158942870141262));
#34677=DIRECTION('',(0.,1.,0.));
#34678=DIRECTION('',(-0.987287781769459,0.,0.158942870141262));
#34679=DIRECTION('',(0.,-1.,0.));
#34680=DIRECTION('center_axis',(-0.775544864787709,0.,-0.631292454177471));
#34681=DIRECTION('ref_axis',(0.631292454177471,0.,-0.775544864787709));
#34682=DIRECTION('',(0.,-1.,0.));
#34683=DIRECTION('',(0.631292454177471,0.,-0.775544864787709));
#34684=DIRECTION('center_axis',(0.,-1.,0.));
#34685=DIRECTION('ref_axis',(-0.5,0.,-0.866025403784438));
#34686=DIRECTION('center_axis',(0.,-1.,0.));
#34687=DIRECTION('ref_axis',(1.,0.,0.));
#34688=DIRECTION('center_axis',(0.32796889493822,0.,0.944688522187606));
#34689=DIRECTION('ref_axis',(-0.944688522187606,0.,0.32796889493822));
#34690=DIRECTION('',(0.,1.,0.));
#34691=DIRECTION('',(-0.944688522187606,0.,0.32796889493822));
#34692=DIRECTION('',(0.,-1.,0.));
#34693=DIRECTION('center_axis',(-0.873385379894542,0.,-0.487029750822746));
#34694=DIRECTION('ref_axis',(0.487029750822746,0.,-0.873385379894542));
#34695=DIRECTION('',(0.,-1.,0.));
#34696=DIRECTION('',(0.487029750822746,0.,-0.873385379894542));
#34697=DIRECTION('center_axis',(0.,-1.,0.));
#34698=DIRECTION('ref_axis',(-0.64278760968654,0.,-0.766044443118978));
#34699=DIRECTION('center_axis',(0.,-1.,0.));
#34700=DIRECTION('ref_axis',(1.,0.,0.));
#34701=DIRECTION('center_axis',(0.487029750822748,0.,0.873385379894541));
#34702=DIRECTION('ref_axis',(-0.873385379894541,0.,0.487029750822748));
#34703=DIRECTION('',(0.,1.,0.));
#34704=DIRECTION('',(-0.873385379894541,0.,0.487029750822748));
#34705=DIRECTION('',(0.,-1.,0.));
#34706=DIRECTION('center_axis',(-0.944688522187607,0.,-0.327968894938217));
#34707=DIRECTION('ref_axis',(0.327968894938217,0.,-0.944688522187607));
#34708=DIRECTION('',(0.,-1.,0.));
#34709=DIRECTION('',(0.327968894938217,0.,-0.944688522187607));
#34710=DIRECTION('center_axis',(0.,-1.,0.));
#34711=DIRECTION('ref_axis',(-0.766044443118978,0.,-0.642787609686539));
#34712=DIRECTION('center_axis',(0.,-1.,0.));
#34713=DIRECTION('ref_axis',(1.,0.,0.));
#34714=DIRECTION('center_axis',(0.631292454177473,0.,0.775544864787707));
#34715=DIRECTION('ref_axis',(-0.775544864787707,0.,0.631292454177473));
#34716=DIRECTION('',(0.,1.,0.));
#34717=DIRECTION('',(-0.775544864787707,0.,0.631292454177473));
#34718=DIRECTION('',(0.,-1.,0.));
#34719=DIRECTION('center_axis',(-0.987287781769459,0.,-0.158942870141259));
#34720=DIRECTION('ref_axis',(0.158942870141259,0.,-0.987287781769459));
#34721=DIRECTION('',(0.,-1.,0.));
#34722=DIRECTION('',(0.158942870141259,0.,-0.987287781769459));
#34723=DIRECTION('center_axis',(0.,-1.,0.));
#34724=DIRECTION('ref_axis',(-0.866025403784439,0.,-0.5));
#34725=DIRECTION('center_axis',(0.,-1.,0.));
#34726=DIRECTION('ref_axis',(1.,0.,0.));
#34727=DIRECTION('center_axis',(0.756373655761411,0.,0.654139811408936));
#34728=DIRECTION('ref_axis',(-0.654139811408936,0.,0.756373655761411));
#34729=DIRECTION('',(0.,1.,0.));
#34730=DIRECTION('',(-0.654139811408936,0.,0.756373655761411));
#34731=DIRECTION('',(0.,-1.,0.));
#34732=DIRECTION('center_axis',(-0.999888801693969,0.,0.0149125533359685));
#34733=DIRECTION('ref_axis',(-0.0149125533359685,0.,-0.999888801693969));
#34734=DIRECTION('',(0.,-1.,0.));
#34735=DIRECTION('',(-0.0149125533359685,0.,-0.999888801693969));
#34736=DIRECTION('center_axis',(0.,-1.,0.));
#34737=DIRECTION('ref_axis',(-0.939692620785909,0.,-0.342020143325668));
#34738=DIRECTION('center_axis',(0.,-1.,0.));
#34739=DIRECTION('ref_axis',(1.,0.,0.));
#34740=DIRECTION('center_axis',(0.858472826558576,0.,0.512859050871221));
#34741=DIRECTION('ref_axis',(-0.512859050871221,0.,0.858472826558576));
#34742=DIRECTION('',(0.,1.,0.));
#34743=DIRECTION('',(-0.512859050871221,0.,0.858472826558576));
#34744=DIRECTION('',(0.,-1.,0.));
#34745=DIRECTION('center_axis',(-0.982108706347156,0.,0.188314866426198));
#34746=DIRECTION('ref_axis',(-0.188314866426198,0.,-0.982108706347155));
#34747=DIRECTION('',(0.,-1.,0.));
#34748=DIRECTION('',(-0.188314866426198,0.,-0.982108706347155));
#34749=DIRECTION('center_axis',(0.,-1.,0.));
#34750=DIRECTION('ref_axis',(-0.984807753012208,0.,-0.17364817766693));
#34751=DIRECTION('center_axis',(0.,-1.,0.));
#34752=DIRECTION('ref_axis',(1.,0.,0.));
#34753=DIRECTION('center_axis',(0.934487734928969,0.,0.355995327591985));
#34754=DIRECTION('ref_axis',(-0.355995327591985,0.,0.934487734928969));
#34755=DIRECTION('',(0.,1.,0.));
#34756=DIRECTION('',(-0.355995327591985,0.,0.934487734928969));
#34757=DIRECTION('',(0.,-1.,0.));
#34758=DIRECTION('center_axis',(-0.934487734928968,0.,0.355995327591988));
#34759=DIRECTION('ref_axis',(-0.355995327591988,0.,-0.934487734928968));
#34760=DIRECTION('',(0.,-1.,0.));
#34761=DIRECTION('',(-0.355995327591988,0.,-0.934487734928968));
#34762=DIRECTION('center_axis',(0.,-1.,0.));
#34763=DIRECTION('ref_axis',(-1.,0.,1.83697019872103E-16));
#34764=DIRECTION('center_axis',(0.,-1.,0.));
#34765=DIRECTION('ref_axis',(1.,0.,0.));
#34766=DIRECTION('center_axis',(0.982108706347156,0.,0.188314866426195));
#34767=DIRECTION('ref_axis',(-0.188314866426195,0.,0.982108706347156));
#34768=DIRECTION('',(0.,1.,0.));
#34769=DIRECTION('',(-0.188314866426195,0.,0.982108706347156));
#34770=DIRECTION('',(0.,-1.,0.));
#34771=DIRECTION('center_axis',(-0.858472826558574,0.,0.512859050871223));
#34772=DIRECTION('ref_axis',(-0.512859050871223,0.,-0.858472826558574));
#34773=DIRECTION('',(0.,-1.,0.));
#34774=DIRECTION('',(-0.512859050871223,0.,-0.858472826558574));
#34775=DIRECTION('center_axis',(0.,-1.,0.));
#34776=DIRECTION('ref_axis',(-0.984807753012208,0.,0.17364817766693));
#34777=DIRECTION('center_axis',(0.,-1.,0.));
#34778=DIRECTION('ref_axis',(1.,0.,0.));
#34779=DIRECTION('center_axis',(0.999888801693969,0.,0.0149125533359649));
#34780=DIRECTION('ref_axis',(-0.0149125533359649,0.,0.999888801693969));
#34781=DIRECTION('',(0.,1.,0.));
#34782=DIRECTION('',(-0.0149125533359649,0.,0.999888801693969));
#34783=DIRECTION('',(0.,-1.,0.));
#34784=DIRECTION('center_axis',(-0.756373655761409,0.,0.654139811408939));
#34785=DIRECTION('ref_axis',(-0.654139811408939,0.,-0.756373655761409));
#34786=DIRECTION('',(0.,-1.,0.));
#34787=DIRECTION('',(-0.654139811408939,0.,-0.756373655761409));
#34788=DIRECTION('center_axis',(0.,-1.,0.));
#34789=DIRECTION('ref_axis',(-0.939692620785908,0.,0.342020143325669));
#34790=DIRECTION('center_axis',(0.,-1.,0.));
#34791=DIRECTION('ref_axis',(1.,0.,0.));
#34792=DIRECTION('center_axis',(0.987287781769459,0.,-0.158942870141262));
#34793=DIRECTION('ref_axis',(0.158942870141262,0.,0.987287781769459));
#34794=DIRECTION('',(0.,1.,0.));
#34795=DIRECTION('',(0.158942870141262,0.,0.987287781769459));
#34796=DIRECTION('',(0.,-1.,0.));
#34797=DIRECTION('center_axis',(-0.631292454177471,0.,0.775544864787709));
#34798=DIRECTION('ref_axis',(-0.775544864787709,0.,-0.631292454177471));
#34799=DIRECTION('',(0.,-1.,0.));
#34800=DIRECTION('',(-0.775544864787709,0.,-0.631292454177471));
#34801=DIRECTION('center_axis',(0.,-1.,0.));
#34802=DIRECTION('ref_axis',(-0.866025403784438,0.,0.5));
#34803=DIRECTION('center_axis',(0.,-1.,0.));
#34804=DIRECTION('ref_axis',(1.,0.,0.));
#34805=DIRECTION('center_axis',(0.944688522187606,0.,-0.32796889493822));
#34806=DIRECTION('ref_axis',(0.32796889493822,0.,0.944688522187606));
#34807=DIRECTION('',(0.,1.,0.));
#34808=DIRECTION('',(0.32796889493822,0.,0.944688522187606));
#34809=DIRECTION('',(0.,-1.,0.));
#34810=DIRECTION('center_axis',(-0.487029750822746,0.,0.873385379894542));
#34811=DIRECTION('ref_axis',(-0.873385379894542,0.,-0.487029750822746));
#34812=DIRECTION('',(0.,-1.,0.));
#34813=DIRECTION('',(-0.873385379894542,0.,-0.487029750822746));
#34814=DIRECTION('center_axis',(0.,-1.,0.));
#34815=DIRECTION('ref_axis',(-0.766044443118978,0.,0.642787609686539));
#34816=DIRECTION('center_axis',(0.,-1.,0.));
#34817=DIRECTION('ref_axis',(1.,0.,0.));
#34818=DIRECTION('center_axis',(0.873385379894541,0.,-0.487029750822748));
#34819=DIRECTION('ref_axis',(0.487029750822748,0.,0.873385379894541));
#34820=DIRECTION('',(0.,1.,0.));
#34821=DIRECTION('',(0.487029750822748,0.,0.873385379894541));
#34822=DIRECTION('',(0.,-1.,0.));
#34823=DIRECTION('center_axis',(-0.327968894938217,0.,0.944688522187607));
#34824=DIRECTION('ref_axis',(-0.944688522187607,0.,-0.327968894938217));
#34825=DIRECTION('',(0.,-1.,0.));
#34826=DIRECTION('',(-0.944688522187607,0.,-0.327968894938217));
#34827=DIRECTION('center_axis',(0.,-1.,0.));
#34828=DIRECTION('ref_axis',(-0.642787609686539,0.,0.766044443118978));
#34829=DIRECTION('center_axis',(0.,-1.,0.));
#34830=DIRECTION('ref_axis',(1.,0.,0.));
#34831=DIRECTION('center_axis',(0.775544864787707,0.,-0.631292454177473));
#34832=DIRECTION('ref_axis',(0.631292454177473,0.,0.775544864787707));
#34833=DIRECTION('',(0.,1.,0.));
#34834=DIRECTION('',(0.631292454177473,0.,0.775544864787707));
#34835=DIRECTION('',(0.,-1.,0.));
#34836=DIRECTION('center_axis',(-0.158942870141259,0.,0.987287781769459));
#34837=DIRECTION('ref_axis',(-0.987287781769459,0.,-0.158942870141259));
#34838=DIRECTION('',(0.,-1.,0.));
#34839=DIRECTION('',(-0.987287781769459,0.,-0.158942870141259));
#34840=DIRECTION('center_axis',(0.,-1.,0.));
#34841=DIRECTION('ref_axis',(-0.5,0.,0.866025403784439));
#34842=DIRECTION('center_axis',(0.,-1.,0.));
#34843=DIRECTION('ref_axis',(1.,0.,0.));
#34844=DIRECTION('center_axis',(0.654139811408936,0.,-0.756373655761411));
#34845=DIRECTION('ref_axis',(0.756373655761411,0.,0.654139811408936));
#34846=DIRECTION('',(0.,1.,0.));
#34847=DIRECTION('',(0.75637365576141,0.,0.654139811408937));
#34848=DIRECTION('',(0.,-1.,0.));
#34849=DIRECTION('center_axis',(0.014912553335968,0.,0.999888801693969));
#34850=DIRECTION('ref_axis',(-0.999888801693969,0.,0.014912553335968));
#34851=DIRECTION('',(0.,-1.,0.));
#34852=DIRECTION('',(-0.999888801693969,0.,0.014912553335968));
#34853=DIRECTION('center_axis',(0.,-1.,0.));
#34854=DIRECTION('ref_axis',(-0.342020143325669,0.,0.939692620785908));
#34855=DIRECTION('center_axis',(0.,-1.,0.));
#34856=DIRECTION('ref_axis',(1.,0.,0.));
#34857=DIRECTION('center_axis',(0.512859050871221,0.,-0.858472826558576));
#34858=DIRECTION('ref_axis',(0.858472826558576,0.,0.512859050871221));
#34859=DIRECTION('',(0.,1.,0.));
#34860=DIRECTION('',(0.858472826558576,0.,0.512859050871221));
#34861=DIRECTION('',(0.,-1.,0.));
#34862=DIRECTION('center_axis',(0.188314866426198,0.,0.982108706347156));
#34863=DIRECTION('ref_axis',(-0.982108706347156,0.,0.188314866426198));
#34864=DIRECTION('',(0.,-1.,0.));
#34865=DIRECTION('',(-0.982108706347155,0.,0.188314866426198));
#34866=DIRECTION('center_axis',(0.,-1.,0.));
#34867=DIRECTION('ref_axis',(-0.17364817766693,0.,0.984807753012208));
#34868=DIRECTION('center_axis',(0.,-1.,0.));
#34869=DIRECTION('ref_axis',(1.,0.,0.));
#34870=DIRECTION('center_axis',(0.355995327591986,0.,-0.934487734928969));
#34871=DIRECTION('ref_axis',(0.934487734928969,0.,0.355995327591986));
#34872=DIRECTION('',(0.,1.,0.));
#34873=DIRECTION('',(0.934487734928969,0.,0.355995327591986));
#34874=DIRECTION('',(0.,-1.,0.));
#34875=DIRECTION('center_axis',(0.355995327591988,0.,0.934487734928968));
#34876=DIRECTION('ref_axis',(-0.934487734928968,0.,0.355995327591988));
#34877=DIRECTION('',(0.,-1.,0.));
#34878=DIRECTION('',(-0.934487734928968,0.,0.355995327591988));
#34879=DIRECTION('center_axis',(0.,-1.,0.));
#34880=DIRECTION('ref_axis',(1.22464679914735E-16,0.,1.));
#34881=DIRECTION('center_axis',(0.,-1.,0.));
#34882=DIRECTION('ref_axis',(1.,0.,0.));
#34883=DIRECTION('center_axis',(0.,-1.,0.));
#34884=DIRECTION('ref_axis',(1.,0.,0.));
#34885=DIRECTION('center_axis',(0.188314866426195,0.,-0.982108706347156));
#34886=DIRECTION('ref_axis',(0.982108706347156,0.,0.188314866426195));
#34887=DIRECTION('',(0.,1.,0.));
#34888=DIRECTION('',(0.982108706347156,0.,0.188314866426195));
#34889=DIRECTION('',(0.,-1.,0.));
#34890=DIRECTION('center_axis',(0.512859050871224,0.,0.858472826558574));
#34891=DIRECTION('ref_axis',(-0.858472826558574,0.,0.512859050871224));
#34892=DIRECTION('',(0.,-1.,0.));
#34893=DIRECTION('',(-0.858472826558574,0.,0.512859050871224));
#34894=DIRECTION('center_axis',(0.,-1.,0.));
#34895=DIRECTION('ref_axis',(0.173648177666931,0.,0.984807753012208));
#34896=DIRECTION('center_axis',(0.,-1.,0.));
#34897=DIRECTION('ref_axis',(1.,0.,0.));
#34898=DIRECTION('center_axis',(0.0149125533359654,0.,-0.999888801693969));
#34899=DIRECTION('ref_axis',(0.999888801693969,0.,0.0149125533359654));
#34900=DIRECTION('',(0.,1.,0.));
#34901=DIRECTION('',(0.999888801693969,0.,0.0149125533359654));
#34902=DIRECTION('',(0.,-1.,0.));
#34903=DIRECTION('center_axis',(0.654139811408939,0.,0.756373655761409));
#34904=DIRECTION('ref_axis',(-0.756373655761409,0.,0.654139811408939));
#34905=DIRECTION('',(0.,-1.,0.));
#34906=DIRECTION('',(-0.756373655761409,0.,0.654139811408938));
#34907=DIRECTION('center_axis',(0.,-1.,0.));
#34908=DIRECTION('ref_axis',(0.342020143325669,0.,0.939692620785908));
#34909=DIRECTION('center_axis',(0.,-1.,0.));
#34910=DIRECTION('ref_axis',(1.,0.,0.));
#34911=DIRECTION('center_axis',(-0.158942870141261,0.,-0.987287781769459));
#34912=DIRECTION('ref_axis',(0.987287781769459,0.,-0.158942870141261));
#34913=DIRECTION('',(0.,1.,0.));
#34914=DIRECTION('',(0.987287781769459,0.,-0.158942870141261));
#34915=DIRECTION('',(0.,-1.,0.));
#34916=DIRECTION('center_axis',(0.775544864787709,0.,0.631292454177471));
#34917=DIRECTION('ref_axis',(-0.631292454177471,0.,0.775544864787709));
#34918=DIRECTION('',(0.,-1.,0.));
#34919=DIRECTION('',(-0.631292454177471,0.,0.775544864787709));
#34920=DIRECTION('center_axis',(0.,-1.,0.));
#34921=DIRECTION('ref_axis',(0.5,0.,0.866025403784439));
#34922=DIRECTION('center_axis',(0.,-1.,0.));
#34923=DIRECTION('ref_axis',(1.,0.,0.));
#34924=DIRECTION('center_axis',(-0.32796889493822,0.,-0.944688522187606));
#34925=DIRECTION('ref_axis',(0.944688522187606,0.,-0.32796889493822));
#34926=DIRECTION('',(0.,1.,0.));
#34927=DIRECTION('',(0.944688522187606,0.,-0.32796889493822));
#34928=DIRECTION('',(0.,-1.,0.));
#34929=DIRECTION('center_axis',(0.873385379894542,0.,0.487029750822746));
#34930=DIRECTION('ref_axis',(-0.487029750822746,0.,0.873385379894542));
#34931=DIRECTION('',(0.,-1.,0.));
#34932=DIRECTION('',(-0.487029750822746,0.,0.873385379894542));
#34933=DIRECTION('center_axis',(0.,-1.,0.));
#34934=DIRECTION('ref_axis',(0.642787609686539,0.,0.766044443118978));
#34935=DIRECTION('center_axis',(0.,-1.,0.));
#34936=DIRECTION('ref_axis',(1.,0.,0.));
#34937=DIRECTION('center_axis',(-0.487029750822748,0.,-0.873385379894541));
#34938=DIRECTION('ref_axis',(0.873385379894541,0.,-0.487029750822748));
#34939=DIRECTION('',(0.,1.,0.));
#34940=DIRECTION('',(0.873385379894541,0.,-0.487029750822748));
#34941=DIRECTION('',(0.,-1.,0.));
#34942=DIRECTION('center_axis',(0.944688522187607,0.,0.327968894938217));
#34943=DIRECTION('ref_axis',(-0.327968894938217,0.,0.944688522187607));
#34944=DIRECTION('',(0.,-1.,0.));
#34945=DIRECTION('',(-0.327968894938217,0.,0.944688522187607));
#34946=DIRECTION('center_axis',(0.,-1.,0.));
#34947=DIRECTION('ref_axis',(0.766044443118978,0.,0.642787609686539));
#34948=DIRECTION('center_axis',(0.,-1.,0.));
#34949=DIRECTION('ref_axis',(1.,0.,0.));
#34950=DIRECTION('center_axis',(-0.631292454177473,0.,-0.775544864787707));
#34951=DIRECTION('ref_axis',(0.775544864787707,0.,-0.631292454177473));
#34952=DIRECTION('',(0.,1.,0.));
#34953=DIRECTION('',(0.775544864787707,0.,-0.631292454177473));
#34954=DIRECTION('',(0.,-1.,0.));
#34955=DIRECTION('center_axis',(0.987287781769459,0.,0.158942870141259));
#34956=DIRECTION('ref_axis',(-0.158942870141259,0.,0.987287781769459));
#34957=DIRECTION('',(0.,-1.,0.));
#34958=DIRECTION('',(-0.158942870141259,0.,0.987287781769459));
#34959=DIRECTION('center_axis',(0.,-1.,0.));
#34960=DIRECTION('ref_axis',(0.866025403784439,0.,0.5));
#34961=DIRECTION('center_axis',(0.,-1.,0.));
#34962=DIRECTION('ref_axis',(1.,0.,0.));
#34963=DIRECTION('center_axis',(-0.756373655761411,0.,-0.654139811408937));
#34964=DIRECTION('ref_axis',(0.654139811408937,0.,-0.756373655761411));
#34965=DIRECTION('',(0.,1.,0.));
#34966=DIRECTION('',(0.654139811408937,0.,-0.75637365576141));
#34967=DIRECTION('',(0.,-1.,0.));
#34968=DIRECTION('center_axis',(0.999888801693969,0.,-0.014912553335968));
#34969=DIRECTION('ref_axis',(0.014912553335968,0.,0.999888801693969));
#34970=DIRECTION('',(0.,-1.,0.));
#34971=DIRECTION('',(0.014912553335968,0.,0.999888801693969));
#34972=DIRECTION('center_axis',(0.,-1.,0.));
#34973=DIRECTION('ref_axis',(0.939692620785908,0.,0.342020143325669));
#34974=DIRECTION('center_axis',(0.,-1.,0.));
#34975=DIRECTION('ref_axis',(1.,0.,0.));
#34976=DIRECTION('center_axis',(-0.858472826558576,0.,-0.512859050871221));
#34977=DIRECTION('ref_axis',(0.512859050871221,0.,-0.858472826558576));
#34978=DIRECTION('',(0.,1.,0.));
#34979=DIRECTION('',(0.512859050871221,0.,-0.858472826558576));
#34980=DIRECTION('',(0.,-1.,0.));
#34981=DIRECTION('center_axis',(0.982108706347156,0.,-0.188314866426198));
#34982=DIRECTION('ref_axis',(0.188314866426198,0.,0.982108706347155));
#34983=DIRECTION('',(0.,-1.,0.));
#34984=DIRECTION('',(0.188314866426198,0.,0.982108706347156));
#34985=DIRECTION('center_axis',(0.,-1.,0.));
#34986=DIRECTION('ref_axis',(0.984807753012208,0.,0.17364817766693));
#34987=DIRECTION('center_axis',(0.,-1.,0.));
#34988=DIRECTION('ref_axis',(1.,0.,0.));
#34989=DIRECTION('center_axis',(-0.934487734928969,0.,-0.355995327591986));
#34990=DIRECTION('ref_axis',(0.355995327591986,0.,-0.934487734928969));
#34991=DIRECTION('',(0.,1.,0.));
#34992=DIRECTION('',(0.355995327591986,0.,-0.934487734928969));
#34993=DIRECTION('',(0.,-1.,0.));
#34994=DIRECTION('center_axis',(0.934487734928968,0.,-0.355995327591988));
#34995=DIRECTION('ref_axis',(0.355995327591988,0.,0.934487734928968));
#34996=DIRECTION('',(0.,-1.,0.));
#34997=DIRECTION('',(0.355995327591988,0.,0.934487734928968));
#34998=DIRECTION('center_axis',(0.,-1.,0.));
#34999=DIRECTION('ref_axis',(1.,0.,-6.12323399573677E-17));
#35000=DIRECTION('center_axis',(0.,-1.,0.));
#35001=DIRECTION('ref_axis',(1.,0.,0.));
#35002=DIRECTION('center_axis',(-0.982108706347156,0.,-0.188314866426195));
#35003=DIRECTION('ref_axis',(0.188314866426195,0.,-0.982108706347156));
#35004=DIRECTION('',(0.,1.,0.));
#35005=DIRECTION('',(0.188314866426195,0.,-0.982108706347156));
#35006=DIRECTION('',(0.,-1.,0.));
#35007=DIRECTION('center_axis',(0.858472826558574,0.,-0.512859050871223));
#35008=DIRECTION('ref_axis',(0.512859050871223,0.,0.858472826558574));
#35009=DIRECTION('',(0.,-1.,0.));
#35010=DIRECTION('',(0.512859050871223,0.,0.858472826558574));
#35011=DIRECTION('center_axis',(0.,-1.,0.));
#35012=DIRECTION('ref_axis',(0.984807753012208,0.,-0.17364817766693));
#35013=DIRECTION('center_axis',(0.,-1.,0.));
#35014=DIRECTION('ref_axis',(1.,0.,0.));
#35015=DIRECTION('center_axis',(-0.999888801693969,0.,-0.0149125533359654));
#35016=DIRECTION('ref_axis',(0.0149125533359654,0.,-0.999888801693969));
#35017=DIRECTION('',(0.,1.,0.));
#35018=DIRECTION('',(0.0149125533359654,0.,-0.999888801693969));
#35019=DIRECTION('',(0.,-1.,0.));
#35020=DIRECTION('center_axis',(0.756373655761409,0.,-0.654139811408938));
#35021=DIRECTION('ref_axis',(0.654139811408938,0.,0.756373655761409));
#35022=DIRECTION('',(0.,-1.,0.));
#35023=DIRECTION('',(0.654139811408938,0.,0.756373655761409));
#35024=DIRECTION('center_axis',(0.,-1.,0.));
#35025=DIRECTION('ref_axis',(0.939692620785908,0.,-0.342020143325669));
#35026=DIRECTION('center_axis',(0.,-1.,0.));
#35027=DIRECTION('ref_axis',(1.,0.,0.));
#35028=DIRECTION('center_axis',(-0.987287781769459,0.,0.158942870141262));
#35029=DIRECTION('ref_axis',(-0.158942870141262,0.,-0.987287781769459));
#35030=DIRECTION('',(0.,1.,0.));
#35031=DIRECTION('',(-0.158942870141262,0.,-0.987287781769459));
#35032=DIRECTION('',(0.,-1.,0.));
#35033=DIRECTION('center_axis',(0.631292454177471,0.,-0.775544864787709));
#35034=DIRECTION('ref_axis',(0.775544864787709,0.,0.631292454177471));
#35035=DIRECTION('',(0.,-1.,0.));
#35036=DIRECTION('',(0.775544864787709,0.,0.631292454177471));
#35037=DIRECTION('center_axis',(0.,-1.,0.));
#35038=DIRECTION('ref_axis',(0.866025403784439,0.,-0.5));
#35039=DIRECTION('center_axis',(0.,-1.,0.));
#35040=DIRECTION('ref_axis',(1.,0.,0.));
#35041=DIRECTION('center_axis',(-0.944688522187606,0.,0.32796889493822));
#35042=DIRECTION('ref_axis',(-0.32796889493822,0.,-0.944688522187606));
#35043=DIRECTION('',(0.,1.,0.));
#35044=DIRECTION('',(-0.32796889493822,0.,-0.944688522187606));
#35045=DIRECTION('',(0.,-1.,0.));
#35046=DIRECTION('center_axis',(0.487029750822746,0.,-0.873385379894542));
#35047=DIRECTION('ref_axis',(0.873385379894542,0.,0.487029750822746));
#35048=DIRECTION('',(0.,-1.,0.));
#35049=DIRECTION('',(0.873385379894542,0.,0.487029750822746));
#35050=DIRECTION('center_axis',(0.,-1.,0.));
#35051=DIRECTION('ref_axis',(0.766044443118978,0.,-0.642787609686539));
#35052=DIRECTION('center_axis',(0.,-1.,0.));
#35053=DIRECTION('ref_axis',(1.,0.,0.));
#35054=DIRECTION('center_axis',(-0.873385379894541,0.,0.487029750822748));
#35055=DIRECTION('ref_axis',(-0.487029750822748,0.,-0.873385379894541));
#35056=DIRECTION('',(0.,1.,0.));
#35057=DIRECTION('',(-0.487029750822748,0.,-0.873385379894541));
#35058=DIRECTION('',(0.,-1.,0.));
#35059=DIRECTION('center_axis',(0.327968894938217,0.,-0.944688522187607));
#35060=DIRECTION('ref_axis',(0.944688522187607,0.,0.327968894938217));
#35061=DIRECTION('',(0.,-1.,0.));
#35062=DIRECTION('',(0.944688522187607,0.,0.327968894938217));
#35063=DIRECTION('center_axis',(0.,-1.,0.));
#35064=DIRECTION('ref_axis',(0.642787609686539,0.,-0.766044443118978));
#35065=DIRECTION('center_axis',(0.,-1.,0.));
#35066=DIRECTION('ref_axis',(1.,0.,0.));
#35067=DIRECTION('center_axis',(-0.775544864787707,0.,0.631292454177473));
#35068=DIRECTION('ref_axis',(-0.631292454177473,0.,-0.775544864787707));
#35069=DIRECTION('',(0.,1.,0.));
#35070=DIRECTION('',(-0.631292454177473,0.,-0.775544864787707));
#35071=DIRECTION('',(0.,-1.,0.));
#35072=DIRECTION('center_axis',(0.158942870141259,0.,-0.987287781769459));
#35073=DIRECTION('ref_axis',(0.987287781769459,0.,0.158942870141259));
#35074=DIRECTION('',(0.,-1.,0.));
#35075=DIRECTION('',(0.987287781769459,0.,0.158942870141259));
#35076=DIRECTION('center_axis',(0.,-1.,0.));
#35077=DIRECTION('ref_axis',(0.5,0.,-0.866025403784439));
#35078=DIRECTION('center_axis',(0.,-1.,0.));
#35079=DIRECTION('ref_axis',(1.,0.,0.));
#35080=DIRECTION('center_axis',(-0.654139811408937,0.,0.756373655761411));
#35081=DIRECTION('ref_axis',(-0.756373655761411,0.,-0.654139811408937));
#35082=DIRECTION('',(0.,1.,0.));
#35083=DIRECTION('',(-0.75637365576141,0.,-0.654139811408937));
#35084=DIRECTION('',(0.,-1.,0.));
#35085=DIRECTION('center_axis',(-0.014912553335968,0.,-0.999888801693969));
#35086=DIRECTION('ref_axis',(0.999888801693969,0.,-0.014912553335968));
#35087=DIRECTION('',(0.,-1.,0.));
#35088=DIRECTION('',(0.999888801693969,0.,-0.014912553335968));
#35089=DIRECTION('center_axis',(0.,-1.,0.));
#35090=DIRECTION('ref_axis',(0.342020143325669,0.,-0.939692620785908));
#35091=DIRECTION('center_axis',(0.,-1.,0.));
#35092=DIRECTION('ref_axis',(1.,0.,0.));
#35093=DIRECTION('center_axis',(-0.512859050871221,0.,0.858472826558576));
#35094=DIRECTION('ref_axis',(-0.858472826558576,0.,-0.512859050871221));
#35095=DIRECTION('',(0.,1.,0.));
#35096=DIRECTION('',(-0.858472826558576,0.,-0.512859050871221));
#35097=DIRECTION('',(0.,-1.,0.));
#35098=DIRECTION('center_axis',(-0.188314866426198,0.,-0.982108706347156));
#35099=DIRECTION('ref_axis',(0.982108706347156,0.,-0.188314866426198));
#35100=DIRECTION('',(0.,-1.,0.));
#35101=DIRECTION('',(0.982108706347155,0.,-0.188314866426198));
#35102=DIRECTION('center_axis',(0.,-1.,0.));
#35103=DIRECTION('ref_axis',(0.17364817766693,0.,-0.984807753012208));
#35104=DIRECTION('center_axis',(0.,-1.,0.));
#35105=DIRECTION('ref_axis',(1.,0.,0.));
#35106=DIRECTION('center_axis',(-0.355995327591986,0.,0.934487734928969));
#35107=DIRECTION('ref_axis',(-0.934487734928969,0.,-0.355995327591986));
#35108=DIRECTION('',(0.,1.,0.));
#35109=DIRECTION('',(-0.934487734928969,0.,-0.355995327591986));
#35110=DIRECTION('',(0.,-1.,0.));
#35111=DIRECTION('center_axis',(-0.355995327591988,0.,-0.934487734928968));
#35112=DIRECTION('ref_axis',(0.934487734928968,0.,-0.355995327591988));
#35113=DIRECTION('',(0.,-1.,0.));
#35114=DIRECTION('',(0.934487734928968,0.,-0.355995327591988));
#35115=DIRECTION('center_axis',(0.,-1.,0.));
#35116=DIRECTION('ref_axis',(0.,0.,-1.));
#35117=DIRECTION('center_axis',(0.,-1.,0.));
#35118=DIRECTION('ref_axis',(1.,0.,0.));
#35119=DIRECTION('center_axis',(0.,1.,0.));
#35120=DIRECTION('ref_axis',(1.,0.,0.));
#35121=DIRECTION('',(0.,-1.,0.));
#35122=DIRECTION('center_axis',(0.,1.,0.));
#35123=DIRECTION('ref_axis',(1.,0.,0.));
#35124=DIRECTION('',(0.5,0.,-0.866025403784439));
#35125=DIRECTION('',(1.,0.,0.));
#35126=DIRECTION('',(0.5,0.,0.866025403784439));
#35127=DIRECTION('',(-0.5,0.,0.866025403784439));
#35128=DIRECTION('',(-1.,0.,0.));
#35129=DIRECTION('',(-0.5,0.,-0.866025403784439));
#35130=DIRECTION('center_axis',(0.,1.,0.));
#35131=DIRECTION('ref_axis',(0.,0.,1.));
#35132=DIRECTION('',(0.5,0.,-0.866025403784439));
#35133=DIRECTION('center_axis',(0.,-1.,0.));
#35134=DIRECTION('ref_axis',(1.,0.,0.));
#35135=DIRECTION('center_axis',(0.,1.,0.));
#35136=DIRECTION('ref_axis',(0.,0.,1.));
#35137=DIRECTION('',(1.,0.,0.));
#35138=DIRECTION('center_axis',(0.,-1.,0.));
#35139=DIRECTION('ref_axis',(1.,0.,0.));
#35140=DIRECTION('center_axis',(0.,1.,0.));
#35141=DIRECTION('ref_axis',(0.,0.,1.));
#35142=DIRECTION('',(0.5,0.,0.866025403784439));
#35143=DIRECTION('center_axis',(0.,-1.,0.));
#35144=DIRECTION('ref_axis',(1.,0.,0.));
#35145=DIRECTION('center_axis',(0.,1.,0.));
#35146=DIRECTION('ref_axis',(0.,0.,1.));
#35147=DIRECTION('',(-0.5,0.,0.866025403784439));
#35148=DIRECTION('center_axis',(0.,-1.,0.));
#35149=DIRECTION('ref_axis',(1.,0.,0.));
#35150=DIRECTION('center_axis',(0.,1.,0.));
#35151=DIRECTION('ref_axis',(0.,0.,1.));
#35152=DIRECTION('',(-1.,0.,0.));
#35153=DIRECTION('center_axis',(0.,-1.,0.));
#35154=DIRECTION('ref_axis',(1.,0.,0.));
#35155=DIRECTION('center_axis',(0.,1.,0.));
#35156=DIRECTION('ref_axis',(0.,0.,1.));
#35157=DIRECTION('',(-0.5,0.,-0.866025403784439));
#35158=DIRECTION('center_axis',(0.,-1.,0.));
#35159=DIRECTION('ref_axis',(1.,0.,0.));
#35160=DIRECTION('center_axis',(0.,1.,0.));
#35161=DIRECTION('ref_axis',(1.,0.,0.));
#35162=DIRECTION('',(-0.85716730070211,0.515038074910058,1.04972719113862E-16));
#35163=DIRECTION('center_axis',(-0.866025403784439,0.,-0.5));
#35164=DIRECTION('ref_axis',(0.5,0.,-0.866025403784439));
#35165=DIRECTION('',(0.,-1.,0.));
#35166=DIRECTION('',(0.,-1.,0.));
#35167=DIRECTION('center_axis',(-0.866025403784439,0.,0.5));
#35168=DIRECTION('ref_axis',(-0.5,0.,-0.866025403784439));
#35169=DIRECTION('',(0.,-1.,0.));
#35170=DIRECTION('center_axis',(0.,0.,1.));
#35171=DIRECTION('ref_axis',(-1.,0.,0.));
#35172=DIRECTION('',(0.,-1.,0.));
#35173=DIRECTION('center_axis',(0.866025403784439,0.,0.5));
#35174=DIRECTION('ref_axis',(-0.5,0.,0.866025403784439));
#35175=DIRECTION('',(0.,-1.,0.));
#35176=DIRECTION('center_axis',(0.866025403784439,0.,-0.5));
#35177=DIRECTION('ref_axis',(0.5,0.,0.866025403784439));
#35178=DIRECTION('',(0.,-1.,0.));
#35179=DIRECTION('center_axis',(0.,0.,-1.));
#35180=DIRECTION('ref_axis',(1.,0.,0.));
#59383=CARTESIAN_POINT('',(0.,0.,0.));
#59384=CARTESIAN_POINT('Origin',(-17.98,42.93984859951,7.87));
#59385=CARTESIAN_POINT('',(-18.810359785549,40.8943234078509,8.83093840933902));
#59386=CARTESIAN_POINT('',(-18.810359785549,41.063821643627,8.83093840933902));
#59387=CARTESIAN_POINT('',(-18.810359785549,42.93984859951,8.83093840933902));
#59388=CARTESIAN_POINT('',(-18.7697008138552,41.466,6.8753781499502));
#59389=CARTESIAN_POINT('Ctrl Pts',(-18.7697008138552,41.466,6.87537814995019));
#59390=CARTESIAN_POINT('Ctrl Pts',(-18.7662893129558,41.4655640034933,6.87266951748195));
#59391=CARTESIAN_POINT('Ctrl Pts',(-18.7628639760175,41.4651280069866,6.86997851593477));
#59392=CARTESIAN_POINT('Ctrl Pts',(-18.7594249204986,41.4646920104799,6.86730523422837));
#59393=CARTESIAN_POINT('Ctrl Pts',(-18.7203639216068,41.4597399360012,6.83694194023791));
#59394=CARTESIAN_POINT('Ctrl Pts',(-18.6794401066147,41.4547878615226,6.80879775765171));
#59395=CARTESIAN_POINT('Ctrl Pts',(-18.636935323112,41.449835787044,6.78310718962369));
#59396=CARTESIAN_POINT('Ctrl Pts',(-18.5945093211734,41.4448928911128,6.75746423842754));
#59397=CARTESIAN_POINT('Ctrl Pts',(-18.5505086271947,41.4399499951817,6.7342661620788));
#59398=CARTESIAN_POINT('Ctrl Pts',(-18.5052459638554,41.4350070992505,6.71370562681746));
#59399=CARTESIAN_POINT('Ctrl Pts',(-18.4600296773934,41.4300692678927,6.69316615822235));
#59400=CARTESIAN_POINT('Ctrl Pts',(-18.4135544770867,41.4251314365349,6.67525910546274));
#59401=CARTESIAN_POINT('Ctrl Pts',(-18.3661578415816,41.420193605177,6.66013136193015));
#59402=CARTESIAN_POINT('Ctrl Pts',(-18.3187896931452,41.415258741632,6.64501271071101));
#59403=CARTESIAN_POINT('Ctrl Pts',(-18.2705017267598,41.4103238780869,6.63267022523192));
#59404=CARTESIAN_POINT('Ctrl Pts',(-18.2216491507329,41.4053890145419,6.62320182549457));
#59405=CARTESIAN_POINT('Ctrl Pts',(-18.1728052452749,41.400455026858,6.61373510625023));
#59406=CARTESIAN_POINT('Ctrl Pts',(-18.1233974659279,41.3955210391741,6.60714156320865));
#59407=CARTESIAN_POINT('Ctrl Pts',(-18.0737913182603,41.3905870514902,6.60346804674379));
#59408=CARTESIAN_POINT('Ctrl Pts',(-18.0241380309588,41.3856483751461,6.59979103941682));
#59409=CARTESIAN_POINT('Ctrl Pts',(-17.9742865454902,41.3807096988019,6.59903963882925));
#59410=CARTESIAN_POINT('Ctrl Pts',(-17.9246057785493,41.3757710224578,6.60120865378508));
#59411=CARTESIAN_POINT('Ctrl Pts',(-17.874898993866,41.3708297597363,6.60337880465075));
#59412=CARTESIAN_POINT('Ctrl Pts',(-17.8253636504628,41.3658884970149,6.60847236140719));
#59413=CARTESIAN_POINT('Ctrl Pts',(-17.7763634063757,41.3609472342934,6.61643223647977));
#59414=CARTESIAN_POINT('Ctrl Pts',(-17.7272731594248,41.3559968955397,6.62440673212346));
#59415=CARTESIAN_POINT('Ctrl Pts',(-17.6787205076998,41.351046556786,6.63525793527213));
#59416=CARTESIAN_POINT('Ctrl Pts',(-17.6310571840911,41.3460962180323,6.648878011325));
#59417=CARTESIAN_POINT('Ctrl Pts',(-17.607174645919,41.3436157646081,6.65570258757383));
#59418=CARTESIAN_POINT('Ctrl Pts',(-17.5835151218471,41.341135311184,6.66322156449435));
#59419=CARTESIAN_POINT('Ctrl Pts',(-17.5601209284272,41.3386548577598,6.67141685092141));
#59420=CARTESIAN_POINT('Ctrl Pts',(-17.513378656745,41.3336988404369,6.68779126904351));
#59421=CARTESIAN_POINT('Ctrl Pts',(-17.4674961099178,41.3287428231139,6.70693891537748));
#59422=CARTESIAN_POINT('Ctrl Pts',(-17.4228233946656,41.3237868057909,6.72874883112083));
#59423=CARTESIAN_POINT('Ctrl Pts',(-17.3782304368162,41.3188396368011,6.75051980805726));
#59424=CARTESIAN_POINT('Ctrl Pts',(-17.3348435128803,41.3138924678114,6.77494338870558));
#59425=CARTESIAN_POINT('Ctrl Pts',(-17.292994156614,41.3089452988216,6.80186004140209));
#59426=CARTESIAN_POINT('Ctrl Pts',(-17.2511859440286,41.3040029935803,6.82875023132198));
#59427=CARTESIAN_POINT('Ctrl Pts',(-17.2109127631429,41.299060688339,6.85812834631362));
#59428=CARTESIAN_POINT('Ctrl Pts',(-17.1724809489868,41.2941183830976,6.88978931741652));
#59429=CARTESIAN_POINT('Ctrl Pts',(-17.1340707187855,41.2891788535383,6.92143250718429));
#59430=CARTESIAN_POINT('Ctrl Pts',(-17.0975002268711,41.2842393239789,6.95535566624437));
#59431=CARTESIAN_POINT('Ctrl Pts',(-17.0630441374719,41.2792997944195,6.99131237281081));
#59432=CARTESIAN_POINT('Ctrl Pts',(-17.0285928762913,41.2743609570202,7.02726404088209));
#59433=CARTESIAN_POINT('Ctrl Pts',(-16.9962558059207,41.2694221196208,7.06524829586063));
#59434=CARTESIAN_POINT('Ctrl Pts',(-16.9662701561303,41.2644832822215,7.10498248147644));
#59435=CARTESIAN_POINT('Ctrl Pts',(-16.936254577797,41.2595395153907,7.14475632560514));
#59436=CARTESIAN_POINT('Ctrl Pts',(-16.9085954342255,41.2545957485599,7.18628315017448));
#59437=CARTESIAN_POINT('Ctrl Pts',(-16.8834880035964,41.249651981729,7.2292493138958));
#59438=CARTESIAN_POINT('Ctrl Pts',(-16.858366704078,41.244705484051,7.27223921134671));
#59439=CARTESIAN_POINT('Ctrl Pts',(-16.8358001717748,41.2397589863731,7.3166695440082));
#59440=CARTESIAN_POINT('Ctrl Pts',(-16.8159371695144,41.2348124886951,7.36220306550568));
#59441=CARTESIAN_POINT('Ctrl Pts',(-16.7960370638932,41.2298567511406,7.40782164195374));
#59442=CARTESIAN_POINT('Ctrl Pts',(-16.7788507563306,41.2249010135861,7.45454700763435));
#59443=CARTESIAN_POINT('Ctrl Pts',(-16.7644778697622,41.2199452760317,7.50202452404801));
#59444=CARTESIAN_POINT('Ctrl Pts',(-16.7573939362051,41.2175027523677,7.52542466500993));
#59445=CARTESIAN_POINT('Ctrl Pts',(-16.7509926544444,41.2150602287038,7.54900732953798));
#59446=CARTESIAN_POINT('Ctrl Pts',(-16.7452813598676,41.2126177050399,7.57272928211886));
#59447=CARTESIAN_POINT('Ctrl Pts',(-16.7337241625274,41.2076750904343,7.62073228451796));
#59448=CARTESIAN_POINT('Ctrl Pts',(-16.7249444346566,41.2027324758287,7.6695186469948));
#59449=CARTESIAN_POINT('Ctrl Pts',(-16.7190403175229,41.1977898612231,7.71873639179467));
#59450=CARTESIAN_POINT('Ctrl Pts',(-16.7131472161953,41.1928564684676,7.76786230692452));
#59451=CARTESIAN_POINT('Ctrl Pts',(-16.7101191501758,41.1879230757122,7.81741746730105));
#59452=CARTESIAN_POINT('Ctrl Pts',(-16.7100034521229,41.1829896829568,7.86703885491932));
#59453=CARTESIAN_POINT('Ctrl Pts',(-16.7098878732781,41.1780613732669,7.91660911570106));
#59454=CARTESIAN_POINT('Ctrl Pts',(-16.7126787239308,41.173133063577,7.96624492202012));
#59455=CARTESIAN_POINT('Ctrl Pts',(-16.7183714388613,41.1682047538871,8.01557944126555));
#59456=CARTESIAN_POINT('Ctrl Pts',(-16.7240607256338,41.1632794120298,8.06488425121812));
#59457=CARTESIAN_POINT('Ctrl Pts',(-16.7326483523484,41.1583540701725,8.11388758879785));
#59458=CARTESIAN_POINT('Ctrl Pts',(-16.7440778190009,41.1534287283153,8.16222656024821));
#59459=CARTESIAN_POINT('Ctrl Pts',(-16.75550529592,41.1485042439011,8.21055711646151));
#59460=CARTESIAN_POINT('Ctrl Pts',(-16.7697735035174,41.143579759487,8.25822300200199));
#59461=CARTESIAN_POINT('Ctrl Pts',(-16.7867751539815,41.1386552750728,8.30487293183669));
#59462=CARTESIAN_POINT('Ctrl Pts',(-16.8037933529312,41.1337259974324,8.35156826818565));
#59463=CARTESIAN_POINT('Ctrl Pts',(-16.8235501176279,41.1287967197919,8.39724515755078));
#59464=CARTESIAN_POINT('Ctrl Pts',(-16.8458893229295,41.1238674421515,8.44157061869431));
#59465=CARTESIAN_POINT('Ctrl Pts',(-16.8682404570172,41.1189355323538,8.48591974894088));
#59466=CARTESIAN_POINT('Ctrl Pts',(-16.893176501586,41.1140036225562,8.52891553834176));
#59467=CARTESIAN_POINT('Ctrl Pts',(-16.9204962178153,41.1090717127586,8.57025119459823));
#59468=CARTESIAN_POINT('Ctrl Pts',(-16.9478672195076,41.1041305446189,8.61166444749786));
#59469=CARTESIAN_POINT('Ctrl Pts',(-16.9776304941512,41.0991893764792,8.65141090734916));
#59470=CARTESIAN_POINT('Ctrl Pts',(-17.0095434900046,41.0942482083395,8.68921557737121));
#59471=CARTESIAN_POINT('Ctrl Pts',(-17.0260509141496,41.0916923229996,8.70877054881862));
#59472=CARTESIAN_POINT('Ctrl Pts',(-17.0431328973853,41.0891364376597,8.72780655956598));
#59473=CARTESIAN_POINT('Ctrl Pts',(-17.0607521808746,41.0865805523198,8.74628959085061));
#59474=CARTESIAN_POINT('Ctrl Pts',(-17.0948672620246,41.0816317565397,8.78207709109475));
#59475=CARTESIAN_POINT('Ctrl Pts',(-17.1311506442264,41.0766829607596,8.81594838736544));
#59476=CARTESIAN_POINT('Ctrl Pts',(-17.1693586351461,41.0717341649795,8.84763008218228));
#59477=CARTESIAN_POINT('Ctrl Pts',(-17.207496297458,41.0667944783388,8.8792534612009));
#59478=CARTESIAN_POINT('Ctrl Pts',(-17.247551124006,41.0618547916982,8.90869488560116));
#59479=CARTESIAN_POINT('Ctrl Pts',(-17.2892426818714,41.0569151050575,8.93571775224576));
#59480=CARTESIAN_POINT('Ctrl Pts',(-17.3308918826817,41.0519804369527,8.96271316467397));
#59481=CARTESIAN_POINT('Ctrl Pts',(-17.3741740654164,41.047045768848,8.9872945872446));
#59482=CARTESIAN_POINT('Ctrl Pts',(-17.4187775382754,41.0421111007432,9.00926702245602));
#59483=CARTESIAN_POINT('Ctrl Pts',(-17.463354659789,41.0371793479976,9.03122647654302));
#59484=CARTESIAN_POINT('Ctrl Pts',(-17.5092510345198,41.032247595252,9.05057975520432));
#59485=CARTESIAN_POINT('Ctrl Pts',(-17.5561301971801,41.0273158425064,9.06717767697926));
#59486=CARTESIAN_POINT('Ctrl Pts',(-17.6030015944308,41.0223849066926,9.08377284935221));
#59487=CARTESIAN_POINT('Ctrl Pts',(-17.6508549400012,41.0174539708789,9.09761338913787));
#59488=CARTESIAN_POINT('Ctrl Pts',(-17.6993360470047,41.0125230350651,9.1085991060424));
#59489=CARTESIAN_POINT('Ctrl Pts',(-17.7478643829505,41.0075872956712,9.11959552492597));
#59490=CARTESIAN_POINT('Ctrl Pts',(-17.7970211658719,41.0026515562773,9.12773144782443));
#59491=CARTESIAN_POINT('Ctrl Pts',(-17.8464411553264,40.9977158168833,9.13295765368814));
#59492=CARTESIAN_POINT('Ctrl Pts',(-17.895887655359,40.9927774297894,9.13818666306801));
#59493=CARTESIAN_POINT('Ctrl Pts',(-17.9455970953375,40.9878390426955,9.14050282159945));
#59494=CARTESIAN_POINT('Ctrl Pts',(-17.9952018021158,40.9829006556016,9.13990901454098));
#59495=CARTESIAN_POINT('Ctrl Pts',(-18.0448989824159,40.977953062324,9.13931410050226));
#59496=CARTESIAN_POINT('Ctrl Pts',(-18.0944904931126,40.9730054690463,9.13579843234562));
#59497=CARTESIAN_POINT('Ctrl Pts',(-18.1436129898443,40.9680578757686,9.12941684503353));
#59498=CARTESIAN_POINT('Ctrl Pts',(-18.1684823091492,40.965553050379,9.12618602935649));
#59499=CARTESIAN_POINT('Ctrl Pts',(-18.1932315680045,40.9630482249894,9.12222146616022));
#59500=CARTESIAN_POINT('Ctrl Pts',(-18.2178149117059,40.9605433995999,9.11753519700661));
#59501=CARTESIAN_POINT('Ctrl Pts',(-18.266382885828,40.9555947524109,9.10827679010531));
#59502=CARTESIAN_POINT('Ctrl Pts',(-18.3145163539881,40.950646105222,9.09615754486093));
#59503=CARTESIAN_POINT('Ctrl Pts',(-18.3618534959181,40.9456974580331,9.08123404330258));
#59504=CARTESIAN_POINT('Ctrl Pts',(-18.4091054333049,40.9407577181674,9.06633740331808));
#59505=CARTESIAN_POINT('Ctrl Pts',(-18.4555633687124,40.9358179783017,9.04864667986656));
#59506=CARTESIAN_POINT('Ctrl Pts',(-18.5008764485329,40.930878238436,9.02826928016062));
#59507=CARTESIAN_POINT('Ctrl Pts',(-18.5461422178815,40.925943656053,9.0079131560863));
#59508=CARTESIAN_POINT('Ctrl Pts',(-18.5902650016222,40.9210090736699,8.98487613439213));
#59509=CARTESIAN_POINT('Ctrl Pts',(-18.632911998898,40.9160744912869,8.95931442737852));
#59510=CARTESIAN_POINT('Ctrl Pts',(-18.6755365947284,40.9111425009217,8.93376614731687));
#59511=CARTESIAN_POINT('Ctrl Pts',(-18.7166864689408,40.9062105105565,8.90569608701138));
#59512=CARTESIAN_POINT('Ctrl Pts',(-18.7560538356799,40.9012785201913,8.87530614447863));
#59513=CARTESIAN_POINT('Ctrl Pts',(-18.7745591744945,40.8989601494112,8.86102080538415));
#59514=CARTESIAN_POINT('Ctrl Pts',(-18.7926710403453,40.896641778631,8.84622349164109));
#59515=CARTESIAN_POINT('Ctrl Pts',(-18.810359785549,40.8943234078509,8.83093840933902));
#59516=CARTESIAN_POINT('',(-17.1902017145829,41.466,6.87545554732221));
#59517=CARTESIAN_POINT('Origin',(-17.98,41.466,7.87));
#59518=CARTESIAN_POINT('Ctrl Pts',(-17.1902017145829,41.466,6.8754555473222));
#59519=CARTESIAN_POINT('Ctrl Pts',(-17.1488581735048,41.46074845197,6.90828772266504));
#59520=CARTESIAN_POINT('Ctrl Pts',(-17.1095277389328,41.45549690394,6.94373146166701));
#59521=CARTESIAN_POINT('Ctrl Pts',(-17.0725391330082,41.45024535591,6.98150983411271));
#59522=CARTESIAN_POINT('Ctrl Pts',(-17.0369268116997,41.4451892092633,7.0178825360412));
#59523=CARTESIAN_POINT('Ctrl Pts',(-17.0034854613723,41.4401330626166,7.05641875636496));
#59524=CARTESIAN_POINT('Ctrl Pts',(-16.9724723315806,41.43507691597,7.0968324907438));
#59525=CARTESIAN_POINT('Ctrl Pts',(-16.9414666942878,41.4300219908438,7.13723646152047));
#59526=CARTESIAN_POINT('Ctrl Pts',(-16.912888425032,41.4249670657176,7.17951663961273));
#59527=CARTESIAN_POINT('Ctrl Pts',(-16.8869538267822,41.4199121405914,7.22335476247492));
#59528=CARTESIAN_POINT('Ctrl Pts',(-16.8610166860104,41.414856719901,7.26719718304738));
#59529=CARTESIAN_POINT('Ctrl Pts',(-16.8377239906499,41.4098012992106,7.31259740987186));
#59530=CARTESIAN_POINT('Ctrl Pts',(-16.8172469983271,41.4047458785202,7.35921094657329));
#59531=CARTESIAN_POINT('Ctrl Pts',(-16.7967610431176,41.3996882450457,7.40584488626361));
#59532=CARTESIAN_POINT('Ctrl Pts',(-16.7790934417601,41.3946306115713,7.45369272028221));
#59533=CARTESIAN_POINT('Ctrl Pts',(-16.7643672089986,41.3895729780968,7.50239026476135));
#59534=CARTESIAN_POINT('Ctrl Pts',(-16.7496177628025,41.3845073721119,7.55116457274716));
#59535=CARTESIAN_POINT('Ctrl Pts',(-16.7378190830481,41.379441766127,7.60079077170885));
#59536=CARTESIAN_POINT('Ctrl Pts',(-16.7290438642617,41.3743761601421,7.65089101693723));
#59537=CARTESIAN_POINT('Ctrl Pts',(-16.7202606764508,41.3693059539371,7.70103675961648));
#59538=CARTESIAN_POINT('Ctrl Pts',(-16.7145064743903,41.364235747732,7.75165689655593));
#59539=CARTESIAN_POINT('Ctrl Pts',(-16.711802087889,41.3591655415269,7.80236823440583));
#59540=CARTESIAN_POINT('Ctrl Pts',(-16.7090922072103,41.3540850347923,7.85318259639535));
#59541=CARTESIAN_POINT('Ctrl Pts',(-16.7094445054123,41.3490045280577,7.9040880169369));
#59542=CARTESIAN_POINT('Ctrl Pts',(-16.7128277501521,41.3439240213231,7.95470235661039));
#59543=CARTESIAN_POINT('Ctrl Pts',(-16.7137070339155,41.3426036299754,7.96785670118008));
#59544=CARTESIAN_POINT('Ctrl Pts',(-16.7147907711315,41.3412832386277,7.9809914252611));
#59545=CARTESIAN_POINT('Ctrl Pts',(-16.716077846963,41.33996284728,7.99409992369983));
#59546=CARTESIAN_POINT('Ctrl Pts',(-16.7208583168536,41.3350586365668,8.04278763934462));
#59547=CARTESIAN_POINT('Ctrl Pts',(-16.7284689095781,41.3301544258535,8.09132687279746));
#59548=CARTESIAN_POINT('Ctrl Pts',(-16.7388931309886,41.3252502151403,8.13935801397516));
#59549=CARTESIAN_POINT('Ctrl Pts',(-16.7492957772868,41.3203561547196,8.1872897446339));
#59550=CARTESIAN_POINT('Ctrl Pts',(-16.7625003926254,41.3154620942988,8.23471492660863));
#59551=CARTESIAN_POINT('Ctrl Pts',(-16.7784387857867,41.3105680338781,8.28127928284587));
#59552=CARTESIAN_POINT('Ctrl Pts',(-16.7943588359799,41.3056796058692,8.32779004970989));
#59553=CARTESIAN_POINT('Ctrl Pts',(-16.8130062614727,41.3007911778603,8.3734414244914));
#59554=CARTESIAN_POINT('Ctrl Pts',(-16.8342624010277,41.2959027498514,8.4178917359307));
#59555=CARTESIAN_POINT('Ctrl Pts',(-16.8555035418765,41.2910177712033,8.46231068244799));
#59556=CARTESIAN_POINT('Ctrl Pts',(-16.8793495130331,41.2861327925552,8.5055297396731));
#59557=CARTESIAN_POINT('Ctrl Pts',(-16.9056336178924,41.2812478139072,8.54722734513384));
#59558=CARTESIAN_POINT('Ctrl Pts',(-16.9319108774696,41.276364107475,8.58891409110851));
#59559=CARTESIAN_POINT('Ctrl Pts',(-16.9606247132791,41.2714804010429,8.62907969843351));
#59560=CARTESIAN_POINT('Ctrl Pts',(-16.9915639654444,41.2665966946107,8.66742974962811));
#59561=CARTESIAN_POINT('Ctrl Pts',(-17.022531549917,41.2617085159737,8.70581491949443));
#59562=CARTESIAN_POINT('Ctrl Pts',(-17.0557282686084,41.2568203373368,8.74238077681579));
#59563=CARTESIAN_POINT('Ctrl Pts',(-17.0909025557302,41.2519321586998,8.77686588567053));
#59564=CARTESIAN_POINT('Ctrl Pts',(-17.1260939629179,41.2470416008835,8.81136777915358));
#59565=CARTESIAN_POINT('Ctrl Pts',(-17.1632644324539,41.2421510430671,8.84378654025613));
#59566=CARTESIAN_POINT('Ctrl Pts',(-17.2021281422095,41.2372604852507,8.87390008111241));
#59567=CARTESIAN_POINT('Ctrl Pts',(-17.2410661571624,41.2323605769666,8.90407119734194));
#59568=CARTESIAN_POINT('Ctrl Pts',(-17.2817034113001,41.2274606686825,8.93192798131612));
#59569=CARTESIAN_POINT('Ctrl Pts',(-17.3237252953702,41.2225607603984,8.95729182470168));
#59570=CARTESIAN_POINT('Ctrl Pts',(-17.3484102292207,41.2196824051189,8.97219131838266));
#59571=CARTESIAN_POINT('Ctrl Pts',(-17.373572487103,41.2168040498395,8.98623143042253));
#59572=CARTESIAN_POINT('Ctrl Pts',(-17.3991449984387,41.21392569456,8.99938366694457));
#59573=CARTESIAN_POINT('Ctrl Pts',(-17.4431413364607,41.2089736157375,9.02201148930331));
#59574=CARTESIAN_POINT('Ctrl Pts',(-17.4885586565541,41.204021536915,9.04211435978455));
#59575=CARTESIAN_POINT('Ctrl Pts',(-17.5350766527608,41.1990694580926,9.05951385661602));
#59576=CARTESIAN_POINT('Ctrl Pts',(-17.5815084299456,41.1941265577263,9.07688110425956));
#59577=CARTESIAN_POINT('Ctrl Pts',(-17.6290363287014,41.1891836573601,9.09155472662279));
#59578=CARTESIAN_POINT('Ctrl Pts',(-17.6773174249779,41.1842407569939,9.10340312095356));
#59579=CARTESIAN_POINT('Ctrl Pts',(-17.725549052196,41.1793029211487,9.11523937535886));
#59580=CARTESIAN_POINT('Ctrl Pts',(-17.7745318204545,41.1743650853034,9.12425600303587));
#59581=CARTESIAN_POINT('Ctrl Pts',(-17.8239069283246,41.1694272494582,9.13037095847807));
#59582=CARTESIAN_POINT('Ctrl Pts',(-17.8732523604535,41.1644923813825,9.1364822386709));
#59583=CARTESIAN_POINT('Ctrl Pts',(-17.9229891232676,41.1595575133068,9.13969523465749));
#59584=CARTESIAN_POINT('Ctrl Pts',(-17.9727500344444,41.154622645231,9.1399793061304));
#59585=CARTESIAN_POINT('Ctrl Pts',(-18.0225021141912,41.1496886529821,9.14026332718707));
#59586=CARTESIAN_POINT('Ctrl Pts',(-18.0722777871663,41.1447546607332,9.137619453456));
#59587=CARTESIAN_POINT('Ctrl Pts',(-18.1217091818159,41.1398206684844,9.13206913748378));
#59588=CARTESIAN_POINT('Ctrl Pts',(-18.1711875501415,41.1348819875603,9.12651354715616));
#59589=CARTESIAN_POINT('Ctrl Pts',(-18.2203204424377,41.1299433066362,9.11804606179781));
#59590=CARTESIAN_POINT('Ctrl Pts',(-18.2687462450927,41.1250046257122,9.10673991038733));
#59591=CARTESIAN_POINT('Ctrl Pts',(-18.3171974083899,41.1200633583959,9.09542783793383));
#59592=CARTESIAN_POINT('Ctrl Pts',(-18.3649402195001,41.1151220910796,9.08127429396082));
#59593=CARTESIAN_POINT('Ctrl Pts',(-18.4116278165976,41.1101808237633,9.0644025401594));
#59594=CARTESIAN_POINT('Ctrl Pts',(-18.4584011683509,41.105230480446,9.04749979672621));
#59595=CARTESIAN_POINT('Ctrl Pts',(-18.504114934574,41.1002801371287,9.02786909389845));
#59596=CARTESIAN_POINT('Ctrl Pts',(-18.5484433448027,41.0953297938114,9.0056813654144));
#59597=CARTESIAN_POINT('Ctrl Pts',(-18.5706545228201,41.0928493764876,8.99456398979415));
#59598=CARTESIAN_POINT('Ctrl Pts',(-18.5925182992269,41.0903689591638,8.98280535865674));
#59599=CARTESIAN_POINT('Ctrl Pts',(-18.6139964278095,41.08788854184,8.9704310653216));
#59600=CARTESIAN_POINT('Ctrl Pts',(-18.6568995557085,41.0829338428644,8.9457130882606));
#59601=CARTESIAN_POINT('Ctrl Pts',(-18.6984463437109,41.0779791438888,8.9184297097546));
#59602=CARTESIAN_POINT('Ctrl Pts',(-18.7383134522219,41.0730244449132,8.88875448866707));
#59603=CARTESIAN_POINT('Ctrl Pts',(-18.7629963562215,41.0699568444845,8.87038168309808));
#59604=CARTESIAN_POINT('Ctrl Pts',(-18.7870357913132,41.0668892440557,8.85109298601484));
#59605=CARTESIAN_POINT('Ctrl Pts',(-18.810359785549,41.063821643627,8.83093840933902));
#59606=CARTESIAN_POINT('Origin',(-17.98,42.93984859951,7.87));
#59607=CARTESIAN_POINT('',(-18.810359785549,40.1006362902583,8.83093840933902));
#59608=CARTESIAN_POINT('',(-18.8103597856021,40.2713186493562,8.83093840929314));
#59609=CARTESIAN_POINT('',(-18.810359785549,42.93984859951,8.83093840933902));
#59610=CARTESIAN_POINT('',(-19.2499997814169,40.7859014005834,7.87074511808734));
#59611=CARTESIAN_POINT('Ctrl Pts',(-19.2499997814175,40.78590140049,7.87074511714441));
#59612=CARTESIAN_POINT('Ctrl Pts',(-19.2500292717684,40.7809229133116,7.8204808874935));
#59613=CARTESIAN_POINT('Ctrl Pts',(-19.2470703767674,40.7759444261332,7.77021052155451));
#59614=CARTESIAN_POINT('Ctrl Pts',(-19.2411472950103,40.7709659389547,7.72030864992208));
#59615=CARTESIAN_POINT('Ctrl Pts',(-19.234951069999,40.7657578685552,7.6681055506235));
#59616=CARTESIAN_POINT('Ctrl Pts',(-19.2255106220564,40.7605497981556,7.61630639720772));
#59617=CARTESIAN_POINT('Ctrl Pts',(-19.2129139779418,40.755341727756,7.56533112565334));
#59618=CARTESIAN_POINT('Ctrl Pts',(-19.2008516061128,40.7503545517193,7.51651791207196));
#59619=CARTESIAN_POINT('Ctrl Pts',(-19.185895653102,40.7453673756826,7.46846059818919));
#59620=CARTESIAN_POINT('Ctrl Pts',(-19.1681744271675,40.7403801996459,7.42151195040994));
#59621=CARTESIAN_POINT('Ctrl Pts',(-19.1504375370169,40.7353886153248,7.37452180359616));
#59622=CARTESIAN_POINT('Ctrl Pts',(-19.1299307302168,40.7303970310037,7.32864275755956));
#59623=CARTESIAN_POINT('Ctrl Pts',(-19.1068294753863,40.7254054466826,7.28420538291932));
#59624=CARTESIAN_POINT('Ctrl Pts',(-19.0836825292143,40.7204039896431,7.23968011680862));
#59625=CARTESIAN_POINT('Ctrl Pts',(-19.0579311765533,40.7154025326036,7.19660266311589));
#59626=CARTESIAN_POINT('Ctrl Pts',(-19.0297946982172,40.7104010755641,7.15527551350531));
#59627=CARTESIAN_POINT('Ctrl Pts',(-19.0261718104269,40.7097570817627,7.14995417854845));
#59628=CARTESIAN_POINT('Ctrl Pts',(-19.0225094325684,40.7091130879613,7.14466181686219));
#59629=CARTESIAN_POINT('Ctrl Pts',(-19.0188080796698,40.7084690941599,7.13939903256795));
#59630=CARTESIAN_POINT('Ctrl Pts',(-18.9903689402581,40.7035210035561,7.09896272175442));
#59631=CARTESIAN_POINT('Ctrl Pts',(-18.9595023877379,40.6985729129523,7.06010002379334));
#59632=CARTESIAN_POINT('Ctrl Pts',(-18.9264088784134,40.6936248223485,7.02311734292156));
#59633=CARTESIAN_POINT('Ctrl Pts',(-18.8933762760976,40.6886858384669,6.98620272689119));
#59634=CARTESIAN_POINT('Ctrl Pts',(-18.8581252083308,40.6837468545854,6.95116167046038));
#59635=CARTESIAN_POINT('Ctrl Pts',(-18.8208979175303,40.6788078707038,6.91826963256748));
#59636=CARTESIAN_POINT('Ctrl Pts',(-18.7837084376806,40.6738739032409,6.88541100240317));
#59637=CARTESIAN_POINT('Ctrl Pts',(-18.744547117042,40.6689399357781,6.85469743083038));
#59638=CARTESIAN_POINT('Ctrl Pts',(-18.7036932738055,40.6640059683152,6.82636785913397));
#59639=CARTESIAN_POINT('Ctrl Pts',(-18.6628635413039,40.6590749127345,6.79805500671626));
#59640=CARTESIAN_POINT('Ctrl Pts',(-18.6203437144694,40.6541438571539,6.77212367858167));
#59641=CARTESIAN_POINT('Ctrl Pts',(-18.576444394999,40.6492128015733,6.74877117247448));
#59642=CARTESIAN_POINT('Ctrl Pts',(-18.5325523052841,40.6442825580856,6.72542251227902));
#59643=CARTESIAN_POINT('Ctrl Pts',(-18.4872816579289,40.6393523145978,6.70465208730612));
#59644=CARTESIAN_POINT('Ctrl Pts',(-18.4409678318851,40.6344220711101,6.68661136647036));
#59645=CARTESIAN_POINT('Ctrl Pts',(-18.3946087602894,40.6294870110999,6.66855302104083));
#59646=CARTESIAN_POINT('Ctrl Pts',(-18.3472049871667,40.6245519510896,6.65322990253454));
#59647=CARTESIAN_POINT('Ctrl Pts',(-18.2991103659587,40.6196168910793,6.64074470741929));
#59648=CARTESIAN_POINT('Ctrl Pts',(-18.2509898794041,40.6146791769877,6.6282527977507));
#59649=CARTESIAN_POINT('Ctrl Pts',(-18.2021783430207,40.6097414628961,6.61860195709194));
#59650=CARTESIAN_POINT('Ctrl Pts',(-18.1530397230229,40.6048037488044,6.61184370833502));
#59651=CARTESIAN_POINT('Ctrl Pts',(-18.1038093074305,40.5998568105954,6.60507283452957));
#59652=CARTESIAN_POINT('Ctrl Pts',(-18.0542511352957,40.5949098723863,6.6012053802761));
#59653=CARTESIAN_POINT('Ctrl Pts',(-18.0047325749995,40.5899629341773,6.60024084971445));
#59654=CARTESIAN_POINT('Ctrl Pts',(-17.9796043103234,40.5874526032648,6.59975139729304));
#59655=CARTESIAN_POINT('Ctrl Pts',(-17.9544862158352,40.5849422723523,6.60000863318833));
#59656=CARTESIAN_POINT('Ctrl Pts',(-17.9294257401133,40.5824319414398,6.6010073899991));
#59657=CARTESIAN_POINT('Ctrl Pts',(-17.8800299431995,40.5774839190114,6.60297600341003));
#59658=CARTESIAN_POINT('Ctrl Pts',(-17.8306400654593,40.5725358965829,6.60783739216335));
#59659=CARTESIAN_POINT('Ctrl Pts',(-17.7816222424847,40.5675878741545,6.61558927566638));
#59660=CARTESIAN_POINT('Ctrl Pts',(-17.7326946132916,40.562648956187,6.62332689554764));
#59661=CARTESIAN_POINT('Ctrl Pts',(-17.6841382179459,40.5577100382194,6.63394437677166));
#59662=CARTESIAN_POINT('Ctrl Pts',(-17.6363158496529,40.5527711202519,6.64738754922084));
#59663=CARTESIAN_POINT('Ctrl Pts',(-17.5885420400171,40.5478372172436,6.66081707152211));
#59664=CARTESIAN_POINT('Ctrl Pts',(-17.5415013069363,40.5429033142352,6.67706645745127));
#59665=CARTESIAN_POINT('Ctrl Pts',(-17.4955458646341,40.5379694112268,6.69603058356408));
#59666=CARTESIAN_POINT('Ctrl Pts',(-17.4496175294702,40.5330384185156,6.7149835235548));
#59667=CARTESIAN_POINT('Ctrl Pts',(-17.4047737224866,40.5281074258043,6.73664782283407));
#59668=CARTESIAN_POINT('Ctrl Pts',(-17.3613486310191,40.523176433093,6.76086949205333));
#59669=CARTESIAN_POINT('Ctrl Pts',(-17.3179306762151,40.518246250762,6.78508718058086));
#59670=CARTESIAN_POINT('Ctrl Pts',(-17.2759314518796,40.513316068431,6.81186113701932));
#59671=CARTESIAN_POINT('Ctrl Pts',(-17.2356600737474,40.5083858861,6.84099170353868));
#59672=CARTESIAN_POINT('Ctrl Pts',(-17.1953493273036,40.5034508841436,6.87015074738542));
#59673=CARTESIAN_POINT('Ctrl Pts',(-17.1567702437983,40.4985158821873,6.901670678426));
#59674=CARTESIAN_POINT('Ctrl Pts',(-17.1202009765152,40.4935808802309,6.93530986994908));
#59675=CARTESIAN_POINT('Ctrl Pts',(-17.0836120295355,40.4886432225106,6.9689671643529));
#59676=CARTESIAN_POINT('Ctrl Pts',(-17.0490354337303,40.4837055647903,7.0047455958323));
#59677=CARTESIAN_POINT('Ctrl Pts',(-17.0167118280288,40.47876790707,7.04236729297323));
#59678=CARTESIAN_POINT('Ctrl Pts',(-16.9843278164935,40.4738210219344,7.08005929693602));
#59679=CARTESIAN_POINT('Ctrl Pts',(-16.9542055306432,40.4688741367989,7.11960100553891));
#59680=CARTESIAN_POINT('Ctrl Pts',(-16.9265437463089,40.4639272516634,7.16068348280958));
#59681=CARTESIAN_POINT('Ctrl Pts',(-16.9125038431012,40.4614164306822,7.18153513856123));
#59682=CARTESIAN_POINT('Ctrl Pts',(-16.8990970792571,40.458905609701,7.20278328899552));
#59683=CARTESIAN_POINT('Ctrl Pts',(-16.8863448531053,40.4563947887199,7.2243852389616));
#59684=CARTESIAN_POINT('Ctrl Pts',(-16.8612152184356,40.4514469456354,7.26695420726064));
#59685=CARTESIAN_POINT('Ctrl Pts',(-16.8385191063271,40.4464991025508,7.31108675266179));
#59686=CARTESIAN_POINT('Ctrl Pts',(-16.8184531478053,40.4415512594663,7.35647404139954));
#59687=CARTESIAN_POINT('Ctrl Pts',(-16.7984241350082,40.43661252642,7.40177776242349));
#59688=CARTESIAN_POINT('Ctrl Pts',(-16.7810158909585,40.4316737933737,7.4483311476469));
#59689=CARTESIAN_POINT('Ctrl Pts',(-16.7663796379728,40.4267350603274,7.49580003090198));
#59690=CARTESIAN_POINT('Ctrl Pts',(-16.7517582569089,40.4218013455362,7.54322068094346));
#59691=CARTESIAN_POINT('Ctrl Pts',(-16.7399034516814,40.416867630745,7.59155446629698));
#59692=CARTESIAN_POINT('Ctrl Pts',(-16.73091789783,40.4119339159538,7.64044847628775));
#59693=CARTESIAN_POINT('Ctrl Pts',(-16.7219376497172,40.4070031143944,7.6893136156227));
#59694=CARTESIAN_POINT('Ctrl Pts',(-16.7158233955496,40.4020723128349,7.73873778628424));
#59695=CARTESIAN_POINT('Ctrl Pts',(-16.7126269786028,40.3971415112754,7.78835672327441));
#59696=CARTESIAN_POINT('Ctrl Pts',(-16.7094310886601,40.392211522674,7.83796747942134));
#59697=CARTESIAN_POINT('Ctrl Pts',(-16.7091521151252,40.3872815340726,7.8877723914887));
#59698=CARTESIAN_POINT('Ctrl Pts',(-16.711789934967,40.3823515454712,7.93740349359653));
#59699=CARTESIAN_POINT('Ctrl Pts',(-16.7144303323067,40.3774167396208,7.9870830918365));
#59700=CARTESIAN_POINT('Ctrl Pts',(-16.7199931834056,40.3724819337704,8.03658799276528));
#59701=CARTESIAN_POINT('Ctrl Pts',(-16.7284263127276,40.3675471279199,8.08555348600119));
#59702=CARTESIAN_POINT('Ctrl Pts',(-16.7368639777004,40.3626096679472,8.13454531470192));
#59703=CARTESIAN_POINT('Ctrl Pts',(-16.7481748702453,40.3576722079745,8.18299662378046));
#59704=CARTESIAN_POINT('Ctrl Pts',(-16.7622560188676,40.3527347480018,8.23055456787554));
#59705=CARTESIAN_POINT('Ctrl Pts',(-16.7763634825116,40.3477880608439,8.27820138883457));
#59706=CARTESIAN_POINT('Ctrl Pts',(-16.7932513487559,40.342841373686,8.32495099692852));
#59707=CARTESIAN_POINT('Ctrl Pts',(-16.8127678444057,40.3378946865281,8.37046887510291));
#59708=CARTESIAN_POINT('Ctrl Pts',(-16.8226799875669,40.335382336352,8.39358674077668));
#59709=CARTESIAN_POINT('Ctrl Pts',(-16.8332694302267,40.3328699861759,8.41638725639511));
#59710=CARTESIAN_POINT('Ctrl Pts',(-16.8445118559991,40.3303576359998,8.43882921411729));
#59711=CARTESIAN_POINT('Ctrl Pts',(-16.8666532967774,40.3254096778132,8.48302761826214));
#59712=CARTESIAN_POINT('Ctrl Pts',(-16.8914281664316,40.3204617196265,8.52602906244405));
#59713=CARTESIAN_POINT('Ctrl Pts',(-16.9186835779852,40.3155137614398,8.56750086190748));
#59714=CARTESIAN_POINT('Ctrl Pts',(-16.9458888212654,40.3105749108214,8.60889632539012));
#59715=CARTESIAN_POINT('Ctrl Pts',(-16.9755652522928,40.3056360602029,8.64876727415595));
#59716=CARTESIAN_POINT('Ctrl Pts',(-17.0075140777037,40.3006972095844,8.68680544252321));
#59717=CARTESIAN_POINT('Ctrl Pts',(-17.0394304498725,40.2957633757924,8.72480497216521));
#59718=CARTESIAN_POINT('Ctrl Pts',(-17.0736142961015,40.2908295420005,8.76097498935866));
#59719=CARTESIAN_POINT('Ctrl Pts',(-17.1098247504854,40.2858957082085,8.79503785605357));
#59720=CARTESIAN_POINT('Ctrl Pts',(-17.1460138328477,40.2809647864486,8.82908061826942));
#59721=CARTESIAN_POINT('Ctrl Pts',(-17.1842267553722,40.2760338646886,8.86101831898162));
#59722=CARTESIAN_POINT('Ctrl Pts',(-17.2241855496806,40.2711029429287,8.89060987487303));
#59723=CARTESIAN_POINT('Ctrl Pts',(-17.2641377638907,40.2661728331539,8.92019655786101));
#59724=CARTESIAN_POINT('Ctrl Pts',(-17.3058348384027,40.2612427233792,8.94743753785365));
#59725=CARTESIAN_POINT('Ctrl Pts',(-17.3489675178731,40.2563126136045,8.97213338870606));
#59726=CARTESIAN_POINT('Ctrl Pts',(-17.392142347096,40.2513776860695,8.99685337262922));
#59727=CARTESIAN_POINT('Ctrl Pts',(-17.4367551053224,40.2464427585345,9.01902298964242));
#59728=CARTESIAN_POINT('Ctrl Pts',(-17.4824710481861,40.2415078309995,9.03848831492104));
#59729=CARTESIAN_POINT('Ctrl Pts',(-17.5282115825324,40.2365702488724,9.05796411097146));
#59730=CARTESIAN_POINT('Ctrl Pts',(-17.5750559667399,40.2316326667453,9.07473253367482));
#59731=CARTESIAN_POINT('Ctrl Pts',(-17.6226518823375,40.2266950846181,9.08868877191967));
#59732=CARTESIAN_POINT('Ctrl Pts',(-17.6703367367258,40.2217482760148,9.10267108910292));
#59733=CARTESIAN_POINT('Ctrl Pts',(-17.7187753910701,40.2168014674114,9.11383061058746));
#59734=CARTESIAN_POINT('Ctrl Pts',(-17.767604464576,40.2118546588081,9.12211346791413));
#59735=CARTESIAN_POINT('Ctrl Pts',(-17.7923939696334,40.2093432669653,9.12631850230956));
#59736=CARTESIAN_POINT('Ctrl Pts',(-17.817284006811,40.2068318751226,9.12978294105041));
#59737=CARTESIAN_POINT('Ctrl Pts',(-17.8422268232743,40.2043204832799,9.13250487198066));
#59738=CARTESIAN_POINT('Ctrl Pts',(-17.8913534837793,40.1993741174741,9.1378659095734));
#59739=CARTESIAN_POINT('Ctrl Pts',(-17.9409021352363,40.1944277516684,9.14036708668766));
#59740=CARTESIAN_POINT('Ctrl Pts',(-17.9905106969094,40.1894813858626,9.13995650525933));
#59741=CARTESIAN_POINT('Ctrl Pts',(-18.0400449886139,40.18454242536,9.13954653852064));
#59742=CARTESIAN_POINT('Ctrl Pts',(-18.0896384699735,40.1796034648573,9.13623344728117));
#59743=CARTESIAN_POINT('Ctrl Pts',(-18.1389243096997,40.1746645043546,9.13001708868827));
#59744=CARTESIAN_POINT('Ctrl Pts',(-18.1881573429765,40.1697308356146,9.12380739050388));
#59745=CARTESIAN_POINT('Ctrl Pts',(-18.2370828464377,40.1647971668746,9.11470065464772));
#59746=CARTESIAN_POINT('Ctrl Pts',(-18.2853369673953,40.1598634981346,9.10274869147845));
#59747=CARTESIAN_POINT('Ctrl Pts',(-18.3336099836073,40.1549278974782,9.0907920481828));
#59748=CARTESIAN_POINT('Ctrl Pts',(-18.3812105498021,40.1499922968219,9.07598804149137));
#59749=CARTESIAN_POINT('Ctrl Pts',(-18.42778436983,40.1450566961655,9.05843979996295));
#59750=CARTESIAN_POINT('Ctrl Pts',(-18.4743157618438,40.1401255917633,9.04090754460523));
#59751=CARTESIAN_POINT('Ctrl Pts',(-18.5198217640123,40.1351944873612,9.02063624598971));
#59752=CARTESIAN_POINT('Ctrl Pts',(-18.5639669334419,40.130263382959,8.99777773548093));
#59753=CARTESIAN_POINT('Ctrl Pts',(-18.6081724812026,40.1253255341755,8.97488796087836));
#59754=CARTESIAN_POINT('Ctrl Pts',(-18.651012987107,40.1203876853921,8.94940415445937));
#59755=CARTESIAN_POINT('Ctrl Pts',(-18.6921770859854,40.1154498366086,8.92152451145817));
#59756=CARTESIAN_POINT('Ctrl Pts',(-18.7333411848638,40.1105119878252,8.89364486845697));
#59757=CARTESIAN_POINT('Ctrl Pts',(-18.7728284521389,40.1055741390417,8.86336973860931));
#59758=CARTESIAN_POINT('Ctrl Pts',(-18.810359785549,40.1006362902583,8.83093840933902));
#59759=CARTESIAN_POINT('Ctrl Pts',(-18.810359785549,40.8943234078509,8.83093840933902));
#59760=CARTESIAN_POINT('Ctrl Pts',(-18.8483926190765,40.8893386444367,8.79807372708177));
#59761=CARTESIAN_POINT('Ctrl Pts',(-18.8844667877788,40.8843538810224,8.76295164180727));
#59762=CARTESIAN_POINT('Ctrl Pts',(-18.9183146859056,40.8793691176081,8.72584201241465));
#59763=CARTESIAN_POINT('Ctrl Pts',(-18.9518376889585,40.8744322013326,8.68908858640387));
#59764=CARTESIAN_POINT('Ctrl Pts',(-18.9831766720718,40.8694952850571,8.65038607854338));
#59765=CARTESIAN_POINT('Ctrl Pts',(-19.0121121380009,40.8645583687816,8.61003009032823));
#59766=CARTESIAN_POINT('Ctrl Pts',(-19.0414682549524,40.859549681798,8.56908742458229));
#59767=CARTESIAN_POINT('Ctrl Pts',(-19.0683500745277,40.8545409948143,8.52644329266378));
#59768=CARTESIAN_POINT('Ctrl Pts',(-19.0925755837736,40.8495323078307,8.48243413555332));
#59769=CARTESIAN_POINT('Ctrl Pts',(-19.1168010930194,40.8445236208471,8.43842497844286));
#59770=CARTESIAN_POINT('Ctrl Pts',(-19.1383701029171,40.8395149338635,8.39305134970394));
#59771=CARTESIAN_POINT('Ctrl Pts',(-19.157151668176,40.8345062468798,8.34666964462862));
#59772=CARTESIAN_POINT('Ctrl Pts',(-19.177972122364,40.8289538269166,8.29525283498756));
#59773=CARTESIAN_POINT('Ctrl Pts',(-19.1954458292539,40.8234014069534,8.24240611743118));
#59774=CARTESIAN_POINT('Ctrl Pts',(-19.2093998643273,40.8178489869902,8.18855293687549));
#59775=CARTESIAN_POINT('Ctrl Pts',(-19.2232553640092,40.8123357750318,8.13508003659026));
#59776=CARTESIAN_POINT('Ctrl Pts',(-19.2336405829136,40.8068225630735,8.08061511205944));
#59777=CARTESIAN_POINT('Ctrl Pts',(-19.2404326460799,40.8013093511151,8.02559416665144));
#59778=CARTESIAN_POINT('Ctrl Pts',(-19.2467599784388,40.7961733676046,7.97433789889201));
#59779=CARTESIAN_POINT('Ctrl Pts',(-19.249969358089,40.791037384094,7.92259947572652));
#59780=CARTESIAN_POINT('Ctrl Pts',(-19.2499997814169,40.7859014005834,7.87074511808734));
#59781=CARTESIAN_POINT('',(-19.2499999197349,40.9554735995101,7.87045152332722));
#59782=CARTESIAN_POINT('Ctrl Pts',(-18.810359785549,41.063821643627,8.83093840933902));
#59783=CARTESIAN_POINT('Ctrl Pts',(-18.8479499855859,41.0588777342526,8.79845621262589));
#59784=CARTESIAN_POINT('Ctrl Pts',(-18.8836800735341,41.0539338248782,8.76372296388289));
#59785=CARTESIAN_POINT('Ctrl Pts',(-18.9172735335047,41.0489899155038,8.72698210214193));
#59786=CARTESIAN_POINT('Ctrl Pts',(-18.9508427414233,41.044049575275,8.69026776464973));
#59787=CARTESIAN_POINT('Ctrl Pts',(-18.9822780092121,41.0391092350461,8.65154908674822));
#59788=CARTESIAN_POINT('Ctrl Pts',(-19.0113395539479,41.0341688948173,8.61110641912118));
#59789=CARTESIAN_POINT('Ctrl Pts',(-19.040392367812,41.0292300387998,8.57067590156185));
#59790=CARTESIAN_POINT('Ctrl Pts',(-19.0670725549055,41.0242911827824,8.52852286460955));
#59791=CARTESIAN_POINT('Ctrl Pts',(-19.091182129228,41.0193523267649,8.48495875933612));
#59792=CARTESIAN_POINT('Ctrl Pts',(-19.1153130085742,41.0144091064048,8.44135615756007));
#59793=CARTESIAN_POINT('Ctrl Pts',(-19.1368684688677,41.0094658860446,8.39634047332026));
#59794=CARTESIAN_POINT('Ctrl Pts',(-19.1556961153788,41.0045226656845,8.35024852345759));
#59795=CARTESIAN_POINT('Ctrl Pts',(-19.1745314548344,40.9995774255329,8.30413774050222));
#59796=CARTESIAN_POINT('Ctrl Pts',(-19.1906365789394,40.9946321853813,8.25695033198814));
#59797=CARTESIAN_POINT('Ctrl Pts',(-19.2039082916343,40.9896869452297,8.20904054870888));
#59798=CARTESIAN_POINT('Ctrl Pts',(-19.2172064675032,40.9847318445007,8.16103523556413));
#59799=CARTESIAN_POINT('Ctrl Pts',(-19.2276598262009,40.9797767437717,8.11230520480288));
#59800=CARTESIAN_POINT('Ctrl Pts',(-19.235216157106,40.9748216430426,8.06321593862808));
#59801=CARTESIAN_POINT('Ctrl Pts',(-19.241809197014,40.9704982250684,8.02038463663699));
#59802=CARTESIAN_POINT('Ctrl Pts',(-19.2461975587629,40.9661748070942,7.97728021341245));
#59803=CARTESIAN_POINT('Ctrl Pts',(-19.2483789912293,40.96185138912,7.93414619714567));
#59804=CARTESIAN_POINT('Ctrl Pts',(-19.2494516546792,40.95972545925,7.91293615126488));
#59805=CARTESIAN_POINT('Ctrl Pts',(-19.2499923657969,40.95759952938,7.89169848919924));
#59806=CARTESIAN_POINT('Ctrl Pts',(-19.2499999197349,40.9554735995101,7.87045152332722));
#59807=CARTESIAN_POINT('Ctrl Pts',(-19.2499998766701,40.9543644179868,7.87055969442492));
#59808=CARTESIAN_POINT('Ctrl Pts',(-19.250007281152,40.9527258740035,7.85375822096658));
#59809=CARTESIAN_POINT('Ctrl Pts',(-19.2496812724635,40.9511020712888,7.83695686015624));
#59810=CARTESIAN_POINT('Ctrl Pts',(-19.2462699092907,40.9427582088214,7.75008733675439));
#59811=CARTESIAN_POINT('Ctrl Pts',(-19.237717536916,40.9362295709881,7.68034909395144));
#59812=CARTESIAN_POINT('Ctrl Pts',(-19.2140602666449,40.9253330909973,7.56647835519206));
#59813=CARTESIAN_POINT('Ctrl Pts',(-19.202216554662,40.9209996991522,7.52183874183336));
#59814=CARTESIAN_POINT('Ctrl Pts',(-19.1774953312972,40.9133763697255,7.44566946610432));
#59815=CARTESIAN_POINT('Ctrl Pts',(-19.165731729046,40.9101174368386,7.41382976234178));
#59816=CARTESIAN_POINT('Ctrl Pts',(-19.1452338292564,40.9049227256803,7.36452069340626));
#59817=CARTESIAN_POINT('Ctrl Pts',(-19.137346857584,40.9030155713523,7.34671484396063));
#59818=CARTESIAN_POINT('Ctrl Pts',(-19.1213350143937,40.8993056729837,7.31270037717588));
#59819=CARTESIAN_POINT('Ctrl Pts',(-19.1132662153869,40.8975052764277,7.29647050445557));
#59820=CARTESIAN_POINT('Ctrl Pts',(-19.0929460119853,40.8931265728803,7.25770181112711));
#59821=CARTESIAN_POINT('Ctrl Pts',(-19.0803542564405,40.8905367239873,7.23535193864384));
#59822=CARTESIAN_POINT('Ctrl Pts',(-19.0261873612767,40.8798599412999,7.1456707768098));
#59823=CARTESIAN_POINT('Ctrl Pts',(-18.9790474763241,40.8715799850507,7.08192647799003));
#59824=CARTESIAN_POINT('Ctrl Pts',(-18.8943595007561,40.8581880742321,6.98731096414885));
#59825=CARTESIAN_POINT('Ctrl Pts',(-18.8604273929855,40.8531292207383,6.95346233473273));
#59826=CARTESIAN_POINT('Ctrl Pts',(-18.8033411659183,40.8451515924129,6.90261974323977));
#59827=CARTESIAN_POINT('Ctrl Pts',(-18.7813823505824,40.8421960567695,6.88435201438156));
#59828=CARTESIAN_POINT('Ctrl Pts',(-18.7489435810057,40.8380068978013,6.85916755787131));
#59829=CARTESIAN_POINT('Ctrl Pts',(-18.7389498837332,40.8367393093728,6.85164270652434));
#59830=CARTESIAN_POINT('Ctrl Pts',(-18.7205139141966,40.8344446474489,6.83818336616758));
#59831=CARTESIAN_POINT('Ctrl Pts',(-18.7121084929173,40.8334148378287,6.83220252700361));
#59832=CARTESIAN_POINT('Ctrl Pts',(-18.6910604241126,40.8308746016824,6.81760890219221));
#59833=CARTESIAN_POINT('Ctrl Pts',(-18.6783332987314,40.8293721754493,6.80912082099662));
#59834=CARTESIAN_POINT('Ctrl Pts',(-18.5949136776903,40.8197163394275,6.75563802088071));
#59835=CARTESIAN_POINT('Ctrl Pts',(-18.5200556333534,40.8119210932889,6.71749542843296));
#59836=CARTESIAN_POINT('Ctrl Pts',(-18.3976613609614,40.7996096983438,6.669699279121));
#59837=CARTESIAN_POINT('Ctrl Pts',(-18.352417038883,40.7951457148352,6.65490008525363));
#59838=CARTESIAN_POINT('Ctrl Pts',(-18.2729820548916,40.7873232382475,6.63377145556607));
#59839=CARTESIAN_POINT('Ctrl Pts',(-18.2391654813188,40.7839979816903,6.62624267728335));
#59840=CARTESIAN_POINT('Ctrl Pts',(-18.1857077137223,40.7787145261421,6.61661575641215));
#59841=CARTESIAN_POINT('Ctrl Pts',(-18.1662515355845,40.7767862242785,6.61357730622942));
#59842=CARTESIAN_POINT('Ctrl Pts',(-18.1286401191192,40.7730424553114,6.60859632115452));
#59843=CARTESIAN_POINT('Ctrl Pts',(-18.1104980615269,40.771229477806,6.6065906074063));
#59844=CARTESIAN_POINT('Ctrl Pts',(-18.0666762831058,40.7668287232122,6.60269971202443));
#59845=CARTESIAN_POINT('Ctrl Pts',(-18.0409715279906,40.7642295026928,6.60120331651778));
#59846=CARTESIAN_POINT('Ctrl Pts',(-17.942139920233,40.7541555756746,6.59845977091006));
#59847=CARTESIAN_POINT('Ctrl Pts',(-17.8690144642146,40.7465223802064,6.60274861594604));
#59848=CARTESIAN_POINT('Ctrl Pts',(-17.7460325529543,40.7334339939283,6.62068866460258));
#59849=CARTESIAN_POINT('Ctrl Pts',(-17.6958778722398,40.7280265944951,6.63113172465954));
#59850=CARTESIAN_POINT('Ctrl Pts',(-17.6178891172514,40.719589979437,6.65235710478228));
#59851=CARTESIAN_POINT('Ctrl Pts',(-17.5895674321675,40.7165207402653,6.66114047979514));
#59852=CARTESIAN_POINT('Ctrl Pts',(-17.5495570824783,40.7121975221576,6.67510212248155));
#59853=CARTESIAN_POINT('Ctrl Pts',(-17.5376010403528,40.7109073363997,6.67947690003055));
#59854=CARTESIAN_POINT('Ctrl Pts',(-17.5160476616713,40.7085868903455,6.68773297001442));
#59855=CARTESIAN_POINT('Ctrl Pts',(-17.5064293721965,40.7075536293404,6.69155272397297));
#59856=CARTESIAN_POINT('Ctrl Pts',(-17.4827808638863,40.7050171999904,6.70128069411211));
#59857=CARTESIAN_POINT('Ctrl Pts',(-17.468808174912,40.7035218213224,6.70732434393366));
#59858=CARTESIAN_POINT('Ctrl Pts',(-17.3780745486415,40.6938099009134,6.74852182997586));
#59859=CARTESIAN_POINT('Ctrl Pts',(-17.3048593364787,40.6859576526881,6.79101059244738));
#59860=CARTESIAN_POINT('Ctrl Pts',(-17.1981270169557,40.6736195900199,6.86810039523383));
#59861=CARTESIAN_POINT('Ctrl Pts',(-17.161434467363,40.6691886772591,6.89784873872427));
#59862=CARTESIAN_POINT('Ctrl Pts',(-17.1009752694255,40.661417041168,6.95272017823123));
#59863=CARTESIAN_POINT('Ctrl Pts',(-17.0764210128806,40.6581089290884,6.97689793695855));
#59864=CARTESIAN_POINT('Ctrl Pts',(-17.0394582020459,40.6528476076009,7.01638010686075));
#59865=CARTESIAN_POINT('Ctrl Pts',(-17.0263698521508,40.650923917104,7.03102727588699));
#59866=CARTESIAN_POINT('Ctrl Pts',(-17.001797087242,40.6471865283621,7.05984477166056));
#59867=CARTESIAN_POINT('Ctrl Pts',(-16.9902678896433,40.6453752741507,7.07397067030402));
#59868=CARTESIAN_POINT('Ctrl Pts',(-16.9631973777922,40.6409752495249,7.10863569012619));
#59869=CARTESIAN_POINT('Ctrl Pts',(-16.9479698553032,40.6383749734931,7.12940786002853));
#59870=CARTESIAN_POINT('Ctrl Pts',(-16.8897069021195,40.6278930980094,7.21417447723697));
#59871=CARTESIAN_POINT('Ctrl Pts',(-16.851915671158,40.6198314044893,7.28155527115836));
#59872=CARTESIAN_POINT('Ctrl Pts',(-16.800551421224,40.6065601178852,7.39651735041782));
#59873=CARTESIAN_POINT('Ctrl Pts',(-16.7832179507076,40.6014021537742,7.44221741792405));
#59874=CARTESIAN_POINT('Ctrl Pts',(-16.7598888472047,40.5932916840693,7.5163573503009));
#59875=CARTESIAN_POINT('Ctrl Pts',(-16.7521603467498,40.5903016996136,7.5442017044723));
#59876=CARTESIAN_POINT('Ctrl Pts',(-16.7424328183009,40.5860688653072,7.58454186948642));
#59877=CARTESIAN_POINT('Ctrl Pts',(-16.7396604500834,40.5847915379565,7.59683938523784));
#59878=CARTESIAN_POINT('Ctrl Pts',(-16.734948470425,40.5824851121012,7.61929390362714));
#59879=CARTESIAN_POINT('Ctrl Pts',(-16.7329491645861,40.5814531783995,7.62943589092593));
#59880=CARTESIAN_POINT('Ctrl Pts',(-16.7282966901755,40.5789097129878,7.65465576906936));
#59881=CARTESIAN_POINT('Ctrl Pts',(-16.7257918572627,40.5774061670467,7.6697593257701));
#59882=CARTESIAN_POINT('Ctrl Pts',(-16.7113812272796,40.567771734605,7.76758021481907));
#59883=CARTESIAN_POINT('Ctrl Pts',(-16.7073892850552,40.5599971284281,7.85127138567328));
#59884=CARTESIAN_POINT('Ctrl Pts',(-16.7140799847703,40.5477039213984,7.98230784505999));
#59885=CARTESIAN_POINT('Ctrl Pts',(-16.7191790746373,40.5432366545736,8.02967639823069));
#59886=CARTESIAN_POINT('Ctrl Pts',(-16.732558520168,40.535411754879,8.11080842291858));
#59887=CARTESIAN_POINT('Ctrl Pts',(-16.7395867608868,40.5320874869395,8.14472434230894));
#59888=CARTESIAN_POINT('Ctrl Pts',(-16.7527623240707,40.5268085748212,8.19737439431743));
#59889=CARTESIAN_POINT('Ctrl Pts',(-16.7579753712203,40.5248838983516,8.21632644815318));
#59890=CARTESIAN_POINT('Ctrl Pts',(-16.7688567994311,40.521149563144,8.25257439568354));
#59891=CARTESIAN_POINT('Ctrl Pts',(-16.7744613965734,40.5193424201344,8.26988449347853));
#59892=CARTESIAN_POINT('Ctrl Pts',(-16.7888438506188,40.5149617668288,8.31125117182886));
#59893=CARTESIAN_POINT('Ctrl Pts',(-16.7979808072105,40.5123769574935,8.33517303564982));
#59894=CARTESIAN_POINT('Ctrl Pts',(-16.8387002840066,40.5015980456084,8.43282028008869));
#59895=CARTESIAN_POINT('Ctrl Pts',(-16.8765024211767,40.4932057546648,8.50373462868146));
#59896=CARTESIAN_POINT('Ctrl Pts',(-16.9466106994287,40.4798075664947,8.60973526833562));
#59897=CARTESIAN_POINT('Ctrl Pts',(-16.9746459313085,40.4748543221235,8.64740939108677));
#59898=CARTESIAN_POINT('Ctrl Pts',(-17.0227857036458,40.4670154608755,8.70512741450899));
#59899=CARTESIAN_POINT('Ctrl Pts',(-17.0415882024122,40.4640946704907,8.72620130750585));
#59900=CARTESIAN_POINT('Ctrl Pts',(-17.0697104785887,40.4599400032964,8.75568014811557));
#59901=CARTESIAN_POINT('Ctrl Pts',(-17.0784749538847,40.4586732394454,8.76459989653525));
#59902=CARTESIAN_POINT('Ctrl Pts',(-17.0947382606243,40.4563753990957,8.78066950019678));
#59903=CARTESIAN_POINT('Ctrl Pts',(-17.1021945954706,40.455341667552,8.78785890823777));
#59904=CARTESIAN_POINT('Ctrl Pts',(-17.1210118338545,40.452779834005,8.80556341268336));
#59905=CARTESIAN_POINT('Ctrl Pts',(-17.1324785773211,40.4512600069224,8.81596357669802));
#59906=CARTESIAN_POINT('Ctrl Pts',(-17.2058990046647,40.441761216154,8.88014756294862));
#59907=CARTESIAN_POINT('Ctrl Pts',(-17.2727632147549,40.4341229455702,8.9280414485952));
#59908=CARTESIAN_POINT('Ctrl Pts',(-17.385585506634,40.4219097727431,8.99334462576646));
#59909=CARTESIAN_POINT('Ctrl Pts',(-17.4287201947854,40.4173803092128,9.0151295684408));
#59910=CARTESIAN_POINT('Ctrl Pts',(-17.5050174941755,40.409463131924,9.04835140369458));
#59911=CARTESIAN_POINT('Ctrl Pts',(-17.5376055627803,40.4061099569932,9.06096897044695));
#59912=CARTESIAN_POINT('Ctrl Pts',(-17.589335121813,40.4007954550415,9.07858171576351));
#59913=CARTESIAN_POINT('Ctrl Pts',(-17.6081452829912,40.3988647531316,9.08450103913765));
#59914=CARTESIAN_POINT('Ctrl Pts',(-17.6445649901821,40.3951241364239,9.09503652920914));
#59915=CARTESIAN_POINT('Ctrl Pts',(-17.6621510767718,40.3933168252073,9.09971668189172));
#59916=CARTESIAN_POINT('Ctrl Pts',(-17.7046263449102,40.3889447820579,9.11004861315677));
#59917=CARTESIAN_POINT('Ctrl Pts',(-17.7295959201395,40.3863689241327,9.11533078685432));
#59918=CARTESIAN_POINT('Ctrl Pts',(-17.8349655810278,40.3754623995383,9.13432433334843));
#59919=CARTESIAN_POINT('Ctrl Pts',(-17.9164158388159,40.3669255575321,9.14102423373969));
#59920=CARTESIAN_POINT('Ctrl Pts',(-18.0439958587764,40.3534744668979,9.13922307157601));
#59921=CARTESIAN_POINT('Ctrl Pts',(-18.0899966570576,40.3486127246355,9.13606629434577));
#59922=CARTESIAN_POINT('Ctrl Pts',(-18.1634527700716,40.3408955258291,9.12699068055585));
#59923=CARTESIAN_POINT('Ctrl Pts',(-18.1910619369153,40.3380060162458,9.12265067427382));
#59924=CARTESIAN_POINT('Ctrl Pts',(-18.2307555026782,40.3338855507928,9.11506110330259));
#59925=CARTESIAN_POINT('Ctrl Pts',(-18.2429682886803,40.3326224834983,9.11253901264723));
#59926=CARTESIAN_POINT('Ctrl Pts',(-18.2652712994163,40.3303267108203,9.10758956195903));
#59927=CARTESIAN_POINT('Ctrl Pts',(-18.2753714130709,40.3292914290233,9.10521795010416));
#59928=CARTESIAN_POINT('Ctrl Pts',(-18.3005659040645,40.3267180974789,9.09897528751248));
#59929=CARTESIAN_POINT('Ctrl Pts',(-18.3156202671508,40.3251884905972,9.0949497440672));
#59930=CARTESIAN_POINT('Ctrl Pts',(-18.4085159051642,40.3157763919866,9.06826798957341));
#59931=CARTESIAN_POINT('Ctrl Pts',(-18.4841271356515,40.3082250949298,9.03847458477402));
#59932=CARTESIAN_POINT('Ctrl Pts',(-18.599797485842,40.2960638521589,8.9795601897357));
#59933=CARTESIAN_POINT('Ctrl Pts',(-18.6418915187764,40.2914958553629,8.95497546777293));
#59934=CARTESIAN_POINT('Ctrl Pts',(-18.7117228903261,40.2835224210026,8.90861194925388));
#59935=CARTESIAN_POINT('Ctrl Pts',(-18.7401570325403,40.2801522842537,8.8879852474216));
#59936=CARTESIAN_POINT('Ctrl Pts',(-18.7821738962323,40.2749433911493,8.85476272556558));
#59937=CARTESIAN_POINT('Ctrl Pts',(-18.7963979653531,40.2731373371248,8.84300300568812));
#59938=CARTESIAN_POINT('Ctrl Pts',(-18.8103597856021,40.2713186493562,8.83093840929314));
#59939=CARTESIAN_POINT('Origin',(-17.98,42.93984859951,7.87));
#59940=CARTESIAN_POINT('',(-18.8112652832218,39.306728237878,8.83197225855912));
#59941=CARTESIAN_POINT('',(-18.8103598916419,39.4763547317748,8.83093831766272));
#59942=CARTESIAN_POINT('',(-18.810359785549,42.93984859951,8.83093840933902));
#59943=CARTESIAN_POINT('',(-19.2490488064308,39.9921506520735,7.86895363828034));
#59944=CARTESIAN_POINT('Ctrl Pts',(-19.2490122151085,39.9921506232699,7.86895337816756));
#59945=CARTESIAN_POINT('Ctrl Pts',(-19.2500434345316,39.9788491414599,7.73500034620256));
#59946=CARTESIAN_POINT('Ctrl Pts',(-19.1688377106395,39.9235352754098,7.17917982593972));
#59947=CARTESIAN_POINT('Ctrl Pts',(-18.3618920861238,39.8262090251199,6.41823176153347));
#59948=CARTESIAN_POINT('Ctrl Pts',(-16.967275569684,39.7001718723999,6.76191054540271));
#59949=CARTESIAN_POINT('Ctrl Pts',(-16.4998154505205,39.5741347196799,8.12005338135742));
#59950=CARTESIAN_POINT('Ctrl Pts',(-17.3874749649531,39.4480975669599,9.24927045136922));
#59951=CARTESIAN_POINT('Ctrl Pts',(-18.398879038736,39.3589620730259,9.1548465851481));
#59952=CARTESIAN_POINT('Ctrl Pts',(-18.7727866904524,39.311838963332,8.8657852835991));
#59953=CARTESIAN_POINT('Ctrl Pts',(-18.8112652832218,39.306728237878,8.83197225855911));
#59954=CARTESIAN_POINT('Ctrl Pts',(-18.810359785549,40.1006362902583,8.83093840933902));
#59955=CARTESIAN_POINT('Ctrl Pts',(-18.847959120699,40.0956894947554,8.79844831885196));
#59956=CARTESIAN_POINT('Ctrl Pts',(-18.8835950569689,40.0907426992525,8.76379461517207));
#59957=CARTESIAN_POINT('Ctrl Pts',(-18.9170253535683,40.0857959037497,8.72725345538537));
#59958=CARTESIAN_POINT('Ctrl Pts',(-18.9339486021519,40.0832917126864,8.70875541039301));
#59959=CARTESIAN_POINT('Ctrl Pts',(-18.9503072702293,40.0807875216231,8.68977420582005));
#59960=CARTESIAN_POINT('Ctrl Pts',(-18.9660740975914,40.0782833305598,8.67034859533788));
#59961=CARTESIAN_POINT('Ctrl Pts',(-18.9971163167093,40.0733530014636,8.63210285044349));
#59962=CARTESIAN_POINT('Ctrl Pts',(-19.0260027419378,40.0684226723673,8.59195889304783));
#59963=CARTESIAN_POINT('Ctrl Pts',(-19.0524931374539,40.063492343271,8.55019002500348));
#59964=CARTESIAN_POINT('Ctrl Pts',(-19.0789414125603,40.0585698535248,8.50848757053285));
#59965=CARTESIAN_POINT('Ctrl Pts',(-19.1030009068902,40.0536473637785,8.46516578154316));
#59966=CARTESIAN_POINT('Ctrl Pts',(-19.1244721268655,40.0487248740322,8.42053024515274));
#59967=CARTESIAN_POINT('Ctrl Pts',(-19.1459198459749,40.0438077720921,8.3759435636367));
#59968=CARTESIAN_POINT('Ctrl Pts',(-19.1647846613904,40.0388906701519,8.33004647638606));
#59969=CARTESIAN_POINT('Ctrl Pts',(-19.1809122084234,40.0339735682118,8.28317050676398));
#59970=CARTESIAN_POINT('Ctrl Pts',(-19.1970288332318,40.0290597963312,8.23632628343698));
#59971=CARTESIAN_POINT('Ctrl Pts',(-19.2104116848931,40.0241460244506,8.18850501252312));
#59972=CARTESIAN_POINT('Ctrl Pts',(-19.2209549331405,40.01923225257,8.14005713083393));
#59973=CARTESIAN_POINT('Ctrl Pts',(-19.2315006822663,40.0143173151335,8.091597757216));
#59974=CARTESIAN_POINT('Ctrl Pts',(-19.2392053521092,40.009402377697,8.04251201270796));
#59975=CARTESIAN_POINT('Ctrl Pts',(-19.2440138612301,40.0044874402604,7.99316232629432));
#59976=CARTESIAN_POINT('Ctrl Pts',(-19.2480368327339,40.0003754270036,7.95187460546928));
#59977=CARTESIAN_POINT('Ctrl Pts',(-19.2500334984016,39.9962634137468,7.91040250412155));
#59978=CARTESIAN_POINT('Ctrl Pts',(-19.2499995744981,39.99215140049,7.86896039690264));
#59979=CARTESIAN_POINT('Ctrl Pts',(-18.8103597856021,40.2713186493562,8.83093840929314));
#59980=CARTESIAN_POINT('Ctrl Pts',(-18.8113353487289,40.2711915710316,8.83009541209269));
#59981=CARTESIAN_POINT('Ctrl Pts',(-18.8123096314845,40.2710644312613,8.82925092636535));
#59982=CARTESIAN_POINT('Ctrl Pts',(-18.8270029153982,40.2691435575313,8.81647588987751));
#59983=CARTESIAN_POINT('Ctrl Pts',(-18.8404645086,40.2673380063092,8.80425440351711));
#59984=CARTESIAN_POINT('Ctrl Pts',(-18.8721112373488,40.2629773532221,8.77425878974085));
#59985=CARTESIAN_POINT('Ctrl Pts',(-18.8900330129945,40.2604112711266,8.75622011676833));
#59986=CARTESIAN_POINT('Ctrl Pts',(-18.9512887341706,40.2512791113806,8.69074664278821));
#59987=CARTESIAN_POINT('Ctrl Pts',(-18.9915466578312,40.2445956812025,8.64058242508443));
#59988=CARTESIAN_POINT('Ctrl Pts',(-19.0674435395144,40.2304722228324,8.52975837315787));
#59989=CARTESIAN_POINT('Ctrl Pts',(-19.1021991430942,40.2230412192,8.46873574689834));
#59990=CARTESIAN_POINT('Ctrl Pts',(-19.1416774742103,40.2133112943378,8.38377170479687));
#59991=CARTESIAN_POINT('Ctrl Pts',(-19.1510164752077,40.2108821353506,8.36211438849281));
#59992=CARTESIAN_POINT('Ctrl Pts',(-19.1641058645599,40.2072853700062,8.32927317505436));
#59993=CARTESIAN_POINT('Ctrl Pts',(-19.1683119399862,40.2060954771038,8.31827817315408));
#59994=CARTESIAN_POINT('Ctrl Pts',(-19.1759741115113,40.2038629018916,8.29738254012028));
#59995=CARTESIAN_POINT('Ctrl Pts',(-19.1794612974114,40.2028187556447,8.28749553797094));
#59996=CARTESIAN_POINT('Ctrl Pts',(-19.1882986429718,40.2000936577208,8.26141435404993));
#59997=CARTESIAN_POINT('Ctrl Pts',(-19.1934459110803,40.1984238713517,8.24515321351769));
#59998=CARTESIAN_POINT('Ctrl Pts',(-19.216160788911,40.1906177315345,8.16802568509439));
#59999=CARTESIAN_POINT('Ctrl Pts',(-19.2294885616162,40.1846679792351,8.10599530685499));
#60000=CARTESIAN_POINT('Ctrl Pts',(-19.2459963888156,40.1733244437961,7.98609559644813));
#60001=CARTESIAN_POINT('Ctrl Pts',(-19.2499612607445,40.1679420593289,7.92850519690748));
#60002=CARTESIAN_POINT('Ctrl Pts',(-19.2500255463564,40.1588006770076,7.83212210856226));
#60003=CARTESIAN_POINT('Ctrl Pts',(-19.2482801773884,40.155094883314,7.79342073388342));
#60004=CARTESIAN_POINT('Ctrl Pts',(-19.2429290652543,40.1493639202297,7.7346390450327));
#60005=CARTESIAN_POINT('Ctrl Pts',(-19.2406032799203,40.1473784948397,7.71446329122071));
#60006=CARTESIAN_POINT('Ctrl Pts',(-19.2353027391457,40.1436021061938,7.67650644555688));
#60007=CARTESIAN_POINT('Ctrl Pts',(-19.2324310942089,40.1418148587708,7.65871585119259));
#60008=CARTESIAN_POINT('Ctrl Pts',(-19.2248327890104,40.1376064267281,7.61726869868185));
#60009=CARTESIAN_POINT('Ctrl Pts',(-19.219808844847,40.1351763608475,7.59367481668449));
#60010=CARTESIAN_POINT('Ctrl Pts',(-19.1961481691293,40.1249880999119,7.49626335113258));
#60011=CARTESIAN_POINT('Ctrl Pts',(-19.1715684217584,40.1170489948712,7.42406796970317));
#60012=CARTESIAN_POINT('Ctrl Pts',(-19.1106970351154,40.1012526137591,7.28700633499525));
#60013=CARTESIAN_POINT('Ctrl Pts',(-19.0748758555869,40.093430456798,7.22222963867681));
#60014=CARTESIAN_POINT('Ctrl Pts',(-19.0245037562927,40.0841515313849,7.14738072513215));
#60015=CARTESIAN_POINT('Ctrl Pts',(-19.0151242798023,40.082484018365,7.13400779143111));
#60016=CARTESIAN_POINT('Ctrl Pts',(-18.9993705176888,40.0797833684871,7.11244385553752));
#60017=CARTESIAN_POINT('Ctrl Pts',(-18.9931495827782,40.0787410190934,7.104143924455));
#60018=CARTESIAN_POINT('Ctrl Pts',(-18.9794826818378,40.076503372708,7.08636771589139));
#60019=CARTESIAN_POINT('Ctrl Pts',(-18.9720023261264,40.0753104388076,7.07691954059687));
#60020=CARTESIAN_POINT('Ctrl Pts',(-18.9484368262584,40.0716436021589,7.04801004635702));
#60021=CARTESIAN_POINT('Ctrl Pts',(-18.9319037472022,40.0691981711877,7.02891919351889));
#60022=CARTESIAN_POINT('Ctrl Pts',(-18.8884721280407,40.0630454553267,6.98169127715097));
#60023=CARTESIAN_POINT('Ctrl Pts',(-18.8608288661704,40.059374288492,6.95427347200496));
#60024=CARTESIAN_POINT('Ctrl Pts',(-18.7603437351167,40.0466484657817,6.86337625602024));
#60025=CARTESIAN_POINT('Ctrl Pts',(-18.681572567109,40.0376956862913,6.80697566212655));
#60026=CARTESIAN_POINT('Ctrl Pts',(-18.5765124034718,40.0261081354837,6.74855807180531));
#60027=CARTESIAN_POINT('Ctrl Pts',(-18.5555327850923,40.0238117659273,6.7376480729766));
#60028=CARTESIAN_POINT('Ctrl Pts',(-18.5180520475528,40.0197291773038,6.71946768852931));
#60029=CARTESIAN_POINT('Ctrl Pts',(-18.5016772113961,40.0179520638477,6.71195103346215));
#60030=CARTESIAN_POINT('Ctrl Pts',(-18.4664887054554,40.0141425658507,6.69669595059737));
#60031=CARTESIAN_POINT('Ctrl Pts',(-18.4476381662762,40.0121073750776,6.68905627792513));
#60032=CARTESIAN_POINT('Ctrl Pts',(-18.3922052104593,40.0061325635714,6.66812586881319));
#60033=CARTESIAN_POINT('Ctrl Pts',(-18.3551892933437,40.0021545126848,6.65606147057318));
#60034=CARTESIAN_POINT('Ctrl Pts',(-18.2615925230894,39.9921112811397,6.63024554235934));
#60035=CARTESIAN_POINT('Ctrl Pts',(-18.2045118173154,39.9859973451132,6.61864937705951));
#60036=CARTESIAN_POINT('Ctrl Pts',(-18.08478444842,39.9732638633122,6.60278285492688));
#60037=CARTESIAN_POINT('Ctrl Pts',(-18.0221945479173,39.9666573375357,6.59915759520186));
#60038=CARTESIAN_POINT('Ctrl Pts',(-17.9425738396787,39.9584579560645,6.60043756226792));
#60039=CARTESIAN_POINT('Ctrl Pts',(-17.9255669914728,39.9567188288707,6.60105293603353));
#60040=CARTESIAN_POINT('Ctrl Pts',(-17.8981150054009,39.9539361421134,6.60259926183075));
#60041=CARTESIAN_POINT('Ctrl Pts',(-17.8876606452886,39.9528822443823,6.60331800807715));
#60042=CARTESIAN_POINT('Ctrl Pts',(-17.8654678125533,39.9506586344449,6.60512004883764));
#60043=CARTESIAN_POINT('Ctrl Pts',(-17.8537333560946,39.9494907598806,6.60623748780333));
#60044=CARTESIAN_POINT('Ctrl Pts',(-17.8184884581944,39.9460017648623,6.61008962726633));
#60045=CARTESIAN_POINT('Ctrl Pts',(-17.795035416464,39.9437052458999,6.61331846560482));
#60046=CARTESIAN_POINT('Ctrl Pts',(-17.7024090264132,39.9346832097889,6.62872044589387));
#60047=CARTESIAN_POINT('Ctrl Pts',(-17.6342004609265,39.9281416450755,6.64596700181565));
#60048=CARTESIAN_POINT('Ctrl Pts',(-17.5072479134832,39.9155638767811,6.68953460985917));
#60049=CARTESIAN_POINT('Ctrl Pts',(-17.4483984713352,39.9095528034171,6.71484149247598));
#60050=CARTESIAN_POINT('Ctrl Pts',(-17.3691894741759,39.900957648147,6.75624226643411));
#60051=CARTESIAN_POINT('Ctrl Pts',(-17.3470282816727,39.8984945196304,6.76868606601498));
#60052=CARTESIAN_POINT('Ctrl Pts',(-17.3096802008461,39.8942286220278,6.79115717710812));
#60053=CARTESIAN_POINT('Ctrl Pts',(-17.2943075317554,39.8924379255155,6.80086192520758));
#60054=CARTESIAN_POINT('Ctrl Pts',(-17.2626806614534,39.8886757765791,6.82179059744195));
#60055=CARTESIAN_POINT('Ctrl Pts',(-17.2464696052222,39.8867025996206,6.83307038240985));
#60056=CARTESIAN_POINT('Ctrl Pts',(-17.202159545702,39.8811772887929,6.86546073591962));
#60057=CARTESIAN_POINT('Ctrl Pts',(-17.1746665462111,39.87759559835,6.88736459951935));
#60058=CARTESIAN_POINT('Ctrl Pts',(-17.1112712459221,39.8689473234779,6.94232086586985));
#60059=CARTESIAN_POINT('Ctrl Pts',(-17.076297438735,39.8638497311538,6.97635644323875));
#60060=CARTESIAN_POINT('Ctrl Pts',(-16.9886890915822,39.8501998686765,7.07202846990108));
#60061=CARTESIAN_POINT('Ctrl Pts',(-16.9398389321582,39.8416100730414,7.13684021724949));
#60062=CARTESIAN_POINT('Ctrl Pts',(-16.889335823128,39.8316910108919,7.21915841412927));
#60063=CARTESIAN_POINT('Ctrl Pts',(-16.8814268110546,39.8301009339494,7.23259891196903));
#60064=CARTESIAN_POINT('Ctrl Pts',(-16.8686713706722,39.8274772654278,7.25521850665502));
#60065=CARTESIAN_POINT('Ctrl Pts',(-16.8636866044053,39.8264358104254,7.26431687336797));
#60066=CARTESIAN_POINT('Ctrl Pts',(-16.8529636307684,39.8241599085938,7.28447107443897));
#60067=CARTESIAN_POINT('Ctrl Pts',(-16.8472755852718,39.8229284351527,7.29555196365927));
#60068=CARTESIAN_POINT('Ctrl Pts',(-16.8293962487398,39.81897066317,7.33168137585604));
#60069=CARTESIAN_POINT('Ctrl Pts',(-16.8178646186946,39.8162797835117,7.3570500298097));
#60070=CARTESIAN_POINT('Ctrl Pts',(-16.7895901132734,39.8092332896906,7.42511182821588));
#60071=CARTESIAN_POINT('Ctrl Pts',(-16.7743077644469,39.804928644466,7.46836809948586));
#60072=CARTESIAN_POINT('Ctrl Pts',(-16.7382994996124,39.7929442245416,7.59106059757405));
#60073=CARTESIAN_POINT('Ctrl Pts',(-16.7228829887931,39.7852993494336,7.67180385370116));
#60074=CARTESIAN_POINT('Ctrl Pts',(-16.7130191891761,39.7749629706454,7.77884460871983));
#60075=CARTESIAN_POINT('Ctrl Pts',(-16.7114451337938,39.7724926784476,7.80428835767221));
#60076=CARTESIAN_POINT('Ctrl Pts',(-16.7100613401128,39.768218615089,7.84794009257589));
#60077=CARTESIAN_POINT('Ctrl Pts',(-16.7098756875831,39.7664270447809,7.8661290034549));
#60078=CARTESIAN_POINT('Ctrl Pts',(-16.7103029376445,39.7626669647809,7.90403279587781));
#60079=CARTESIAN_POINT('Ctrl Pts',(-16.7109844084988,39.7606967853505,7.92374176402436));
#60080=CARTESIAN_POINT('Ctrl Pts',(-16.7141459314526,39.7551924137859,7.97833340212956));
#60081=CARTESIAN_POINT('Ctrl Pts',(-16.7176080388215,39.7516290519761,8.01313836073583));
#60082=CARTESIAN_POINT('Ctrl Pts',(-16.7292705430451,39.7430414086906,8.09564419373493));
#60083=CARTESIAN_POINT('Ctrl Pts',(-16.7387698433991,39.7379867845643,8.14310454984465));
#60084=CARTESIAN_POINT('Ctrl Pts',(-16.7715699063949,39.724287317659,8.26912084416163));
#60085=CARTESIAN_POINT('Ctrl Pts',(-16.7998015355897,39.7156010564592,8.34616676039986));
#60086=CARTESIAN_POINT('Ctrl Pts',(-16.8419669818062,39.7056022260889,8.43393351215351));
#60087=CARTESIAN_POINT('Ctrl Pts',(-16.8489335326136,39.7040221209275,8.44777926889655));
#60088=CARTESIAN_POINT('Ctrl Pts',(-16.8609783268866,39.7014095719741,8.47066451711307));
#60089=CARTESIAN_POINT('Ctrl Pts',(-16.8659165936715,39.7003694209181,8.47977501629416));
#60090=CARTESIAN_POINT('Ctrl Pts',(-16.8770598819799,39.6980898219277,8.4997455681153));
#60091=CARTESIAN_POINT('Ctrl Pts',(-16.8833147170632,39.6968534438551,8.51057616340708));
#60092=CARTESIAN_POINT('Ctrl Pts',(-16.9041937609624,39.6928569785644,8.54552679796158));
#60093=CARTESIAN_POINT('Ctrl Pts',(-16.9194629556755,39.6901332917146,8.5692546687293));
#60094=CARTESIAN_POINT('Ctrl Pts',(-16.9621572175028,39.6829603224973,8.63097965992323));
#60095=CARTESIAN_POINT('Ctrl Pts',(-16.9909159684543,39.6785643222908,8.66800222151471));
#60096=CARTESIAN_POINT('Ctrl Pts',(-17.0743240718698,39.6666528054053,8.76392011661483));
#60097=CARTESIAN_POINT('Ctrl Pts',(-17.1326070034488,39.6591665509276,8.8193496747899));
#60098=CARTESIAN_POINT('Ctrl Pts',(-17.2158627338382,39.6489899015847,8.8847165841836));
#60099=CARTESIAN_POINT('Ctrl Pts',(-17.2364721786914,39.6465089196388,8.89991342952036));
#60100=CARTESIAN_POINT('Ctrl Pts',(-17.2724971538794,39.6422226017263,8.92483227959429));
#60101=CARTESIAN_POINT('Ctrl Pts',(-17.2876891291906,39.6404296574473,8.93486477429318));
#60102=CARTESIAN_POINT('Ctrl Pts',(-17.3197412875435,39.6366723881534,8.95505562024733));
#60103=CARTESIAN_POINT('Ctrl Pts',(-17.3366323507818,39.6347064731809,8.96515534165965));
#60104=CARTESIAN_POINT('Ctrl Pts',(-17.3839517596869,39.6292320654451,8.99197669001587));
#60105=CARTESIAN_POINT('Ctrl Pts',(-17.41483877871,39.6256949550742,9.00784770893681));
#60106=CARTESIAN_POINT('Ctrl Pts',(-17.4897091674399,39.6171937158938,9.04251858178448));
#60107=CARTESIAN_POINT('Ctrl Pts',(-17.5341791180803,39.6122001798439,9.06013764441958));
#60108=CARTESIAN_POINT('Ctrl Pts',(-17.6584274885196,39.5984287485641,9.10142319171068));
#60109=CARTESIAN_POINT('Ctrl Pts',(-17.7397138757666,39.5896036044402,9.1198308004542));
#60110=CARTESIAN_POINT('Ctrl Pts',(-17.8374630292318,39.5794901834321,9.13206937826961));
#60111=CARTESIAN_POINT('Ctrl Pts',(-17.8527378479838,39.5779245133499,9.13370104336077));
#60112=CARTESIAN_POINT('Ctrl Pts',(-17.8783452606535,39.5753279909192,9.13596735711944));
#60113=CARTESIAN_POINT('Ctrl Pts',(-17.888662094416,39.5742896574515,9.13675351249818));
#60114=CARTESIAN_POINT('Ctrl Pts',(-17.9115455582949,39.5720043823179,9.13821619148546));
#60115=CARTESIAN_POINT('Ctrl Pts',(-17.9241145881642,39.5707606541838,9.13883221383704));
#60116=CARTESIAN_POINT('Ctrl Pts',(-17.9654131052831,39.5667052660875,9.14024135741522));
#60117=CARTESIAN_POINT('Ctrl Pts',(-17.9941632243274,39.5639315296725,9.14024631534447));
#60118=CARTESIAN_POINT('Ctrl Pts',(-18.0712707888497,39.5565619798298,9.13764064319379));
#60119=CARTESIAN_POINT('Ctrl Pts',(-18.1195207317315,39.5520231504256,9.13324105365444));
#60120=CARTESIAN_POINT('Ctrl Pts',(-18.2442319599846,39.5402095655214,9.11463454675975));
#60121=CARTESIAN_POINT('Ctrl Pts',(-18.3198350534797,39.5329568290069,9.09614988885193));
#60122=CARTESIAN_POINT('Ctrl Pts',(-18.4175908919481,39.5230191414013,9.0625081774107));
#60123=CARTESIAN_POINT('Ctrl Pts',(-18.4416494713176,39.5205271433573,9.05340233669953));
#60124=CARTESIAN_POINT('Ctrl Pts',(-18.4822507024794,39.5162282075644,9.03660886190208));
#60125=CARTESIAN_POINT('Ctrl Pts',(-18.4989352741138,39.5144338594558,9.0292834424446));
#60126=CARTESIAN_POINT('Ctrl Pts',(-18.5332624258663,39.5106794599438,9.01332249562221));
#60127=CARTESIAN_POINT('Ctrl Pts',(-18.5508736271378,39.5087178999333,9.0046315840121));
#60128=CARTESIAN_POINT('Ctrl Pts',(-18.5988177209228,39.5032738196776,8.9795730332508));
#60129=CARTESIAN_POINT('Ctrl Pts',(-18.6286940166845,39.4997632343544,8.96237502239997));
#60130=CARTESIAN_POINT('Ctrl Pts',(-18.6977740857092,39.4913486937,8.91877612204459));
#60131=CARTESIAN_POINT('Ctrl Pts',(-18.7362750311286,39.486416251705,8.89136087741531));
#60132=CARTESIAN_POINT('Ctrl Pts',(-18.7857570470864,39.4797536655886,8.85179219470766));
#60133=CARTESIAN_POINT('Ctrl Pts',(-18.7981605331482,39.4780544335529,8.84147994953515));
#60134=CARTESIAN_POINT('Ctrl Pts',(-18.8103598916419,39.4763547317748,8.83093831766273));
#60135=CARTESIAN_POINT('Origin',(-17.98,42.93984859951,7.87));
#60136=CARTESIAN_POINT('',(-18.810359785549,38.5130319987649,8.83093840933902));
#60137=CARTESIAN_POINT('',(-18.8114966369182,38.6825722678645,8.83223897649705));
#60138=CARTESIAN_POINT('',(-18.810359785549,42.93984859951,8.83093840933902));
#60139=CARTESIAN_POINT('',(-19.2502055238694,39.1984014318383,7.8698527011545));
#60140=CARTESIAN_POINT('Ctrl Pts',(-19.2499999914242,39.19840140049,7.86985241131098));
#60141=CARTESIAN_POINT('Ctrl Pts',(-19.2499990709881,39.1976086874999,7.86193206242186));
#60142=CARTESIAN_POINT('Ctrl Pts',(-19.2499240586173,39.1968159745099,7.85401220706734));
#60143=CARTESIAN_POINT('Ctrl Pts',(-19.2497749766161,39.1960232615198,7.84609375061715));
#60144=CARTESIAN_POINT('Ctrl Pts',(-19.2488444410097,39.1910753291281,7.79666856438271));
#60145=CARTESIAN_POINT('Ctrl Pts',(-19.2450217674801,39.1861273967363,7.74718848012828));
#60146=CARTESIAN_POINT('Ctrl Pts',(-19.238301528929,39.1811794643445,7.69801958746717));
#60147=CARTESIAN_POINT('Ctrl Pts',(-19.2315936606194,39.1762406398317,7.64894120217045));
#60148=CARTESIAN_POINT('Ctrl Pts',(-19.2219988793534,39.1713018153188,7.60017341090091));
#60149=CARTESIAN_POINT('Ctrl Pts',(-19.20956370635,39.1663629908059,7.55208005405956));
#60150=CARTESIAN_POINT('Ctrl Pts',(-19.1971411653439,39.1614291832894,7.50403555179797));
#60151=CARTESIAN_POINT('Ctrl Pts',(-19.1818840811064,39.1564953757729,7.45666465568764));
#60152=CARTESIAN_POINT('Ctrl Pts',(-19.163890139538,39.1515615682564,7.41032170216033));
#60153=CARTESIAN_POINT('Ctrl Pts',(-19.1459068187889,39.146630672891,7.36400610229174));
#60154=CARTESIAN_POINT('Ctrl Pts',(-19.1251900388791,39.1416997775257,7.31871775292844));
#60155=CARTESIAN_POINT('Ctrl Pts',(-19.101886720145,39.1367688821604,7.27479399602969));
#60156=CARTESIAN_POINT('Ctrl Pts',(-19.0785872391627,39.131838798849,7.23087747279921));
#60157=CARTESIAN_POINT('Ctrl Pts',(-19.0527023225667,39.1269087155376,7.18832557925812));
#60158=CARTESIAN_POINT('Ctrl Pts',(-19.0244250765477,39.1219786322263,7.14745155215842));
#60159=CARTESIAN_POINT('Ctrl Pts',(-18.9961201969123,39.1170437310472,7.10653758138144));
#60160=CARTESIAN_POINT('Ctrl Pts',(-18.9654186332303,39.1121088298681,7.06730520180628));
#60161=CARTESIAN_POINT('Ctrl Pts',(-18.9325561024963,39.107173928689,7.03003757727084));
#60162=CARTESIAN_POINT('Ctrl Pts',(-18.8996758941321,39.1022363728951,6.99274990548792));
#60163=CARTESIAN_POINT('Ctrl Pts',(-18.8646327902994,39.0972988171013,6.95742948276588));
#60164=CARTESIAN_POINT('Ctrl Pts',(-18.8276995335412,39.0923612613074,6.92432272902744));
#60165=CARTESIAN_POINT('Ctrl Pts',(-18.7906972595141,39.0874144786908,6.89115410861595));
#60166=CARTESIAN_POINT('Ctrl Pts',(-18.7517982119447,39.0824676960742,6.86020775485804));
#60167=CARTESIAN_POINT('Ctrl Pts',(-18.7113070711933,39.0775209134575,6.8316888868828));
#60168=CARTESIAN_POINT('Ctrl Pts',(-18.6907487366439,39.075009311905,6.81720916569135));
#60169=CARTESIAN_POINT('Ctrl Pts',(-18.6697804286997,39.0724977103524,6.80335450224794));
#60170=CARTESIAN_POINT('Ctrl Pts',(-18.6484444243639,39.0699861087999,6.79014720839513));
#60171=CARTESIAN_POINT('Ctrl Pts',(-18.6064118395895,39.0650381764919,6.76412843328754));
#60172=CARTESIAN_POINT('Ctrl Pts',(-18.5627648770544,39.0600902441839,6.74050992054005));
#60173=CARTESIAN_POINT('Ctrl Pts',(-18.5178081895561,39.0551423118759,6.71949474088712));
#60174=CARTESIAN_POINT('Ctrl Pts',(-18.4729342558417,39.050203487448,6.6985182448146));
#60175=CARTESIAN_POINT('Ctrl Pts',(-18.426755871122,39.0452646630201,6.68013580773455));
#60176=CARTESIAN_POINT('Ctrl Pts',(-18.3796039671525,39.0403258385923,6.66450563276471));
#60177=CARTESIAN_POINT('Ctrl Pts',(-18.3324999614159,39.0353920311615,6.64889133536713));
#60178=CARTESIAN_POINT('Ctrl Pts',(-18.2844249118265,39.0304582237306,6.6360239369202));
#60179=CARTESIAN_POINT('Ctrl Pts',(-18.2357295085853,39.0255244162998,6.62601349748531));
#60180=CARTESIAN_POINT('Ctrl Pts',(-18.1870628475282,39.0205935210207,6.61600896665523));
#60181=CARTESIAN_POINT('Ctrl Pts',(-18.1377770939678,39.0156626257416,6.60885816435106));
#60182=CARTESIAN_POINT('Ctrl Pts',(-18.0882353562146,39.0107317304625,6.604620567709));
#60183=CARTESIAN_POINT('Ctrl Pts',(-18.0387017773414,39.0058016472377,6.600383668944));
#60184=CARTESIAN_POINT('Ctrl Pts',(-17.9889128437644,39.0008715640129,6.59905906908673));
#60185=CARTESIAN_POINT('Ctrl Pts',(-17.9392364542431,38.9959414807881,6.60065436805521));
#60186=CARTESIAN_POINT('Ctrl Pts',(-17.8895115190339,38.9910065796955,6.6022512260115));
#60187=CARTESIAN_POINT('Ctrl Pts',(-17.8398998962177,38.9860716786028,6.60677366137129));
#60188=CARTESIAN_POINT('Ctrl Pts',(-17.7907673222606,38.9811367775101,6.61417716469417));
#60189=CARTESIAN_POINT('Ctrl Pts',(-17.7416083185838,38.9761992218028,6.6215846505586));
#60190=CARTESIAN_POINT('Ctrl Pts',(-17.6929294136144,38.9712616660954,6.63187617705311));
#60191=CARTESIAN_POINT('Ctrl Pts',(-17.6450855478346,38.9663241103881,6.6449562008929));
#60192=CARTESIAN_POINT('Ctrl Pts',(-17.597152276093,38.961377327857,6.65806066740873));
#60193=CARTESIAN_POINT('Ctrl Pts',(-17.5500576774657,38.9564305453259,6.67396385609788));
#60194=CARTESIAN_POINT('Ctrl Pts',(-17.5041393928909,38.9514837627948,6.6925210479156));
#60195=CARTESIAN_POINT('Ctrl Pts',(-17.4808255589814,38.9489721605565,6.70194298716862));
#60196=CARTESIAN_POINT('Ctrl Pts',(-17.4578146043481,38.9464605583182,6.71204832976388));
#60197=CARTESIAN_POINT('Ctrl Pts',(-17.4351482004246,38.9439489560799,6.72281365223456));
#60198=CARTESIAN_POINT('Ctrl Pts',(-17.3904946998796,38.9390010237879,6.74402166275233));
#60199=CARTESIAN_POINT('Ctrl Pts',(-17.3469825560467,38.934053091496,6.76788763859601));
#60200=CARTESIAN_POINT('Ctrl Pts',(-17.3049475898042,38.929105159204,6.79426571892089));
#60201=CARTESIAN_POINT('Ctrl Pts',(-17.2629899992104,38.924166334793,6.82059524392954));
#60202=CARTESIAN_POINT('Ctrl Pts',(-17.2225046537098,38.9192275103821,6.84942741328755));
#60203=CARTESIAN_POINT('Ctrl Pts',(-17.1838039252047,38.9142886859711,6.88056995675263));
#60204=CARTESIAN_POINT('Ctrl Pts',(-17.1451425099946,38.9093548785577,6.91168086474088));
#60205=CARTESIAN_POINT('Ctrl Pts',(-17.1082625478236,38.9044210711444,6.94509715880468));
#60206=CARTESIAN_POINT('Ctrl Pts',(-17.0734466738052,38.899487263731,6.98058386187057));
#60207=CARTESIAN_POINT('Ctrl Pts',(-17.0386513496615,38.8945563684698,7.0160496191086));
#60208=CARTESIAN_POINT('Ctrl Pts',(-17.0059180832057,38.8896254732087,7.05358297398715));
#60209=CARTESIAN_POINT('Ctrl Pts',(-16.9754937424663,38.8846945779475,7.09291108708482));
#60210=CARTESIAN_POINT('Ctrl Pts',(-16.9450744122231,38.8797644947411,7.13223272334995));
#60211=CARTESIAN_POINT('Ctrl Pts',(-16.9169635871612,38.8748344115348,7.17334809724056));
#60212=CARTESIAN_POINT('Ctrl Pts',(-16.891367144662,38.8699043283284,7.21595221407101));
#60213=CARTESIAN_POINT('Ctrl Pts',(-16.8657456883327,38.8649694272547,7.25859796528643));
#60214=CARTESIAN_POINT('Ctrl Pts',(-16.8426438024454,38.860034526181,7.30273489305767));
#60215=CARTESIAN_POINT('Ctrl Pts',(-16.822222408586,38.8550996251074,7.34803156338751));
#60216=CARTESIAN_POINT('Ctrl Pts',(-16.8017900295166,38.8501620694193,7.39335259999923));
#60217=CARTESIAN_POINT('Ctrl Pts',(-16.784041209444,38.8452245137313,7.4398341089843));
#60218=CARTESIAN_POINT('Ctrl Pts',(-16.7690881362387,38.8402869580433,7.48712605442254));
#60219=CARTESIAN_POINT('Ctrl Pts',(-16.7541071201858,38.8353401755318,7.53450637444479));
#60220=CARTESIAN_POINT('Ctrl Pts',(-16.7419324125825,38.8303933930204,7.58269962200204));
#60221=CARTESIAN_POINT('Ctrl Pts',(-16.7326255022506,38.8254466105089,7.631343631209));
#60222=CARTESIAN_POINT('Ctrl Pts',(-16.7279001564094,38.8229350081259,7.65604138356838));
#60223=CARTESIAN_POINT('Ctrl Pts',(-16.7239132546785,38.8204234057429,7.68085522387331));
#60224=CARTESIAN_POINT('Ctrl Pts',(-16.7206677123897,38.8179118033599,7.70573743767299));
#60225=CARTESIAN_POINT('Ctrl Pts',(-16.7142738963535,38.812963871038,7.75475614809193));
#60226=CARTESIAN_POINT('Ctrl Pts',(-16.710732251272,38.8080159387161,7.80425714047221));
#60227=CARTESIAN_POINT('Ctrl Pts',(-16.7101023196782,38.8030680063941,7.85387915903438));
#60228=CARTESIAN_POINT('Ctrl Pts',(-16.7094735476278,38.7981291819524,7.90340983612862));
#60229=CARTESIAN_POINT('Ctrl Pts',(-16.7117458658497,38.7931903575107,7.95306055406278));
#60230=CARTESIAN_POINT('Ctrl Pts',(-16.7169271076727,38.788251533069,8.00246459401625));
#60231=CARTESIAN_POINT('Ctrl Pts',(-16.7221030862441,38.7833177256245,8.051818447953));
#60232=CARTESIAN_POINT('Ctrl Pts',(-16.7301820817317,38.7783839181799,8.10092557758484));
#60233=CARTESIAN_POINT('Ctrl Pts',(-16.7411199196841,38.7734501107353,8.14942109189623));
#60234=CARTESIAN_POINT('Ctrl Pts',(-16.7520513016398,38.7685192154425,8.19788798200591));
#60235=CARTESIAN_POINT('Ctrl Pts',(-16.7658380628878,38.7635883201497,8.24574343838036));
#60236=CARTESIAN_POINT('Ctrl Pts',(-16.7823848217199,38.7586574248569,8.2926320914853));
#60237=CARTESIAN_POINT('Ctrl Pts',(-16.7989288555157,38.7537273416186,8.33951302263769));
#60238=CARTESIAN_POINT('Ctrl Pts',(-16.8182318013396,38.7487972583803,8.3854269504489));
#60239=CARTESIAN_POINT('Ctrl Pts',(-16.8401490329719,38.743867175142,8.43003551045009));
#60240=CARTESIAN_POINT('Ctrl Pts',(-16.8620876829688,38.738932274036,8.47468766365754));
#60241=CARTESIAN_POINT('Ctrl Pts',(-16.886645476655,38.7339973729301,8.51803140971679));
#60242=CARTESIAN_POINT('Ctrl Pts',(-16.9136311958668,38.7290624718242,8.55975182027424));
#60243=CARTESIAN_POINT('Ctrl Pts',(-16.9406314314147,38.7241249161037,8.60149467335002));
#60244=CARTESIAN_POINT('Ctrl Pts',(-16.9700618687458,38.7191873603833,8.64161200973613));
#60245=CARTESIAN_POINT('Ctrl Pts',(-17.0016892343157,38.7142498046628,8.67981976127177));
#60246=CARTESIAN_POINT('Ctrl Pts',(-17.0333757020269,38.709303022119,8.71809891173316));
#60247=CARTESIAN_POINT('Ctrl Pts',(-17.0672669180125,38.7043562395752,8.75446095407676));
#60248=CARTESIAN_POINT('Ctrl Pts',(-17.1030919255177,38.6994094570314,8.7886578410419));
#60249=CARTESIAN_POINT('Ctrl Pts',(-17.1212811554622,38.6968978549009,8.80602043448458));
#60250=CARTESIAN_POINT('Ctrl Pts',(-17.1399683433277,38.6943862527704,8.82282552115789));
#60251=CARTESIAN_POINT('Ctrl Pts',(-17.1591149793417,38.6918746506399,8.83904477856231));
#60252=CARTESIAN_POINT('Ctrl Pts',(-17.1968344325165,38.6869267183303,8.87099720716376));
#60253=CARTESIAN_POINT('Ctrl Pts',(-17.2365056878571,38.6819787860206,8.90081470174741));
#60254=CARTESIAN_POINT('Ctrl Pts',(-17.277857497935,38.677030853711,8.92825134386583));
#60255=CARTESIAN_POINT('Ctrl Pts',(-17.3191331898854,38.6720920292818,8.95563748212925));
#60256=CARTESIAN_POINT('Ctrl Pts',(-17.362082848269,38.6671532048526,8.98065115946237));
#60257=CARTESIAN_POINT('Ctrl Pts',(-17.4064025963729,38.6622143804234,9.00308694218593));
#60258=CARTESIAN_POINT('Ctrl Pts',(-17.4506773232259,38.6572805729914,9.02549993400824));
#60259=CARTESIAN_POINT('Ctrl Pts',(-17.4963188979979,38.6523467655594,9.04533996901389));
#60260=CARTESIAN_POINT('Ctrl Pts',(-17.5429967787013,38.6474129581275,9.06244630259586));
#60261=CARTESIAN_POINT('Ctrl Pts',(-17.5896471080499,38.6424820628474,9.0795425392613));
#60262=CARTESIAN_POINT('Ctrl Pts',(-17.6373320180086,38.6375511675673,9.09390808279222));
#60263=CARTESIAN_POINT('Ctrl Pts',(-17.6857011997727,38.6326202722872,9.10543037690709));
#60264=CARTESIAN_POINT('Ctrl Pts',(-17.7340624157598,38.6276901890617,9.11695077344951));
#60265=CARTESIAN_POINT('Ctrl Pts',(-17.7831071468094,38.6227601058361,9.12562872419306));
#60266=CARTESIAN_POINT('Ctrl Pts',(-17.8324726694454,38.6178300226106,9.13140226999139));
#60267=CARTESIAN_POINT('Ctrl Pts',(-17.8818864339751,38.6128951215175,9.13718145792148));
#60268=CARTESIAN_POINT('Ctrl Pts',(-17.9316210705484,38.6079602204243,9.14005051114982));
#60269=CARTESIAN_POINT('Ctrl Pts',(-17.9813082828559,38.6030253193312,9.13999932613997));
#60270=CARTESIAN_POINT('Ctrl Pts',(-18.0310222232361,38.5980877636235,9.13994811359634));
#60271=CARTESIAN_POINT('Ctrl Pts',(-18.0806881409664,38.5931502079159,9.13697356751715));
#60272=CARTESIAN_POINT('Ctrl Pts',(-18.1299408646946,38.5882126522082,9.13111765394615));
#60273=CARTESIAN_POINT('Ctrl Pts',(-18.1792856271185,38.5832658696771,9.1252507974139));
#60274=CARTESIAN_POINT('Ctrl Pts',(-18.2282151147304,38.578319087146,9.11649192337859));
#60275=CARTESIAN_POINT('Ctrl Pts',(-18.2763739880558,38.5733723046148,9.10493419225637));
#60276=CARTESIAN_POINT('Ctrl Pts',(-18.3008254235003,38.5708607023832,9.09906605006564));
#60277=CARTESIAN_POINT('Ctrl Pts',(-18.3250784467569,38.5683491001516,9.09247720781038));
#60278=CARTESIAN_POINT('Ctrl Pts',(-18.3490883789177,38.5658374979199,9.08518466438147));
#60279=CARTESIAN_POINT('Ctrl Pts',(-18.3963731598043,38.5608911881843,9.07082284462152));
#60280=CARTESIAN_POINT('Ctrl Pts',(-18.4429229680734,38.5559448784487,9.0536652596052));
#60281=CARTESIAN_POINT('Ctrl Pts',(-18.4883844413207,38.5509985687131,9.03380636697995));
#60282=CARTESIAN_POINT('Ctrl Pts',(-18.5337803369426,38.5460593939695,9.01397612056713));
#60283=CARTESIAN_POINT('Ctrl Pts',(-18.5780905064593,38.5411202192259,8.99145249459473));
#60284=CARTESIAN_POINT('Ctrl Pts',(-18.6209774872879,38.5361810444823,8.9663794328562));
#60285=CARTESIAN_POINT('Ctrl Pts',(-18.6638174517488,38.5312472844835,8.94133385834727));
#60286=CARTESIAN_POINT('Ctrl Pts',(-18.7052368477543,38.5263135244846,8.9137446606519));
#60287=CARTESIAN_POINT('Ctrl Pts',(-18.7449213816353,38.5213797644858,8.88380238701495));
#60288=CARTESIAN_POINT('Ctrl Pts',(-18.7673030399554,38.5185971759122,8.86691526066286));
#60289=CARTESIAN_POINT('Ctrl Pts',(-18.7891333083039,38.5158145873385,8.84928049341218));
#60290=CARTESIAN_POINT('Ctrl Pts',(-18.810359785549,38.5130319987649,8.83093840933902));
#60291=CARTESIAN_POINT('Ctrl Pts',(-18.8112652832218,39.306728237878,8.83197225855911));
#60292=CARTESIAN_POINT('Ctrl Pts',(-19.0831283208982,39.2706193979584,8.59307288519897));
#60293=CARTESIAN_POINT('Ctrl Pts',(-19.2514866871259,39.2345105580389,8.23122653928661));
#60294=CARTESIAN_POINT('Ctrl Pts',(-19.2520824989184,39.1984017181193,7.86985534807999));
#60295=CARTESIAN_POINT('',(-19.2486386161102,39.3679726942069,7.86909595157452));
#60296=CARTESIAN_POINT('Ctrl Pts',(-18.8103598916419,39.4763547317748,8.83093831766273));
#60297=CARTESIAN_POINT('Ctrl Pts',(-18.8620061132681,39.4691590112148,8.78631011395291));
#60298=CARTESIAN_POINT('Ctrl Pts',(-18.9099933252366,39.4619476178614,8.73757128028793));
#60299=CARTESIAN_POINT('Ctrl Pts',(-18.9636126774288,39.4533741735106,8.67351579312111));
#60300=CARTESIAN_POINT('Ctrl Pts',(-18.9731698682519,39.4518234846111,8.66167241875458));
#60301=CARTESIAN_POINT('Ctrl Pts',(-18.9888542235223,39.4492435241503,8.64150493370748));
#60302=CARTESIAN_POINT('Ctrl Pts',(-18.9950964108587,39.4482070059909,8.63327322898891));
#60303=CARTESIAN_POINT('Ctrl Pts',(-19.0087675185221,39.4459154563924,8.61478037931914));
#60304=CARTESIAN_POINT('Ctrl Pts',(-19.0161445770296,39.4446637927418,8.60448273233148));
#60305=CARTESIAN_POINT('Ctrl Pts',(-19.0400868044573,39.4405436115412,8.56998284764106));
#60306=CARTESIAN_POINT('Ctrl Pts',(-19.0559693654605,39.4377147303983,8.54531502409662));
#60307=CARTESIAN_POINT('Ctrl Pts',(-19.1079695130391,39.4280173732117,8.45805155733503));
#60308=CARTESIAN_POINT('Ctrl Pts',(-19.1395933465726,39.4213072403054,8.39293879686302));
#60309=CARTESIAN_POINT('Ctrl Pts',(-19.1870409289255,39.4088898079164,8.26944492086036));
#60310=CARTESIAN_POINT('Ctrl Pts',(-19.2045684028458,39.4032218674176,8.21195696228121));
#60311=CARTESIAN_POINT('Ctrl Pts',(-19.2230682907053,39.3952176097225,8.13115936753069));
#60312=CARTESIAN_POINT('Ctrl Pts',(-19.2275689638199,39.3929928096936,8.10873523588568));
#60313=CARTESIAN_POINT('Ctrl Pts',(-19.2345113261439,39.388990571676,8.06855040817372));
#60314=CARTESIAN_POINT('Ctrl Pts',(-19.2371870191359,39.3872210676874,8.05083597018949));
#60315=CARTESIAN_POINT('Ctrl Pts',(-19.24165923346,39.3837568503842,8.01629480779699));
#60316=CARTESIAN_POINT('Ctrl Pts',(-19.2434958765408,39.3820638031193,7.99947698992941));
#60317=CARTESIAN_POINT('Ctrl Pts',(-19.246521307358,39.3786278320891,7.96549663107796));
#60318=CARTESIAN_POINT('Ctrl Pts',(-19.2476983593243,39.3768849072122,7.94833661507711));
#60319=CARTESIAN_POINT('Ctrl Pts',(-19.2495244548045,39.3730190528955,7.91046075630686));
#60320=CARTESIAN_POINT('Ctrl Pts',(-19.2500155520902,39.3708920262909,7.88974282348426));
#60321=CARTESIAN_POINT('Ctrl Pts',(-19.2499996247524,39.3687519858842,7.86902371692696));
#60322=CARTESIAN_POINT('Ctrl Pts',(-19.2486386161102,39.3679726942069,7.86909595157452));
#60323=CARTESIAN_POINT('Ctrl Pts',(-19.2496120538636,39.3531045973913,7.71925523329057));
#60324=CARTESIAN_POINT('Ctrl Pts',(-19.1557551286073,39.2962241163357,7.14719552633411));
#60325=CARTESIAN_POINT('Ctrl Pts',(-18.3076284955857,39.19733125104,6.40503162152318));
#60326=CARTESIAN_POINT('Ctrl Pts',(-16.9267603470372,39.0712940983201,6.80034628368819));
#60327=CARTESIAN_POINT('Ctrl Pts',(-16.5101406589765,38.9452569456,8.17493663311751));
#60328=CARTESIAN_POINT('Ctrl Pts',(-17.4391877588077,38.8192197928801,9.27035529110332));
#60329=CARTESIAN_POINT('Ctrl Pts',(-18.4285950040459,38.7316582336349,9.14070744036985));
#60330=CARTESIAN_POINT('Ctrl Pts',(-18.7848458224106,38.6861090586297,8.8555733520524));
#60331=CARTESIAN_POINT('Ctrl Pts',(-18.8114966369182,38.6825722678645,8.83223897649705));
#60332=CARTESIAN_POINT('Origin',(-17.98,42.93984859951,7.87));
#60333=CARTESIAN_POINT('',(-18.8099615219029,37.7194233520466,8.8304622415411));
#60334=CARTESIAN_POINT('',(-18.8103597914526,37.8897334522804,8.83093840423764));
#60335=CARTESIAN_POINT('',(-18.810359785549,42.93984859951,8.83093840933902));
#60336=CARTESIAN_POINT('',(-19.2494450023513,38.40465140049,7.87113066820918));
#60337=CARTESIAN_POINT('Ctrl Pts',(-19.2494450023513,38.40465140049,7.87113066820918));
#60338=CARTESIAN_POINT('Ctrl Pts',(-19.2468218434614,38.3743553311533,7.5662963047995));
#60339=CARTESIAN_POINT('Ctrl Pts',(-18.9838065853326,38.3020468775766,6.83467797247145));
#60340=CARTESIAN_POINT('Ctrl Pts',(-17.7610940240468,38.1877260397599,6.38488952760496));
#60341=CARTESIAN_POINT('Ctrl Pts',(-16.6134802208024,38.0616888870399,7.2486332527821));
#60342=CARTESIAN_POINT('Ctrl Pts',(-16.7169250908296,37.9356517343199,8.68124269815259));
#60343=CARTESIAN_POINT('Ctrl Pts',(-17.857291976994,37.8215632226555,9.30574832435665));
#60344=CARTESIAN_POINT('Ctrl Pts',(-18.5791970423144,37.749487095231,9.02612225094904));
#60345=CARTESIAN_POINT('Ctrl Pts',(-18.8099615219027,37.7194233520466,8.8304622415412));
#60346=CARTESIAN_POINT('Ctrl Pts',(-18.810359785549,38.5130319987649,8.83093840933902));
#60347=CARTESIAN_POINT('Ctrl Pts',(-18.8479687726811,38.5081018195057,8.79843997844458));
#60348=CARTESIAN_POINT('Ctrl Pts',(-18.8836801829122,38.5031716402464,8.76371901167769));
#60349=CARTESIAN_POINT('Ctrl Pts',(-18.9172289811395,38.4982414609872,8.72703082611549));
#60350=CARTESIAN_POINT('Ctrl Pts',(-18.9508060520644,38.4933071269006,8.69031172218875));
#60351=CARTESIAN_POINT('Ctrl Pts',(-18.9822164951175,38.4883727928139,8.6516224889439));
#60352=CARTESIAN_POINT('Ctrl Pts',(-19.0112335911466,38.4834384587273,8.61125385698215));
#60353=CARTESIAN_POINT('Ctrl Pts',(-19.0402614685323,38.4785022912796,8.57087022597931));
#60354=CARTESIAN_POINT('Ctrl Pts',(-19.066893928649,38.4735661238318,8.52880641405647));
#60355=CARTESIAN_POINT('Ctrl Pts',(-19.0909479632238,38.4686299563841,8.48538168888006));
#60356=CARTESIAN_POINT('Ctrl Pts',(-19.1150504368909,38.4636838486716,8.44186951665765));
#60357=CARTESIAN_POINT('Ctrl Pts',(-19.1365638683119,38.4587377409592,8.39699144942104));
#60358=CARTESIAN_POINT('Ctrl Pts',(-19.1553521553955,38.4537916332468,8.3510897118076));
#60359=CARTESIAN_POINT('Ctrl Pts',(-19.1730679265148,38.4491278705645,8.30780824213878));
#60360=CARTESIAN_POINT('Ctrl Pts',(-19.1883611183866,38.4444641078822,8.26361718459007));
#60361=CARTESIAN_POINT('Ctrl Pts',(-19.2011587165291,38.4398003451999,8.21881426152752));
#60362=CARTESIAN_POINT('Ctrl Pts',(-19.2180120774238,38.4336585618171,8.1598125783129));
#60363=CARTESIAN_POINT('Ctrl Pts',(-19.2305987195022,38.4275167784342,8.09954154746724));
#60364=CARTESIAN_POINT('Ctrl Pts',(-19.2387654218309,38.4213749950514,8.03855151379594));
#60365=CARTESIAN_POINT('Ctrl Pts',(-19.2461778518552,38.4158004635309,7.98319448735252));
#60366=CARTESIAN_POINT('Ctrl Pts',(-19.2499495165899,38.4102259320105,7.92724526151886));
#60367=CARTESIAN_POINT('Ctrl Pts',(-19.2499994962489,38.40465140049,7.87113116208534));
#60368=CARTESIAN_POINT('',(-19.2518542553689,38.5741828836634,7.86958341168147));
#60369=CARTESIAN_POINT('Ctrl Pts',(-18.8114966369182,38.6825722678645,8.83223897649705));
#60370=CARTESIAN_POINT('Ctrl Pts',(-19.0836414450039,38.6464563268767,8.59395998673138));
#60371=CARTESIAN_POINT('Ctrl Pts',(-19.2503375314429,38.610340385889,8.23113979624163));
#60372=CARTESIAN_POINT('Ctrl Pts',(-19.251927057606,38.5742244449012,7.86957941617817));
#60373=CARTESIAN_POINT('Ctrl Pts',(-19.2499999609793,38.5731243067121,7.86968517832548));
#60374=CARTESIAN_POINT('Ctrl Pts',(-19.2499976467982,38.5721649088099,7.86034970331008));
#60375=CARTESIAN_POINT('Ctrl Pts',(-19.2498923981337,38.5712095171252,7.85101405572014));
#60376=CARTESIAN_POINT('Ctrl Pts',(-19.2494850282136,38.5693492592664,7.83275027757938));
#60377=CARTESIAN_POINT('Ctrl Pts',(-19.249191645318,38.5684440456419,7.82382248568587));
#60378=CARTESIAN_POINT('Ctrl Pts',(-19.248400106877,38.5666053569461,7.80559613257907));
#60379=CARTESIAN_POINT('Ctrl Pts',(-19.2478938593267,38.5656725322555,7.79629874300408));
#60380=CARTESIAN_POINT('Ctrl Pts',(-19.2464351530712,38.5634499807966,7.77402471215421));
#60381=CARTESIAN_POINT('Ctrl Pts',(-19.2453854873138,38.5621655154125,7.76105564341872));
#60382=CARTESIAN_POINT('Ctrl Pts',(-19.2412723286484,38.5579653159507,7.71839964852164));
#60383=CARTESIAN_POINT('Ctrl Pts',(-19.2373615874497,38.555089990553,7.6888016453913));
#60384=CARTESIAN_POINT('Ctrl Pts',(-19.2262667308048,38.5487105183809,7.62283282772677));
#60385=CARTESIAN_POINT('Ctrl Pts',(-19.2185265717978,38.5452249650623,7.58658384614804));
#60386=CARTESIAN_POINT('Ctrl Pts',(-19.1916012843344,38.5351784646923,7.48292197233717));
#60387=CARTESIAN_POINT('Ctrl Pts',(-19.1684126116585,38.5286556766224,7.41669925232812));
#60388=CARTESIAN_POINT('Ctrl Pts',(-19.1258751099155,38.5187147638503,7.32131685817229));
#60389=CARTESIAN_POINT('Ctrl Pts',(-19.1105976205512,38.5154119558307,7.2904902828806));
#60390=CARTESIAN_POINT('Ctrl Pts',(-19.0846677173216,38.5101575485012,7.24310731694291));
#60391=CARTESIAN_POINT('Ctrl Pts',(-19.074848631642,38.5082353703526,7.22611214426612));
#60392=CARTESIAN_POINT('Ctrl Pts',(-19.0551595489161,38.5045002516073,7.19378693092562));
#60393=CARTESIAN_POINT('Ctrl Pts',(-19.0453454060493,38.5026897429341,7.17842842180635));
#60394=CARTESIAN_POINT('Ctrl Pts',(-19.0208741330301,38.498290447733,7.14188994021249));
#60395=CARTESIAN_POINT('Ctrl Pts',(-19.0058973076877,38.4956901403741,7.12093545907858));
#60396=CARTESIAN_POINT('Ctrl Pts',(-18.9440180261012,38.4852836404473,7.03969765236556));
#60397=CARTESIAN_POINT('Ctrl Pts',(-18.8923643010938,38.477301370748,6.98325339636389));
#60398=CARTESIAN_POINT('Ctrl Pts',(-18.799581647996,38.4640653519918,6.89860316337923));
#60399=CARTESIAN_POINT('Ctrl Pts',(-18.7612943287668,38.4588627231777,6.86755025023491));
#60400=CARTESIAN_POINT('Ctrl Pts',(-18.6977355144261,38.4506939261036,6.8218598064911));
#60401=CARTESIAN_POINT('Ctrl Pts',(-18.6735959915075,38.4476897889213,6.80573164408738));
#60402=CARTESIAN_POINT('Ctrl Pts',(-18.6381925271546,38.4434412698912,6.78379471308814));
#60403=CARTESIAN_POINT('Ctrl Pts',(-18.627363489712,38.4421620802644,6.77730613275331));
#60404=CARTESIAN_POINT('Ctrl Pts',(-18.6074920237669,38.4398536564728,6.76579863880266));
#60405=CARTESIAN_POINT('Ctrl Pts',(-18.5984827821527,38.4388215622287,6.76072728656436));
#60406=CARTESIAN_POINT('Ctrl Pts',(-18.5759972610137,38.4362796645418,6.74842921218987));
#60407=CARTESIAN_POINT('Ctrl Pts',(-18.5624505393226,38.4347778069882,6.74133476378052));
#60408=CARTESIAN_POINT('Ctrl Pts',(-18.4738786457491,38.4251247828164,6.69696918396517));
#60409=CARTESIAN_POINT('Ctrl Pts',(-18.395436327126,38.4173316741842,6.66694742866786));
#60410=CARTESIAN_POINT('Ctrl Pts',(-18.2687553604257,38.4050271455999,6.63234967898701));
#60411=CARTESIAN_POINT('Ctrl Pts',(-18.2222529478992,38.4005678844358,6.62241396824339));
#60412=CARTESIAN_POINT('Ctrl Pts',(-18.1411270533502,38.3927543340857,6.60978788549234));
#60413=CARTESIAN_POINT('Ctrl Pts',(-18.1067486828358,38.3894332290498,6.60586757038739));
#60414=CARTESIAN_POINT('Ctrl Pts',(-18.0526497345825,38.3841571185286,6.6019272587129));
#60415=CARTESIAN_POINT('Ctrl Pts',(-18.0330139422562,38.3822319727734,6.60095473768511));
#60416=CARTESIAN_POINT('Ctrl Pts',(-17.9951584018545,38.3784952508256,6.59995987294544));
#60417=CARTESIAN_POINT('Ctrl Pts',(-17.9769450927404,38.3766861705908,6.59987312414843));
#60418=CARTESIAN_POINT('Ctrl Pts',(-17.9330804791314,38.3722978015241,6.60060761761898));
#60419=CARTESIAN_POINT('Ctrl Pts',(-17.9074450061548,38.3697071444885,6.60181468635598));
#60420=CARTESIAN_POINT('Ctrl Pts',(-17.8029447999354,38.3590277439848,6.60991372483158));
#60421=CARTESIAN_POINT('Ctrl Pts',(-17.7247847130406,38.3507471318824,6.62339417503107));
#60422=CARTESIAN_POINT('Ctrl Pts',(-17.6025485286636,38.3373989980658,6.65645688488191));
#60423=CARTESIAN_POINT('Ctrl Pts',(-17.5574233956132,38.3323838659728,6.67142335791343));
#60424=CARTESIAN_POINT('Ctrl Pts',(-17.4867987210199,38.324462625584,6.69933314732718));
#60425=CARTESIAN_POINT('Ctrl Pts',(-17.4607117141526,38.3215206842797,6.71066897000109));
#60426=CARTESIAN_POINT('Ctrl Pts',(-17.4236991583217,38.3173417127826,6.72825283703624));
#60427=CARTESIAN_POINT('Ctrl Pts',(-17.41245333362,38.3160713382579,6.73380105682558));
#60428=CARTESIAN_POINT('Ctrl Pts',(-17.3920728509226,38.3137701171472,6.74423408161451));
#60429=CARTESIAN_POINT('Ctrl Pts',(-17.3829134300982,38.3127365617054,6.74906517504684));
#60430=CARTESIAN_POINT('Ctrl Pts',(-17.3602477065413,38.3101788602424,6.76137679775517));
#60431=CARTESIAN_POINT('Ctrl Pts',(-17.3468167662757,38.3086629145994,6.76899255979818));
#60432=CARTESIAN_POINT('Ctrl Pts',(-17.2625958038725,38.2991314819451,6.81879970857973));
#60433=CARTESIAN_POINT('Ctrl Pts',(-17.1959019073837,38.2914603565271,6.86755987551028));
#60434=CARTESIAN_POINT('Ctrl Pts',(-17.0984938198642,38.2792284803047,6.95448801984256));
#60435=CARTESIAN_POINT('Ctrl Pts',(-17.0644453845139,38.2747145515071,6.98853843346888));
#60436=CARTESIAN_POINT('Ctrl Pts',(-17.0092051794265,38.2668204807477,7.05044378092391));
#60437=CARTESIAN_POINT('Ctrl Pts',(-16.9870807916653,38.2634745808771,7.07739294505653));
#60438=CARTESIAN_POINT('Ctrl Pts',(-16.9542302326868,38.2581690661467,7.12094422761147));
#60439=CARTESIAN_POINT('Ctrl Pts',(-16.9427343459682,38.25623990979,7.1369460983174));
#60440=CARTESIAN_POINT('Ctrl Pts',(-16.9213462026713,38.2525009565014,7.1682285069406));
#60441=CARTESIAN_POINT('Ctrl Pts',(-16.9114010824907,38.250693741297,7.18346714822124));
#60442=CARTESIAN_POINT('Ctrl Pts',(-16.8882924262967,38.246319754514,7.22059504863165));
#60443=CARTESIAN_POINT('Ctrl Pts',(-16.8754558736915,38.2437418152971,7.2426769183748));
#60444=CARTESIAN_POINT('Ctrl Pts',(-16.824569092692,38.2328577040173,7.3366234092631));
#60445=CARTESIAN_POINT('Ctrl Pts',(-16.7928069620044,38.224346786645,7.41165684700205));
#60446=CARTESIAN_POINT('Ctrl Pts',(-16.7545701246106,38.2109028708543,7.53330991949744));
#60447=CARTESIAN_POINT('Ctrl Pts',(-16.7431229774018,38.2060224670745,7.57815368389028));
#60448=CARTESIAN_POINT('Ctrl Pts',(-16.7287133597135,38.1982803814804,7.65098946282639));
#60449=CARTESIAN_POINT('Ctrl Pts',(-16.7241887573008,38.195384404995,7.67863030656963));
#60450=CARTESIAN_POINT('Ctrl Pts',(-16.7189743124548,38.1912569763955,7.71877222552474));
#60451=CARTESIAN_POINT('Ctrl Pts',(-16.7175495595056,38.1899932446534,7.73116716701736));
#60452=CARTESIAN_POINT('Ctrl Pts',(-16.7152754110474,38.1876973347979,7.75389987776677));
#60453=CARTESIAN_POINT('Ctrl Pts',(-16.7143696595033,38.1866625624029,7.7642295727156));
#60454=CARTESIAN_POINT('Ctrl Pts',(-16.7124217274978,38.184092387392,7.79007985859153));
#60455=CARTESIAN_POINT('Ctrl Pts',(-16.7115379364456,38.1825653852408,7.80561070027402));
#60456=CARTESIAN_POINT('Ctrl Pts',(-16.7078119969442,38.1731307884693,7.9024160823585));
#60457=CARTESIAN_POINT('Ctrl Pts',(-16.7124959753099,38.1655568916047,7.98380542716558));
#60458=CARTESIAN_POINT('Ctrl Pts',(-16.7323676674995,38.1533821422053,8.1122306411467));
#60459=CARTESIAN_POINT('Ctrl Pts',(-16.7425499134142,38.1488241262221,8.15979098488128));
#60460=CARTESIAN_POINT('Ctrl Pts',(-16.7647275357339,38.1408652981565,8.24046279470303));
#60461=CARTESIAN_POINT('Ctrl Pts',(-16.7754191607689,38.1374995930019,8.27387418437521));
#60462=CARTESIAN_POINT('Ctrl Pts',(-16.7942662964075,38.1321705970052,8.32532967119125));
#60463=CARTESIAN_POINT('Ctrl Pts',(-16.8014849235645,38.1302382466433,8.34369994040799));
#60464=CARTESIAN_POINT('Ctrl Pts',(-16.8161707491735,38.1264974651681,8.3786571520249));
#60465=CARTESIAN_POINT('Ctrl Pts',(-16.8235720838452,38.1246916834838,8.39526660880723));
#60466=CARTESIAN_POINT('Ctrl Pts',(-16.8421798361182,38.1203288476713,8.43472352953543));
#60467=CARTESIAN_POINT('Ctrl Pts',(-16.8537208225479,38.1177607811575,8.45740306906119));
#60468=CARTESIAN_POINT('Ctrl Pts',(-16.9125639166615,38.1052768086952,8.5649200037193));
#60469=CARTESIAN_POINT('Ctrl Pts',(-16.9688043742522,38.0950518824559,8.64447311777763));
#60470=CARTESIAN_POINT('Ctrl Pts',(-17.0577420795365,38.0809973294834,8.74387521550877));
#60471=CARTESIAN_POINT('Ctrl Pts',(-17.0830958193713,38.0771823958861,8.76987823280343));
#60472=CARTESIAN_POINT('Ctrl Pts',(-17.1271289231425,38.0708983650362,8.8113262122702));
#60473=CARTESIAN_POINT('Ctrl Pts',(-17.1451985787768,38.0684069477507,8.82738756619677));
#60474=CARTESIAN_POINT('Ctrl Pts',(-17.1728118306571,38.0647386307379,8.85055503791356));
#60475=CARTESIAN_POINT('Ctrl Pts',(-17.182013269141,38.0635381997632,8.85805776186167));
#60476=CARTESIAN_POINT('Ctrl Pts',(-17.1995026857574,38.061299246945,8.87191464252989));
#60477=CARTESIAN_POINT('Ctrl Pts',(-17.2077655167593,38.060259073004,8.87829704352528));
#60478=CARTESIAN_POINT('Ctrl Pts',(-17.2295119773185,38.05756444592,8.89467033013827));
#60479=CARTESIAN_POINT('Ctrl Pts',(-17.2431168415203,38.0559206693928,8.90449739947941));
#60480=CARTESIAN_POINT('Ctrl Pts',(-17.3116957394469,38.0478172357043,8.95199352425984));
#60481=CARTESIAN_POINT('Ctrl Pts',(-17.3693886087074,38.0415677440801,8.98557039862542));
#60482=CARTESIAN_POINT('Ctrl Pts',(-17.4798590050485,38.0300815396568,9.03871161820281));
#60483=CARTESIAN_POINT('Ctrl Pts',(-17.5318015383826,38.0248568531135,9.05959884036158));
#60484=CARTESIAN_POINT('Ctrl Pts',(-17.6211317674732,38.015937632364,9.08883674993836));
#60485=CARTESIAN_POINT('Ctrl Pts',(-17.6578244661591,38.012292553772,9.09904505763649));
#60486=CARTESIAN_POINT('Ctrl Pts',(-17.7146105692434,38.0066330747568,9.11212595369512));
#60487=CARTESIAN_POINT('Ctrl Pts',(-17.7344086287793,38.0046567699047,9.1161914779871));
#60488=CARTESIAN_POINT('Ctrl Pts',(-17.7720504322914,38.0008869459159,9.12298944707232));
#60489=CARTESIAN_POINT('Ctrl Pts',(-17.7898720548233,37.9990969635814,9.12581720645946));
#60490=CARTESIAN_POINT('Ctrl Pts',(-17.831845995079,37.9948648690826,9.13156333570185));
#60491=CARTESIAN_POINT('Ctrl Pts',(-17.856032817531,37.9924135537111,9.13416912918405));
#60492=CARTESIAN_POINT('Ctrl Pts',(-17.973286790395,37.9804554308039,9.14340462387749));
#60493=CARTESIAN_POINT('Ctrl Pts',(-18.0667994732495,37.9706614131296,9.14045752181102));
#60494=CARTESIAN_POINT('Ctrl Pts',(-18.1990356764231,37.9565788141841,9.12161847205612));
#60495=CARTESIAN_POINT('Ctrl Pts',(-18.2386584939408,37.9523334922567,9.11403441921126));
#60496=CARTESIAN_POINT('Ctrl Pts',(-18.3029399376025,37.9454511942824,9.09852579939953));
#60497=CARTESIAN_POINT('Ctrl Pts',(-18.3278367798188,37.9427871377813,9.09171016040832));
#60498=CARTESIAN_POINT('Ctrl Pts',(-18.36411628046,37.938921689114,9.08057921542769));
#60499=CARTESIAN_POINT('Ctrl Pts',(-18.3756704962152,37.9376931698901,9.07685220919659));
#60500=CARTESIAN_POINT('Ctrl Pts',(-18.3969677371777,37.935435492855,9.06964365237925));
#60501=CARTESIAN_POINT('Ctrl Pts',(-18.4067238758456,37.934404186528,9.06620806574128));
#60502=CARTESIAN_POINT('Ctrl Pts',(-18.4315836755829,37.9317816272642,9.05711090055117));
#60503=CARTESIAN_POINT('Ctrl Pts',(-18.4466236339688,37.930199904274,9.05128006057468));
#60504=CARTESIAN_POINT('Ctrl Pts',(-18.5317870734777,37.9212477217241,9.0163824299917));
#60505=CARTESIAN_POINT('Ctrl Pts',(-18.5993158529918,37.914160632271,8.98135669529544));
#60506=CARTESIAN_POINT('Ctrl Pts',(-18.7063745890262,37.9022635166177,8.91301909582715));
#60507=CARTESIAN_POINT('Ctrl Pts',(-18.7477281708972,37.8974800210177,8.88296679479367));
#60508=CARTESIAN_POINT('Ctrl Pts',(-18.7949705016936,37.8916644219046,8.84407673226505));
#60509=CARTESIAN_POINT('Ctrl Pts',(-18.8027049932364,37.8907003227464,8.83755301826742));
#60510=CARTESIAN_POINT('Ctrl Pts',(-18.8103597914526,37.8897334522804,8.83093840423764));
#60511=CARTESIAN_POINT('Origin',(-17.98,42.93984859951,7.87));
#60512=CARTESIAN_POINT('',(-18.8103597855476,36.9267571849074,8.8309384093402));
#60513=CARTESIAN_POINT('',(-18.8103598139481,37.0958383925403,8.83093838479897));
#60514=CARTESIAN_POINT('',(-18.810359785549,42.93984859951,8.83093840933902));
#60515=CARTESIAN_POINT('',(-19.2481622217284,37.6108862619992,7.86948592254581));
#60516=CARTESIAN_POINT('Ctrl Pts',(-18.8103597855476,36.9267571849074,8.8309384093402));
#60517=CARTESIAN_POINT('Ctrl Pts',(-18.8032147727197,36.92770968048,8.83711251088705));
#60518=CARTESIAN_POINT('Ctrl Pts',(-18.796000732487,36.9286565669442,8.84320707286185));
#60519=CARTESIAN_POINT('Ctrl Pts',(-18.7789281998143,36.9308627477655,8.85730692212138));
#60520=CARTESIAN_POINT('Ctrl Pts',(-18.7690164583287,36.9321174496358,8.86524585090824));
#60521=CARTESIAN_POINT('Ctrl Pts',(-18.7356538134999,36.9362616373254,8.89115625551136));
#60522=CARTESIAN_POINT('Ctrl Pts',(-18.7116928525083,36.9391108481981,8.90845982068869));
#60523=CARTESIAN_POINT('Ctrl Pts',(-18.6449018654357,36.9467852874517,8.95323224648113));
#60524=CARTESIAN_POINT('Ctrl Pts',(-18.6009900105569,36.9515475452395,8.97899003559175));
#60525=CARTESIAN_POINT('Ctrl Pts',(-18.4896955937105,36.9632433025765,9.03558348480202));
#60526=CARTESIAN_POINT('Ctrl Pts',(-18.4209470858209,36.9701627390575,9.06328873037541));
#60527=CARTESIAN_POINT('Ctrl Pts',(-18.3255305213228,36.9797503580514,9.0923636527249));
#60528=CARTESIAN_POINT('Ctrl Pts',(-18.3006560116582,36.982247274934,9.09912316088744));
#60529=CARTESIAN_POINT('Ctrl Pts',(-18.2578643879094,36.9865521630873,9.10936425879658));
#60530=CARTESIAN_POINT('Ctrl Pts',(-18.2400455744002,36.9883474600287,9.11322507897373));
#60531=CARTESIAN_POINT('Ctrl Pts',(-18.2028847358233,36.992101612378,9.12044295582655));
#60532=CARTESIAN_POINT('Ctrl Pts',(-18.1835358043025,36.9940619456363,9.12373771440852));
#60533=CARTESIAN_POINT('Ctrl Pts',(-18.1301068798706,36.9994958824706,9.13156634041531));
#60534=CARTESIAN_POINT('Ctrl Pts',(-18.095910162572,37.0029973583274,9.13516638191484));
#60535=CARTESIAN_POINT('Ctrl Pts',(-18.0146737588531,37.0113819650799,9.14039765636493));
#60536=CARTESIAN_POINT('Ctrl Pts',(-17.9676080787579,37.0162932639401,9.14080993719881));
#60537=CARTESIAN_POINT('Ctrl Pts',(-17.835829115862,37.0301650074422,9.13464313778041));
#60538=CARTESIAN_POINT('Ctrl Pts',(-17.7516301602392,37.0391811380149,9.12218100248414));
#60539=CARTESIAN_POINT('Ctrl Pts',(-17.6545926545394,37.0494514364498,9.09769706672792));
#60540=CARTESIAN_POINT('Ctrl Pts',(-17.6399532677227,37.0509969477241,9.09372314033049));
#60541=CARTESIAN_POINT('Ctrl Pts',(-17.6154715581996,37.0535713957757,9.08660414816243));
#60542=CARTESIAN_POINT('Ctrl Pts',(-17.6055907512118,37.0546074955674,9.08359976546825));
#60543=CARTESIAN_POINT('Ctrl Pts',(-17.58364067524,37.0569020631242,9.07663192496756));
#60544=CARTESIAN_POINT('Ctrl Pts',(-17.5715923482799,37.058157101892,9.07260739855669));
#60545=CARTESIAN_POINT('Ctrl Pts',(-17.5317041161362,37.0623040875157,9.05861477728356));
#60546=CARTESIAN_POINT('Ctrl Pts',(-17.5041494145224,37.065155683937,9.04785438621417));
#60547=CARTESIAN_POINT('Ctrl Pts',(-17.4302198010537,37.0728399499147,9.01596527888472));
#60548=CARTESIAN_POINT('Ctrl Pts',(-17.3846994047278,37.0776094507408,8.99299278388375));
#60549=CARTESIAN_POINT('Ctrl Pts',(-17.2768454439438,37.0893020305867,8.93015631443276));
#60550=CARTESIAN_POINT('Ctrl Pts',(-17.2163870695905,37.0962112421349,8.88747280345882));
#60551=CARTESIAN_POINT('Ctrl Pts',(-17.1403056282913,37.1057879323274,8.82314089395605));
#60552=CARTESIAN_POINT('Ctrl Pts',(-17.1211386618713,37.1082847782095,8.8059066114038));
#60553=CARTESIAN_POINT('Ctrl Pts',(-17.0893309797913,37.1125895848295,8.77550597823357));
#60554=CARTESIAN_POINT('Ctrl Pts',(-17.0764249581612,37.1143848725165,8.76262782706307));
#60555=CARTESIAN_POINT('Ctrl Pts',(-17.0502099748453,37.1181390423304,8.7353182712188));
#60556=CARTESIAN_POINT('Ctrl Pts',(-17.0369496243363,37.1200994028227,8.72084727140804));
#60557=CARTESIAN_POINT('Ctrl Pts',(-17.0013991121509,37.12553352916,8.68019881367165));
#60558=CARTESIAN_POINT('Ctrl Pts',(-16.9798303666594,37.129035170718,8.65341684492043));
#60559=CARTESIAN_POINT('Ctrl Pts',(-16.9313821811308,37.1374203159222,8.58799267093613));
#60560=CARTESIAN_POINT('Ctrl Pts',(-16.9055130546705,37.1423319931642,8.54866751142825));
#60561=CARTESIAN_POINT('Ctrl Pts',(-16.839241869639,37.1562032654584,8.43460340653079));
#60562=CARTESIAN_POINT('Ctrl Pts',(-16.8040600152699,37.1652185060364,8.35710759355697));
#60563=CARTESIAN_POINT('Ctrl Pts',(-16.7720155421243,37.1754880770742,8.26230550034684));
#60564=CARTESIAN_POINT('Ctrl Pts',(-16.7674160264586,37.1770336847903,8.24784949301934));
#60565=CARTESIAN_POINT('Ctrl Pts',(-16.7601220713794,37.1796082388778,8.22341827832901));
#60566=CARTESIAN_POINT('Ctrl Pts',(-16.7572885300784,37.1806443497761,8.21348702979182));
#60567=CARTESIAN_POINT('Ctrl Pts',(-16.7512407667314,37.1829388741249,8.191266321197));
#60568=CARTESIAN_POINT('Ctrl Pts',(-16.7480891929481,37.184193859606,8.17896134760367));
#60569=CARTESIAN_POINT('Ctrl Pts',(-16.7382177390019,37.1883404025483,8.13786352204775));
#60570=CARTESIAN_POINT('Ctrl Pts',(-16.7323179536728,37.1911916215231,8.10888073979877));
#60571=CARTESIAN_POINT('Ctrl Pts',(-16.7190254406704,37.1988743319381,8.02948844936912));
#60572=CARTESIAN_POINT('Ctrl Pts',(-16.7136440230555,37.2036426860336,7.97879727898873));
#60573=CARTESIAN_POINT('Ctrl Pts',(-16.7079514469827,37.2153357665958,7.85409839389578));
#60574=CARTESIAN_POINT('Ctrl Pts',(-16.7110307687797,37.2222465948687,7.78013708005916));
#60575=CARTESIAN_POINT('Ctrl Pts',(-16.7238310514371,37.2318250137831,7.68131035823987));
#60576=CARTESIAN_POINT('Ctrl Pts',(-16.7279184201746,37.2343218717183,7.65586054195609));
#60577=CARTESIAN_POINT('Ctrl Pts',(-16.736214035353,37.2386266921784,7.6126503254698));
#60578=CARTESIAN_POINT('Ctrl Pts',(-16.7400362628188,37.2404219814352,7.59482328402615));
#60579=CARTESIAN_POINT('Ctrl Pts',(-16.7487672856928,37.2441761482803,7.55798845713815));
#60580=CARTESIAN_POINT('Ctrl Pts',(-16.7537357062197,37.2461365041465,7.53900004474447));
#60581=CARTESIAN_POINT('Ctrl Pts',(-16.7686120872288,37.2515705983024,7.48708862421732));
#60582=CARTESIAN_POINT('Ctrl Pts',(-16.7794191360676,37.2550722117221,7.45444396398152));
#60583=CARTESIAN_POINT('Ctrl Pts',(-16.8081185623732,37.2634572654977,7.37826160861739));
#60584=CARTESIAN_POINT('Ctrl Pts',(-16.8271325697097,37.2683688784931,7.33520245064047));
#60585=CARTESIAN_POINT('Ctrl Pts',(-16.8870362131116,37.2822402306931,7.2176684008618));
#60586=CARTESIAN_POINT('Ctrl Pts',(-16.9330731704459,37.2912556222798,7.14608487720421));
#60587=CARTESIAN_POINT('Ctrl Pts',(-16.9953525687587,37.3015253167339,7.067753474623));
#60588=CARTESIAN_POINT('Ctrl Pts',(-17.0050046249948,37.3030709080812,7.05605028027594));
#60589=CARTESIAN_POINT('Ctrl Pts',(-17.021576983394,37.3056454441737,7.03667415670937));
#60590=CARTESIAN_POINT('Ctrl Pts',(-17.0283849269966,37.3066815531887,7.02890819121319));
#60591=CARTESIAN_POINT('Ctrl Pts',(-17.0437758811704,37.3089760848798,7.01177759047472));
#60592=CARTESIAN_POINT('Ctrl Pts',(-17.0524058997014,37.3102310794118,7.00245718356506));
#60593=CARTESIAN_POINT('Ctrl Pts',(-17.081584890469,37.3143776975236,6.97187730149772));
#60594=CARTESIAN_POINT('Ctrl Pts',(-17.1027381710886,37.3172289805884,6.95120392874093));
#60595=CARTESIAN_POINT('Ctrl Pts',(-17.1622395118933,37.3249119551117,6.89698334720371));
#60596=CARTESIAN_POINT('Ctrl Pts',(-17.2019149886439,37.3296805038975,6.8649735121972));
#60597=CARTESIAN_POINT('Ctrl Pts',(-17.3036024417685,37.3413734993826,6.7925742360146));
#60598=CARTESIAN_POINT('Ctrl Pts',(-17.3674134391802,37.3482840531108,6.75505806825942));
#60599=CARTESIAN_POINT('Ctrl Pts',(-17.4573877313516,37.3578621784835,6.71222600487515));
#60600=CARTESIAN_POINT('Ctrl Pts',(-17.480987505808,37.3603590343976,6.70186023115464));
#60601=CARTESIAN_POINT('Ctrl Pts',(-17.5217918187434,37.364663852542,6.68539979598401));
#60602=CARTESIAN_POINT('Ctrl Pts',(-17.5388430335696,37.3664591415407,6.67894465896834));
#60603=CARTESIAN_POINT('Ctrl Pts',(-17.5745267446772,37.3702133088996,6.66630708269495));
#60604=CARTESIAN_POINT('Ctrl Pts',(-17.5931752950012,37.3721736655526,6.6601852470418));
#60605=CARTESIAN_POINT('Ctrl Pts',(-17.644858999498,37.3776077651561,6.64453587983283));
#60606=CARTESIAN_POINT('Ctrl Pts',(-17.6781478086027,37.381109383335,6.6359147162447));
#60607=CARTESIAN_POINT('Ctrl Pts',(-17.757720017215,37.389494452571,6.61871890921272));
#60608=CARTESIAN_POINT('Ctrl Pts',(-17.8042095413234,37.394406076429,6.61134617358325));
#60609=CARTESIAN_POINT('Ctrl Pts',(-17.9354463509943,37.4082774150947,6.59794603608985));
#60610=CARTESIAN_POINT('Ctrl Pts',(-18.0205553622639,37.4172927811241,6.5978112899045));
#60611=CARTESIAN_POINT('Ctrl Pts',(-18.1201415089112,37.4275624546922,6.6076647000054));
#60612=CARTESIAN_POINT('Ctrl Pts',(-18.1352085804882,37.4291080488103,6.60942853242417));
#60613=CARTESIAN_POINT('Ctrl Pts',(-18.1604751086731,37.4316825879504,6.6128463200297));
#60614=CARTESIAN_POINT('Ctrl Pts',(-18.1706918102567,37.4327186972858,6.61435541990018));
#60615=CARTESIAN_POINT('Ctrl Pts',(-18.1934309520643,37.4350132277385,6.61799818962467));
#60616=CARTESIAN_POINT('Ctrl Pts',(-18.2059417207708,37.4362682207414,6.6201953385972));
#60617=CARTESIAN_POINT('Ctrl Pts',(-18.2474576090307,37.440414826157,6.62813023583685));
#60618=CARTESIAN_POINT('Ctrl Pts',(-18.2762979595537,37.4432660983974,6.63469354030739));
#60619=CARTESIAN_POINT('Ctrl Pts',(-18.3541190855989,37.4509490283154,6.65528666116701));
#60620=CARTESIAN_POINT('Ctrl Pts',(-18.4025279273838,37.45571754422,6.67126540056843));
#60621=CARTESIAN_POINT('Ctrl Pts',(-18.5184990658107,37.4674105540678,6.71744684913855));
#60622=CARTESIAN_POINT('Ctrl Pts',(-18.5846226474918,37.4743211541578,6.750719277603));
#60623=CARTESIAN_POINT('Ctrl Pts',(-18.6693996600084,37.4838993290987,6.80309217075874));
#60624=CARTESIAN_POINT('Ctrl Pts',(-18.6909060815612,37.4863961853522,6.81730035988232));
#60625=CARTESIAN_POINT('Ctrl Pts',(-18.7268624561893,37.4907010038829,6.84265932997988));
#60626=CARTESIAN_POINT('Ctrl Pts',(-18.7415321487791,37.4924962929224,6.85348581868069));
#60627=CARTESIAN_POINT('Ctrl Pts',(-18.7714998507502,37.4962504601872,6.87661528793545));
#60628=CARTESIAN_POINT('Ctrl Pts',(-18.7867556450977,37.4982108167026,6.88896461943294));
#60629=CARTESIAN_POINT('Ctrl Pts',(-18.82792984546,37.503644915365,6.92390445689966));
#60630=CARTESIAN_POINT('Ctrl Pts',(-18.8532242472879,37.5071465327236,6.94719956304562));
#60631=CARTESIAN_POINT('Ctrl Pts',(-18.9108202282476,37.5155315992946,7.00473330125536));
#60632=CARTESIAN_POINT('Ctrl Pts',(-18.9422237122834,37.5204432212802,7.03979685257261));
#60633=CARTESIAN_POINT('Ctrl Pts',(-19.0246454802072,37.5343145623159,7.1427984169679));
#60634=CARTESIAN_POINT('Ctrl Pts',(-19.07090877644,37.5433299327892,7.2142356368844));
#60635=CARTESIAN_POINT('Ctrl Pts',(-19.1166299938529,37.5535996099898,7.30325287026133));
#60636=CARTESIAN_POINT('Ctrl Pts',(-19.1233180506155,37.5551452036275,7.31686894561871));
#60637=CARTESIAN_POINT('Ctrl Pts',(-19.1341470404879,37.5577197422377,7.33995165424622));
#60638=CARTESIAN_POINT('Ctrl Pts',(-19.1384190347504,37.5587558515162,7.34935422987331));
#60639=CARTESIAN_POINT('Ctrl Pts',(-19.1476885271846,37.5610503821786,7.37043538152376));
#60640=CARTESIAN_POINT('Ctrl Pts',(-19.1526263600369,37.5623053754431,7.38213857227139));
#60641=CARTESIAN_POINT('Ctrl Pts',(-19.168471153579,37.5664519830324,7.4213237224336));
#60642=CARTESIAN_POINT('Ctrl Pts',(-19.1785951192066,37.5693032571264,7.44911489503905));
#60643=CARTESIAN_POINT('Ctrl Pts',(-19.2034906236037,37.5769861946825,7.52566834882584));
#60644=CARTESIAN_POINT('Ctrl Pts',(-19.2163145043556,37.5817547162179,7.57500687819286));
#60645=CARTESIAN_POINT('Ctrl Pts',(-19.2371219520155,37.5918576196773,7.68083363887858));
#60646=CARTESIAN_POINT('Ctrl Pts',(-19.2443350737353,37.59718194391,7.73735183038249));
#60647=CARTESIAN_POINT('Ctrl Pts',(-19.2492360708524,37.6049924265085,7.81927636743861));
#60648=CARTESIAN_POINT('Ctrl Pts',(-19.2499917500813,37.6074024411012,7.8444297094667));
#60649=CARTESIAN_POINT('Ctrl Pts',(-19.249999932819,37.6098335524356,7.8695869145078));
#60650=CARTESIAN_POINT('Ctrl Pts',(-18.8099615219027,37.7194233520466,8.8304622415412));
#60651=CARTESIAN_POINT('Ctrl Pts',(-18.9016773777114,37.7074747109911,8.75269843125987));
#60652=CARTESIAN_POINT('Ctrl Pts',(-19.1457002117025,37.6713007271388,8.4794805454805));
#60653=CARTESIAN_POINT('Ctrl Pts',(-19.2472428947117,37.6351267432866,8.11387022531887));
#60654=CARTESIAN_POINT('Ctrl Pts',(-19.2481357945224,37.61090140049,7.86948447023081));
#60655=CARTESIAN_POINT('Ctrl Pts',(-18.8103597914526,37.8897334522804,8.83093840423764));
#60656=CARTESIAN_POINT('Ctrl Pts',(-18.8300348678934,37.8872483116158,8.81393690622473));
#60657=CARTESIAN_POINT('Ctrl Pts',(-18.8491834500945,37.884744708031,8.79633489929289));
#60658=CARTESIAN_POINT('Ctrl Pts',(-18.8820134020668,37.8802822135894,8.76424162825049));
#60659=CARTESIAN_POINT('Ctrl Pts',(-18.8959180353935,37.8783340914939,8.74999449475032));
#60660=CARTESIAN_POINT('Ctrl Pts',(-18.9218326402294,37.8745836694053,8.72216184613498));
#60661=CARTESIAN_POINT('Ctrl Pts',(-18.9338978123935,37.8727843460154,8.70863425330909));
#60662=CARTESIAN_POINT('Ctrl Pts',(-18.9619094478656,37.868472964352,8.67584062268679));
#60663=CARTESIAN_POINT('Ctrl Pts',(-18.9775836357603,37.8659506076449,8.65635356894627));
#60664=CARTESIAN_POINT('Ctrl Pts',(-19.04543573706,37.8545064982477,8.56670035962305));
#60665=CARTESIAN_POINT('Ctrl Pts',(-19.0908482208755,37.8453401152098,8.49173493060826));
#60666=CARTESIAN_POINT('Ctrl Pts',(-19.1465824485972,37.8315882950702,8.37382196217949));
#60667=CARTESIAN_POINT('Ctrl Pts',(-19.1629813568602,37.8270527903362,8.33401156590888));
#60668=CARTESIAN_POINT('Ctrl Pts',(-19.1862766564356,37.8197744014533,8.26814176587284));
#60669=CARTESIAN_POINT('Ctrl Pts',(-19.1944215314265,37.8170011561596,8.24255994228225));
#60670=CARTESIAN_POINT('Ctrl Pts',(-19.2051086219464,37.8130119647009,8.20490321993921));
#60671=CARTESIAN_POINT('Ctrl Pts',(-19.2082950704449,37.8117665114033,8.19302099989463));
#60672=CARTESIAN_POINT('Ctrl Pts',(-19.2138594272067,37.8094846536562,8.17099726688584));
#60673=CARTESIAN_POINT('Ctrl Pts',(-19.216285896331,37.808445973111,8.16087048729322));
#60674=CARTESIAN_POINT('Ctrl Pts',(-19.2221012019579,37.8058387315869,8.13521172880683));
#60675=CARTESIAN_POINT('Ctrl Pts',(-19.2253235487809,37.8042791626728,8.11964375305414));
#60676=CARTESIAN_POINT('Ctrl Pts',(-19.2426459370111,37.795130771309,8.02724607696535));
#60677=CARTESIAN_POINT('Ctrl Pts',(-19.2499282836218,37.7878452278459,7.94929534338273));
#60678=CARTESIAN_POINT('Ctrl Pts',(-19.2500624775109,37.7740476776123,7.80200242607106));
#60679=CARTESIAN_POINT('Ctrl Pts',(-19.2444771305498,37.767565959847,7.73296711427041));
#60680=CARTESIAN_POINT('Ctrl Pts',(-19.2291580819846,37.7584540476398,7.63943217797024));
#60681=CARTESIAN_POINT('Ctrl Pts',(-19.2242489537417,37.7559695433459,7.61426232146536));
#60682=CARTESIAN_POINT('Ctrl Pts',(-19.2145565353906,37.7516791989012,7.57150081758896));
#60683=CARTESIAN_POINT('Ctrl Pts',(-19.2101499181603,37.7498858137683,7.55383122577677));
#60684=CARTESIAN_POINT('Ctrl Pts',(-19.200197431579,37.7461294947516,7.51728912017404));
#60685=CARTESIAN_POINT('Ctrl Pts',(-19.1945899766567,37.7441649971644,7.49843868119012));
#60686=CARTESIAN_POINT('Ctrl Pts',(-19.1779045879273,37.7387004445672,7.44676945610031));
#60687=CARTESIAN_POINT('Ctrl Pts',(-19.1659192761353,37.7351719517395,7.41426500407277));
#60688=CARTESIAN_POINT('Ctrl Pts',(-19.1343369829196,37.726698944372,7.33832961017935));
#60689=CARTESIAN_POINT('Ctrl Pts',(-19.1135956950872,37.7217253240388,7.29543318194078));
#60690=CARTESIAN_POINT('Ctrl Pts',(-19.0499550046961,37.7079298625437,7.18074041689903));
#60691=CARTESIAN_POINT('Ctrl Pts',(-19.0022965308763,37.6990587882167,7.1118477773202));
#60692=CARTESIAN_POINT('Ctrl Pts',(-18.938301227963,37.6889075712726,7.03645741087996));
#60693=CARTESIAN_POINT('Ctrl Pts',(-18.9281803210313,37.687346721933,7.02496233911568));
#60694=CARTESIAN_POINT('Ctrl Pts',(-18.9108806070277,37.6847555416129,7.00601607517522));
#60695=CARTESIAN_POINT('Ctrl Pts',(-18.9038147120301,37.6837178049028,6.99846494986995));
#60696=CARTESIAN_POINT('Ctrl Pts',(-18.8879295768371,37.6814305695523,6.98189929332437));
#60697=CARTESIAN_POINT('Ctrl Pts',(-18.8790670054897,37.6801843333883,6.97292834802095));
#60698=CARTESIAN_POINT('Ctrl Pts',(-18.8494406842844,37.6761085995669,6.94381998775933));
#60699=CARTESIAN_POINT('Ctrl Pts',(-18.8281206851935,37.6733175590677,6.92425783440027));
#60700=CARTESIAN_POINT('Ctrl Pts',(-18.7689642970215,37.6658789910054,6.87359028598551));
#60701=CARTESIAN_POINT('Ctrl Pts',(-18.7299661820066,37.6612897773079,6.84391591089947));
#60702=CARTESIAN_POINT('Ctrl Pts',(-18.6256367778902,37.6495062819862,6.77366387540398));
#60703=CARTESIAN_POINT('Ctrl Pts',(-18.5581725166867,37.6423318853709,6.73663595867115));
#60704=CARTESIAN_POINT('Ctrl Pts',(-18.4641850231329,37.6324755064397,6.69563733148107));
#60705=CARTESIAN_POINT('Ctrl Pts',(-18.4402817772613,37.6299811927968,6.68606449425396));
#60706=CARTESIAN_POINT('Ctrl Pts',(-18.3989897993358,37.6256795994836,6.67096719033118));
#60707=CARTESIAN_POINT('Ctrl Pts',(-18.3817419663761,37.6238849511069,6.66507865947308));
#60708=CARTESIAN_POINT('Ctrl Pts',(-18.3456658829058,37.6201311300037,6.65362268630146));
#60709=CARTESIAN_POINT('Ctrl Pts',(-18.3268234522634,37.6181704655535,6.64811674492403));
#60710=CARTESIAN_POINT('Ctrl Pts',(-18.2746179459316,37.612732619033,6.63416652777873));
#60711=CARTESIAN_POINT('Ctrl Pts',(-18.2410305442971,37.6092274850052,6.62663899389277));
#60712=CARTESIAN_POINT('Ctrl Pts',(-18.1608253925956,37.6008306843994,6.61205634645845));
#60713=CARTESIAN_POINT('Ctrl Pts',(-18.1140404250063,37.5959107175078,6.60621512898476));
#60714=CARTESIAN_POINT('Ctrl Pts',(-17.9825334047712,37.5820496667026,6.59718052106978));
#60715=CARTESIAN_POINT('Ctrl Pts',(-17.8976470506054,37.5730538159799,6.59984395902575));
#60716=CARTESIAN_POINT('Ctrl Pts',(-17.7985964209878,37.5628002568999,6.61293064661125));
#60717=CARTESIAN_POINT('Ctrl Pts',(-17.7835767736196,37.5612527067091,6.6151898110559));
#60718=CARTESIAN_POINT('Ctrl Pts',(-17.7584173899679,37.5586762016982,6.61943701142443));
#60719=CARTESIAN_POINT('Ctrl Pts',(-17.7482555591945,37.5576400494988,6.62128017800801));
#60720=CARTESIAN_POINT('Ctrl Pts',(-17.7256644858379,37.5553471162272,6.6256630989959));
#60721=CARTESIAN_POINT('Ctrl Pts',(-17.7132488896122,37.5540937360872,6.62826541875204));
#60722=CARTESIAN_POINT('Ctrl Pts',(-17.6721387845193,37.5499593837391,6.63752725712236));
#60723=CARTESIAN_POINT('Ctrl Pts',(-17.643634326914,37.5471184277162,6.64499952405626));
#60724=CARTESIAN_POINT('Ctrl Pts',(-17.5669539627857,37.5394775957703,6.66798000669751));
#60725=CARTESIAN_POINT('Ctrl Pts',(-17.5194025060431,37.5347400201923,6.68538616565481));
#60726=CARTESIAN_POINT('Ctrl Pts',(-17.4048165879097,37.5230329594593,6.73527695349495));
#60727=CARTESIAN_POINT('Ctrl Pts',(-17.3393695002255,37.5160782339928,6.77089911019834));
#60728=CARTESIAN_POINT('Ctrl Pts',(-17.2559512047949,37.5064532264038,6.826296244133));
#60729=CARTESIAN_POINT('Ctrl Pts',(-17.2349230539527,37.5039564137256,6.84120249119583));
#60730=CARTESIAN_POINT('Ctrl Pts',(-17.1998212331697,37.4996519518082,6.86772590658961));
#60731=CARTESIAN_POINT('Ctrl Pts',(-17.1855172287835,37.4978569788531,6.87902608181375));
#60732=CARTESIAN_POINT('Ctrl Pts',(-17.1563320419713,37.4941037771619,6.90312046056595));
#60733=CARTESIAN_POINT('Ctrl Pts',(-17.1414944667088,37.4921440748641,6.91595948276378));
#60734=CARTESIAN_POINT('Ctrl Pts',(-17.1015097625954,37.4867129194701,6.95221180615699));
#60735=CARTESIAN_POINT('Ctrl Pts',(-17.0770083707477,37.4832136355872,6.97630776129775));
#60736=CARTESIAN_POINT('Ctrl Pts',(-17.0213745734389,37.4748358492621,7.0356465583227));
#60737=CARTESIAN_POINT('Ctrl Pts',(-16.9911642464969,37.4699292454559,7.07168226249463));
#60738=CARTESIAN_POINT('Ctrl Pts',(-16.9121105187079,37.4560515609369,7.17736951288542));
#60739=CARTESIAN_POINT('Ctrl Pts',(-16.8681559722528,37.4470242886199,7.25037887929964));
#60740=CARTESIAN_POINT('Ctrl Pts',(-16.8253469751711,37.4367450435555,7.34093854392923));
#60741=CARTESIAN_POINT('Ctrl Pts',(-16.8191159331536,37.4352008949839,7.35475453287355));
#60742=CARTESIAN_POINT('Ctrl Pts',(-16.8090581676939,37.4326281315143,7.37816486859752));
#60743=CARTESIAN_POINT('Ctrl Pts',(-16.8050987290957,37.4315923725561,7.38769966535942));
#60744=CARTESIAN_POINT('Ctrl Pts',(-16.7965270808923,37.4292979219784,7.40907351367023));
#60745=CARTESIAN_POINT('Ctrl Pts',(-16.7919754670223,37.4280426674629,7.42093526803272));
#60746=CARTESIAN_POINT('Ctrl Pts',(-16.7774151962916,37.4238927630328,7.46065206558879));
#60747=CARTESIAN_POINT('Ctrl Pts',(-16.7682012606276,37.4210385484136,7.48879112757948));
#60748=CARTESIAN_POINT('Ctrl Pts',(-16.7458037897351,37.4133431719075,7.56625067365603));
#60749=CARTESIAN_POINT('Ctrl Pts',(-16.7345955526899,37.4085654082228,7.61608543269077));
#60750=CARTESIAN_POINT('Ctrl Pts',(-16.7145964222888,37.3968762057408,7.73926028246334));
#60751=CARTESIAN_POINT('Ctrl Pts',(-16.7091416258319,37.3899784178123,7.81293899509459));
#60752=CARTESIAN_POINT('Ctrl Pts',(-16.7104475938165,37.3804141991619,7.91243468420286));
#60753=CARTESIAN_POINT('Ctrl Pts',(-16.7115698864676,37.3779177016801,7.93818242760502));
#60754=CARTESIAN_POINT('Ctrl Pts',(-16.7148216951835,37.3736136016348,7.98205403335076));
#60755=CARTESIAN_POINT('Ctrl Pts',(-16.7165601537087,37.3718186696788,8.00019953121382));
#60756=CARTESIAN_POINT('Ctrl Pts',(-16.7209795700339,37.3680653902383,8.03778721898458));
#60757=CARTESIAN_POINT('Ctrl Pts',(-16.7237219040064,37.3661055669052,8.05721706242381));
#60758=CARTESIAN_POINT('Ctrl Pts',(-16.7325021958648,37.360673570058,8.11047864163257));
#60759=CARTESIAN_POINT('Ctrl Pts',(-16.7394643874593,37.3571735505313,8.14413787797057));
#60760=CARTESIAN_POINT('Ctrl Pts',(-16.7591624715368,37.34879337476,8.2230801174656));
#60761=CARTESIAN_POINT('Ctrl Pts',(-16.7730656431776,37.3438850921945,8.26801794079559));
#60762=CARTESIAN_POINT('Ctrl Pts',(-16.8190003224163,37.3300095043497,8.39172645694));
#60763=CARTESIAN_POINT('Ctrl Pts',(-16.8564955624613,37.3209861875035,8.46821322664545));
#60764=CARTESIAN_POINT('Ctrl Pts',(-16.9093537069664,37.3107101738324,8.55326149576562));
#60765=CARTESIAN_POINT('Ctrl Pts',(-16.9175854348212,37.3091655957653,8.56599218683689));
#60766=CARTESIAN_POINT('Ctrl Pts',(-16.9318037602163,37.3065923601604,8.58714100625244));
#60767=CARTESIAN_POINT('Ctrl Pts',(-16.9376682440562,37.3055565518295,8.59563842825465));
#60768=CARTESIAN_POINT('Ctrl Pts',(-16.9509776385803,37.3032622942126,8.61442883636469));
#60769=CARTESIAN_POINT('Ctrl Pts',(-16.9584744134487,37.302007277446,8.62468326939275));
#60770=CARTESIAN_POINT('Ctrl Pts',(-16.9839371151218,37.297859349712,8.65843744638727));
#60771=CARTESIAN_POINT('Ctrl Pts',(-17.0025716876115,37.2950068206424,8.68142419151736));
#60772=CARTESIAN_POINT('Ctrl Pts',(-17.0554574247065,37.2873183978818,8.74219219273994));
#60773=CARTESIAN_POINT('Ctrl Pts',(-17.091207815977,37.2825457618921,8.77859647422016));
#60774=CARTESIAN_POINT('Ctrl Pts',(-17.1838586369744,37.2708543423037,8.86222466339401));
#60775=CARTESIAN_POINT('Ctrl Pts',(-17.242866698744,37.2639493447231,8.90681397703108));
#60776=CARTESIAN_POINT('Ctrl Pts',(-17.3272409798854,37.2543774105935,8.95971083770372));
#60777=CARTESIAN_POINT('Ctrl Pts',(-17.3494838245695,37.251880851879,8.97272987741142));
#60778=CARTESIAN_POINT('Ctrl Pts',(-17.3881094986076,37.2475766815356,8.9937872961838));
#60779=CARTESIAN_POINT('Ctrl Pts',(-17.4042984388306,37.2457817416169,9.00216601208701));
#60780=CARTESIAN_POINT('Ctrl Pts',(-17.4382766132721,37.2420284772915,9.01883452134757));
#60781=CARTESIAN_POINT('Ctrl Pts',(-17.4560887486572,37.2400686774807,9.02706606332457));
#60782=CARTESIAN_POINT('Ctrl Pts',(-17.5055997441572,37.234636844165,9.04856906963251));
#60783=CARTESIAN_POINT('Ctrl Pts',(-17.5376547931556,37.231136967607,9.06097053128938));
#60784=CARTESIAN_POINT('Ctrl Pts',(-17.6146605148829,37.2227572562461,9.08722496518036));
#60785=CARTESIAN_POINT('Ctrl Pts',(-17.6599540555282,37.217849299974,9.09991021275116));
#60786=CARTESIAN_POINT('Ctrl Pts',(-17.7888078696275,37.2039733047731,9.12839799701166));
#60787=CARTESIAN_POINT('Ctrl Pts',(-17.8734122417257,37.1949492193082,9.13836963777536));
#60788=CARTESIAN_POINT('Ctrl Pts',(-17.9735398806138,37.1846725776728,9.14007401323111));
#60789=CARTESIAN_POINT('Ctrl Pts',(-17.9886992834016,37.1831280830351,9.14006067994603));
#60790=CARTESIAN_POINT('Ctrl Pts',(-18.0141778891335,37.1805549391477,9.13958199818897));
#60791=CARTESIAN_POINT('Ctrl Pts',(-18.0244975003084,37.1795191404128,9.13926222222058));
#60792=CARTESIAN_POINT('Ctrl Pts',(-18.0475029378813,37.1772248453393,9.1382683779033));
#60793=CARTESIAN_POINT('Ctrl Pts',(-18.0601844934833,37.1759697824103,9.13752981045374));
#60794=CARTESIAN_POINT('Ctrl Pts',(-18.1023564244237,37.1718214709779,9.13443821097716));
#60795=CARTESIAN_POINT('Ctrl Pts',(-18.1317783168588,37.1689686147343,9.1312449696965));
#60796=CARTESIAN_POINT('Ctrl Pts',(-18.2115280182011,37.1612788426634,9.11975761064508));
#60797=CARTESIAN_POINT('Ctrl Pts',(-18.261511607922,37.1565052117878,9.10945610176486));
#60798=CARTESIAN_POINT('Ctrl Pts',(-18.3820116156005,37.1448142237615,9.07695286895875));
#60799=CARTESIAN_POINT('Ctrl Pts',(-18.4514582369022,37.1379106262632,9.05155557322976));
#60800=CARTESIAN_POINT('Ctrl Pts',(-18.54164070453,37.1283401900378,9.00935234273155));
#60801=CARTESIAN_POINT('Ctrl Pts',(-18.5646405437834,37.1258436427352,8.99772304148919));
#60802=CARTESIAN_POINT('Ctrl Pts',(-18.6032779015198,37.12153948549,8.97668735854328));
#60803=CARTESIAN_POINT('Ctrl Pts',(-18.6190962389709,37.1197445470522,8.9676284267324));
#60804=CARTESIAN_POINT('Ctrl Pts',(-18.6515260036642,37.1159912799001,8.9481177176939));
#60805=CARTESIAN_POINT('Ctrl Pts',(-18.6681009036295,37.1140314756987,8.93761510959687));
#60806=CARTESIAN_POINT('Ctrl Pts',(-18.7130155425385,37.1085996118756,8.90767474987375));
#60807=CARTESIAN_POINT('Ctrl Pts',(-18.7408174193683,37.1050997086488,8.8874659504289));
#60808=CARTESIAN_POINT('Ctrl Pts',(-18.7822189556672,37.0996632089337,8.85472555352821));
#60809=CARTESIAN_POINT('Ctrl Pts',(-18.7964211951468,37.09775501192,8.8429829332296));
#60810=CARTESIAN_POINT('Ctrl Pts',(-18.8103598139481,37.0958383925403,8.83093838479897));
#60811=CARTESIAN_POINT('Origin',(-17.98,42.93984859951,7.87));
#60812=CARTESIAN_POINT('',(-18.8103594475449,36.1311618021068,8.83093870141285));
#60813=CARTESIAN_POINT('',(-18.8103597855904,36.3002088453023,8.83093840930324));
#60814=CARTESIAN_POINT('',(-18.810359785549,42.93984859951,8.83093840933902));
#60815=CARTESIAN_POINT('Ctrl Pts',(-18.8103594475449,36.1311618021068,8.83093870141285));
#60816=CARTESIAN_POINT('Ctrl Pts',(-18.7760032109335,36.1358942904264,8.86062636578764));
#60817=CARTESIAN_POINT('Ctrl Pts',(-18.7400620458144,36.1406769039139,8.88846536013866));
#60818=CARTESIAN_POINT('Ctrl Pts',(-18.6665241498893,36.1501062373779,8.93935421122266));
#60819=CARTESIAN_POINT('Ctrl Pts',(-18.6290854197678,36.1547435258644,8.96248450985219));
#60820=CARTESIAN_POINT('Ctrl Pts',(-18.5666796502928,36.1621596382488,8.9966970231326));
#60821=CARTESIAN_POINT('Ctrl Pts',(-18.5424227771892,36.1649699795933,9.00899962838746));
#60822=CARTESIAN_POINT('Ctrl Pts',(-18.5065938376522,36.1690012000212,9.02574719947508));
#60823=CARTESIAN_POINT('Ctrl Pts',(-18.4953241691024,36.1702524118464,9.03081596489765));
#60824=CARTESIAN_POINT('Ctrl Pts',(-18.4744338531305,36.1725389076545,9.03984758028955));
#60825=CARTESIAN_POINT('Ctrl Pts',(-18.4648362781758,36.1735765644151,9.04385774131803));
#60826=CARTESIAN_POINT('Ctrl Pts',(-18.4405426876497,36.176172958714,9.05365952841414));
#60827=CARTESIAN_POINT('Ctrl Pts',(-18.4257858197682,36.177722882049,9.05929581490953));
#60828=CARTESIAN_POINT('Ctrl Pts',(-18.3365431046723,36.1869573385961,9.09148671033355));
#60829=CARTESIAN_POINT('Ctrl Pts',(-18.2598022207941,36.1943296290845,9.11131709898632));
#60830=CARTESIAN_POINT('Ctrl Pts',(-18.1327162635908,36.2063876872943,9.13176046738748));
#60831=CARTESIAN_POINT('Ctrl Pts',(-18.0833139910934,36.2110381057285,9.13676254922227));
#60832=CARTESIAN_POINT('Ctrl Pts',(-17.9982701370895,36.2191322722624,9.1403649796513));
#60833=CARTESIAN_POINT('Ctrl Pts',(-17.9627481523514,36.2225390696275,9.14037901732945));
#60834=CARTESIAN_POINT('Ctrl Pts',(-17.9074823685278,36.2279170356055,9.13808266363422));
#60835=CARTESIAN_POINT('Ctrl Pts',(-17.887712503366,36.2298562566793,9.13679728417607));
#60836=CARTESIAN_POINT('Ctrl Pts',(-17.8498905258271,36.2336016819869,9.1334482166024));
#60837=CARTESIAN_POINT('Ctrl Pts',(-17.8318366519856,36.2354051003027,9.13145844408052));
#60838=CARTESIAN_POINT('Ctrl Pts',(-17.7887846573185,36.2397472464753,9.12577666432706));
#60839=CARTESIAN_POINT('Ctrl Pts',(-17.7638431566658,36.2422966907281,9.12172453951716));
#60840=CARTESIAN_POINT('Ctrl Pts',(-17.679209070971,36.2510740921771,9.10536973848571));
#60841=CARTESIAN_POINT('Ctrl Pts',(-17.6202977585061,36.2574055641937,9.08951847377857));
#60842=CARTESIAN_POINT('Ctrl Pts',(-17.4934166814106,36.2715171064884,9.04538383016372));
#60843=CARTESIAN_POINT('Ctrl Pts',(-17.4262930972196,36.2793054042464,9.01529466089719));
#60844=CARTESIAN_POINT('Ctrl Pts',(-17.341351115357,36.2894047168989,8.96799543251322));
#60845=CARTESIAN_POINT('Ctrl Pts',(-17.3208861168189,36.2918571169645,8.95583401132522));
#60846=CARTESIAN_POINT('Ctrl Pts',(-17.2907939889241,36.2954807764256,8.93678702139078));
#60847=CARTESIAN_POINT('Ctrl Pts',(-17.28090289296,36.296674781475,8.93033143375505));
#60848=CARTESIAN_POINT('Ctrl Pts',(-17.2624148785197,36.2989102097108,8.91789371109461));
#60849=CARTESIAN_POINT('Ctrl Pts',(-17.2538000170136,36.2999531653736,8.91194205118032));
#60850=CARTESIAN_POINT('Ctrl Pts',(-17.2314264828812,36.3026679140627,8.89607274675867));
#60851=CARTESIAN_POINT('Ctrl Pts',(-17.2177907841818,36.3043287141557,8.88598464924799));
#60852=CARTESIAN_POINT('Ctrl Pts',(-17.1600139109664,36.3114141695364,8.84142129025013));
#60853=CARTESIAN_POINT('Ctrl Pts',(-17.1179716125759,36.3166957952928,8.8043155506681));
#60854=CARTESIAN_POINT('Ctrl Pts',(-17.0344597503872,36.3278223543935,8.72015583011394));
#60855=CARTESIAN_POINT('Ctrl Pts',(-16.9937494427379,36.3336474510445,8.67257128352692));
#60856=CARTESIAN_POINT('Ctrl Pts',(-16.932750873755,36.3434033739125,8.58958726783062));
#60857=CARTESIAN_POINT('Ctrl Pts',(-16.9103648384086,36.3472697650717,8.55586914786252));
#60858=CARTESIAN_POINT('Ctrl Pts',(-16.8790825672184,36.3531900323301,8.50348546073653));
#60859=CARTESIAN_POINT('Ctrl Pts',(-16.868968657173,36.3551996631879,8.4855747388844));
#60860=CARTESIAN_POINT('Ctrl Pts',(-16.8508370113967,36.3589957492767,8.45156186212521));
#60861=CARTESIAN_POINT('Ctrl Pts',(-16.842717727256,36.360778041389,8.43551940891076));
#60862=CARTESIAN_POINT('Ctrl Pts',(-16.8248844867213,36.3648936738787,8.39834540484185));
#60863=CARTESIAN_POINT('Ctrl Pts',(-16.815405380893,36.3672344693827,8.3771093623447));
#60864=CARTESIAN_POINT('Ctrl Pts',(-16.7684350720293,36.3797052177042,8.26360876050272));
#60865=CARTESIAN_POINT('Ctrl Pts',(-16.7413191913173,36.3901731741449,8.16745199653552));
#60866=CARTESIAN_POINT('Ctrl Pts',(-16.7198013335341,36.4046364467897,8.03192471143991));
#60867=CARTESIAN_POINT('Ctrl Pts',(-16.715551042996,36.4086000772414,7.99445691334066));
#60868=CARTESIAN_POINT('Ctrl Pts',(-16.7112808195574,36.4150924192366,7.93216225369074));
#60869=CARTESIAN_POINT('Ctrl Pts',(-16.7103101997785,36.417645075277,7.90742438437514));
#60870=CARTESIAN_POINT('Ctrl Pts',(-16.7099437921364,36.4213836764688,7.87070262534822));
#60871=CARTESIAN_POINT('Ctrl Pts',(-16.7099935682663,36.4225944033524,7.85873193304394));
#60872=CARTESIAN_POINT('Ctrl Pts',(-16.7104029847268,36.4248402340662,7.83635944989056));
#60873=CARTESIAN_POINT('Ctrl Pts',(-16.7107211944244,36.4258771691182,7.82595913439992));
#60874=CARTESIAN_POINT('Ctrl Pts',(-16.7118761546103,36.4285452090779,7.79903913287394));
#60875=CARTESIAN_POINT('Ctrl Pts',(-16.7129078414682,36.4301660652106,7.78252948486991));
#60876=CARTESIAN_POINT('Ctrl Pts',(-16.7213640660259,36.4402060775442,7.6795696849324));
#60877=CARTESIAN_POINT('Ctrl Pts',(-16.7373104893162,36.4482561535016,7.59403559192311));
#60878=CARTESIAN_POINT('Ctrl Pts',(-16.7804213603706,36.4625466864285,7.4478421696924));
#60879=CARTESIAN_POINT('Ctrl Pts',(-16.8038296414844,36.4687257681357,7.38644299176103));
#60880=CARTESIAN_POINT('Ctrl Pts',(-16.8417186577963,36.4772828230211,7.30631026836668));
#60881=CARTESIAN_POINT('Ctrl Pts',(-16.8521281491136,36.4795230145532,7.28576079027428));
#60882=CARTESIAN_POINT('Ctrl Pts',(-16.8716234185066,36.483541935989,7.24973974122657));
#60883=CARTESIAN_POINT('Ctrl Pts',(-16.8804894038865,36.4853124733835,7.23415583583721));
#60884=CARTESIAN_POINT('Ctrl Pts',(-16.9004330995888,36.4891801170895,7.20076542760622));
#60885=CARTESIAN_POINT('Ctrl Pts',(-16.9116277377321,36.4912810919067,7.18303553278944));
#60886=CARTESIAN_POINT('Ctrl Pts',(-16.947280946252,36.4977730892262,7.12954898813671));
#60887=CARTESIAN_POINT('Ctrl Pts',(-16.9731311844644,36.5022141382845,7.09476426104615));
#60888=CARTESIAN_POINT('Ctrl Pts',(-17.0542058498415,36.515432345718,6.99657800580579));
#60889=CARTESIAN_POINT('Ctrl Pts',(-17.1140036382137,36.5243437943068,6.93725753258706));
#60890=CARTESIAN_POINT('Ctrl Pts',(-17.1937105809719,36.5351154723595,6.87250416097278));
#60891=CARTESIAN_POINT('Ctrl Pts',(-17.2084692493629,36.5370679645552,6.86104540608976));
#60892=CARTESIAN_POINT('Ctrl Pts',(-17.2425883293291,36.5414804686067,6.8357417089507));
#60893=CARTESIAN_POINT('Ctrl Pts',(-17.2620972415296,36.5439324632495,6.82210589399287));
#60894=CARTESIAN_POINT('Ctrl Pts',(-17.2918454986805,36.5475556558794,6.80253438398421));
#60895=CARTESIAN_POINT('Ctrl Pts',(-17.3018018906835,36.5487495914627,6.79618119622263));
#60896=CARTESIAN_POINT('Ctrl Pts',(-17.3207509222787,36.5509849778386,6.78445852412909));
#60897=CARTESIAN_POINT('Ctrl Pts',(-17.3297231980031,36.5520279598731,6.77906015743901));
#60898=CARTESIAN_POINT('Ctrl Pts',(-17.3534018553655,36.5547429091335,6.76520933282668));
#60899=CARTESIAN_POINT('Ctrl Pts',(-17.3682129302077,36.5564038802154,6.75693920273413));
#60900=CARTESIAN_POINT('Ctrl Pts',(-17.4329706837229,36.5635278503611,6.72246357545849));
#60901=CARTESIAN_POINT('Ctrl Pts',(-17.4844731961363,36.5688455902111,6.69930101277673));
#60902=CARTESIAN_POINT('Ctrl Pts',(-17.5957245972839,36.5799835431229,6.65793118292992));
#60903=CARTESIAN_POINT('Ctrl Pts',(-17.655611150837,36.5857847355562,6.64054898574749));
#60904=CARTESIAN_POINT('Ctrl Pts',(-17.756016332831,36.5955078325704,6.61925595475851));
#60905=CARTESIAN_POINT('Ctrl Pts',(-17.7958754378734,36.5993659364716,6.61277018895961));
#60906=CARTESIAN_POINT('Ctrl Pts',(-17.8563936059569,36.6052764719903,6.60586236908693));
#60907=CARTESIAN_POINT('Ctrl Pts',(-17.8768676471414,36.6072848966965,6.60402761101839));
#60908=CARTESIAN_POINT('Ctrl Pts',(-17.9153190570589,36.6110800058669,6.60152071172324));
#60909=CARTESIAN_POINT('Ctrl Pts',(-17.9332839154561,36.6128625496769,6.60073215906969));
#60910=CARTESIAN_POINT('Ctrl Pts',(-17.9745272144698,36.616980649529,6.59979853260095));
#60911=CARTESIAN_POINT('Ctrl Pts',(-17.9978041125463,36.619323694003,6.59991159810141));
#60912=CARTESIAN_POINT('Ctrl Pts',(-18.1204344292266,36.6317806000519,6.60387867263611));
#60913=CARTESIAN_POINT('Ctrl Pts',(-18.2190620238107,36.6422311019821,6.61875068662976));
#60914=CARTESIAN_POINT('Ctrl Pts',(-18.3513352873485,36.6566842686294,6.65491345216613));
#60915=CARTESIAN_POINT('Ctrl Pts',(-18.3872914584938,36.660654888521,6.66648877030307));
#60916=CARTESIAN_POINT('Ctrl Pts',(-18.4459025896686,36.6671569775445,6.68828573177479));
#60917=CARTESIAN_POINT('Ctrl Pts',(-18.4688693719524,36.6697124681243,6.69760039175516));
#60918=CARTESIAN_POINT('Ctrl Pts',(-18.5025107421543,36.6734543103898,6.71240512469698));
#60919=CARTESIAN_POINT('Ctrl Pts',(-18.5134022439764,36.6746655023689,6.71738321272107));
#60920=CARTESIAN_POINT('Ctrl Pts',(-18.5336223757166,36.6769116378522,6.72697309818867));
#60921=CARTESIAN_POINT('Ctrl Pts',(-18.5429667962665,36.6779484208179,6.73154638400424));
#60922=CARTESIAN_POINT('Ctrl Pts',(-18.5670098423513,36.6806152407229,6.7436818333025));
#60923=CARTESIAN_POINT('Ctrl Pts',(-18.5816191997031,36.682235048308,6.75141714506561));
#60924=CARTESIAN_POINT('Ctrl Pts',(-18.6584308453281,36.6907720149526,6.7940276699261));
#60925=CARTESIAN_POINT('Ctrl Pts',(-18.7177741761424,36.697444189274,6.83381580102478));
#60926=CARTESIAN_POINT('Ctrl Pts',(-18.815132955538,36.7091245454212,6.91172029292294));
#60927=CARTESIAN_POINT('Ctrl Pts',(-18.8546496865709,36.7141155853043,6.94764737446438));
#60928=CARTESIAN_POINT('Ctrl Pts',(-18.9040380298795,36.7208535324526,6.99858540022494));
#60929=CARTESIAN_POINT('Ctrl Pts',(-18.9160234459164,36.7225319489762,7.01147234238413));
#60930=CARTESIAN_POINT('Ctrl Pts',(-18.9459342833522,36.7268417131067,7.0450040658457));
#60931=CARTESIAN_POINT('Ctrl Pts',(-18.9634667487566,36.7294851769108,7.06598493182892));
#60932=CARTESIAN_POINT('Ctrl Pts',(-18.9916837909836,36.7339599183775,7.10205674509178));
#60933=CARTESIAN_POINT('Ctrl Pts',(-19.0027410145245,36.7357758196871,7.11684552463702));
#60934=CARTESIAN_POINT('Ctrl Pts',(-19.0246154234862,36.7395037696631,7.147472305832));
#60935=CARTESIAN_POINT('Ctrl Pts',(-19.0354039914933,36.7414163357991,7.16332471172732));
#60936=CARTESIAN_POINT('Ctrl Pts',(-19.0630397868396,36.7465229047993,7.20597694503014));
#60937=CARTESIAN_POINT('Ctrl Pts',(-19.0792496286243,36.7497391133778,7.2331706641325));
#60938=CARTESIAN_POINT('Ctrl Pts',(-19.1423151442754,36.7632439823326,7.34856425988581));
#60939=CARTESIAN_POINT('Ctrl Pts',(-19.1796962098748,36.7738260823295,7.44152145546702));
#60940=CARTESIAN_POINT('Ctrl Pts',(-19.2162205907252,36.7884906932312,7.57632370855713));
#60941=CARTESIAN_POINT('Ctrl Pts',(-19.2248254610046,36.7926447903531,7.61525007202022));
#60942=CARTESIAN_POINT('Ctrl Pts',(-19.2339396686859,36.7981420328911,7.6681890779298));
#60943=CARTESIAN_POINT('Ctrl Pts',(-19.2360688944358,36.7995516734352,7.68189541813096));
#60944=CARTESIAN_POINT('Ctrl Pts',(-19.2393799416035,36.801981944899,7.70578328299771));
#60945=CARTESIAN_POINT('Ctrl Pts',(-19.2406637402371,36.8030075876296,7.71594828667188));
#60946=CARTESIAN_POINT('Ctrl Pts',(-19.2433485954974,36.8053642413517,7.73949589881412));
#60947=CARTESIAN_POINT('Ctrl Pts',(-19.2446602789099,36.8066904720259,7.75288710938346));
#60948=CARTESIAN_POINT('Ctrl Pts',(-19.2485592397566,36.8113627458836,7.80047663378449));
#60949=CARTESIAN_POINT('Ctrl Pts',(-19.2499743351078,36.8146540256962,7.83475976305547));
#60950=CARTESIAN_POINT('Ctrl Pts',(-19.2500519035659,36.824636717189,7.93985156011914));
#60951=CARTESIAN_POINT('Ctrl Pts',(-19.2441855365075,36.831207695006,8.01052479332583));
#60952=CARTESIAN_POINT('Ctrl Pts',(-19.22340539874,36.8430010474847,8.13425649880132));
#60953=CARTESIAN_POINT('Ctrl Pts',(-19.2108809647212,36.8481755539421,8.18752030191754));
#60954=CARTESIAN_POINT('Ctrl Pts',(-19.1883646708274,36.855645412525,8.26149563942603));
#60955=CARTESIAN_POINT('Ctrl Pts',(-19.1811838583637,36.8578517613901,8.28300266001613));
#60956=CARTESIAN_POINT('Ctrl Pts',(-19.1673080719994,36.8618349743332,8.32113214818977));
#60957=CARTESIAN_POINT('Ctrl Pts',(-19.1608294475418,36.8636042242597,8.33782732498489));
#60958=CARTESIAN_POINT('Ctrl Pts',(-19.1459026756098,36.8674978471416,8.37400568988059));
#60959=CARTESIAN_POINT('Ctrl Pts',(-19.1373146579057,36.8696265229225,8.39342470950591));
#60960=CARTESIAN_POINT('Ctrl Pts',(-19.1088685512598,36.8763547816825,8.45362008689353));
#60961=CARTESIAN_POINT('Ctrl Pts',(-19.0873133438803,36.8810102182459,8.49354834798456));
#60962=CARTESIAN_POINT('Ctrl Pts',(-19.0221745438445,36.8939970525749,8.60014094800772));
#60963=CARTESIAN_POINT('Ctrl Pts',(-18.9743868951971,36.9024325342042,8.66399384338684));
#60964=CARTESIAN_POINT('Ctrl Pts',(-18.8954487372901,36.9147678068031,8.75107599236373));
#60965=CARTESIAN_POINT('Ctrl Pts',(-18.8686995537025,36.9187243933491,8.77805018368966));
#60966=CARTESIAN_POINT('Ctrl Pts',(-18.8314356661918,36.9239132717192,8.81240053399039));
#60967=CARTESIAN_POINT('Ctrl Pts',(-18.8219634640118,36.9252062244695,8.82087277333503));
#60968=CARTESIAN_POINT('Ctrl Pts',(-18.8116972203454,36.9265787637597,8.82978149360303));
#60969=CARTESIAN_POINT('Ctrl Pts',(-18.8110288055181,36.9266679984251,8.83036030019834));
#60970=CARTESIAN_POINT('Ctrl Pts',(-18.8103597855476,36.9267571849074,8.8309384093402));
#60971=CARTESIAN_POINT('',(-19.2499996068732,36.9878745608382,7.86961352183627));
#60972=CARTESIAN_POINT('Ctrl Pts',(-18.8103598139481,37.0958383925403,8.83093838479897));
#60973=CARTESIAN_POINT('Ctrl Pts',(-18.8319720210683,37.0928666221235,8.81226298524454));
#60974=CARTESIAN_POINT('Ctrl Pts',(-18.8529504390839,37.0898744369893,8.79286172526314));
#60975=CARTESIAN_POINT('Ctrl Pts',(-18.9336583541334,37.0779359743146,8.7130038368293));
#60976=CARTESIAN_POINT('Ctrl Pts',(-18.9879122389735,37.0689120322178,8.64732566049202));
#60977=CARTESIAN_POINT('Ctrl Pts',(-19.0436375522878,37.0586355077117,8.56412167096038));
#60978=CARTESIAN_POINT('Ctrl Pts',(-19.051846569037,37.0570909975101,8.55137709473417));
#60979=CARTESIAN_POINT('Ctrl Pts',(-19.0652601489183,37.0545178365129,8.52970977537145));
#60980=CARTESIAN_POINT('Ctrl Pts',(-19.0705872504396,37.0534820359881,8.52086562805951));
#60981=CARTESIAN_POINT('Ctrl Pts',(-19.0822267884411,37.0511877479046,8.50099717080175));
#60982=CARTESIAN_POINT('Ctrl Pts',(-19.0884827183789,37.0499326935896,8.48994147638588));
#60983=CARTESIAN_POINT('Ctrl Pts',(-19.1087523403626,37.0457844537475,8.45283205091759));
#60984=CARTESIAN_POINT('Ctrl Pts',(-19.1220229756091,37.0429316585472,8.42638027973928));
#60985=CARTESIAN_POINT('Ctrl Pts',(-19.1678390072408,37.0324436691517,8.32649440535921));
#60986=CARTESIAN_POINT('Ctrl Pts',(-19.19432319928,37.0250086207334,8.25048651960703));
#60987=CARTESIAN_POINT('Ctrl Pts',(-19.226133415198,37.0124454450672,8.12077120684708));
#60988=CARTESIAN_POINT('Ctrl Pts',(-19.2355483171846,37.0073998726599,8.06832241853931));
#60989=CARTESIAN_POINT('Ctrl Pts',(-19.2441503099887,37.0001387262449,7.99370466318839));
#60990=CARTESIAN_POINT('Ctrl Pts',(-19.2460939025166,36.9980080974401,7.97190652745627));
#60991=CARTESIAN_POINT('Ctrl Pts',(-19.248375596739,36.9944547171614,7.93578857165217));
#60992=CARTESIAN_POINT('Ctrl Pts',(-19.2490363322088,36.9930423515387,7.92149306712338));
#60993=CARTESIAN_POINT('Ctrl Pts',(-19.2498222302058,36.9903789954949,7.89466709662065));
#60994=CARTESIAN_POINT('Ctrl Pts',(-19.2500037603679,36.9891299547276,7.88213994300183));
#60995=CARTESIAN_POINT('Ctrl Pts',(-19.249999940972,36.9878750685577,7.8696127904914));
#60996=CARTESIAN_POINT('Ctrl Pts',(-19.2499999411772,36.9878751360372,7.86961346411839));
#60997=CARTESIAN_POINT('Ctrl Pts',(-19.2499965846628,36.9867704107569,7.85858532092341));
#60998=CARTESIAN_POINT('Ctrl Pts',(-19.2498495830066,36.9856612471189,7.84755807683458));
#60999=CARTESIAN_POINT('Ctrl Pts',(-19.2491498541977,36.9829796419562,7.82101290712289));
#61000=CARTESIAN_POINT('Ctrl Pts',(-19.2484561139684,36.9814030655816,7.8055009975196));
#61001=CARTESIAN_POINT('Ctrl Pts',(-19.2438792737663,36.9739852733063,7.73298200009193));
#61002=CARTESIAN_POINT('Ctrl Pts',(-19.2364367565112,36.9680436948589,7.67627503906745));
#61003=CARTESIAN_POINT('Ctrl Pts',(-19.2124017841134,36.9552042403979,7.55643159503664));
#61004=CARTESIAN_POINT('Ctrl Pts',(-19.194708435252,36.9483056553954,7.49367172570919));
#61005=CARTESIAN_POINT('Ctrl Pts',(-19.1621005153993,36.9384226686289,7.40479917747777));
#61006=CARTESIAN_POINT('Ctrl Pts',(-19.1509539363258,36.9353619356922,7.37741424108688));
#61007=CARTESIAN_POINT('Ctrl Pts',(-19.1336659123885,36.9310503252874,7.33885389153321));
#61008=CARTESIAN_POINT('Ctrl Pts',(-19.1282974868712,36.9297632856597,7.32734527042008));
#61009=CARTESIAN_POINT('Ctrl Pts',(-19.1182523236134,36.9274483076655,7.3066277850696));
#61010=CARTESIAN_POINT('Ctrl Pts',(-19.1136347658349,36.9264173753027,7.29739294312918));
#61011=CARTESIAN_POINT('Ctrl Pts',(-19.1019581781109,36.9238888750732,7.2747355433121));
#61012=CARTESIAN_POINT('Ctrl Pts',(-19.0947704441636,36.9223990363303,7.26138118585587));
#61013=CARTESIAN_POINT('Ctrl Pts',(-19.045771323413,36.9126448405902,7.17412608831189));
#61014=CARTESIAN_POINT('Ctrl Pts',(-18.9968703820359,36.904750227946,7.10443533384081));
#61015=CARTESIAN_POINT('Ctrl Pts',(-18.9106393858459,36.8923842792171,7.00453951579789));
#61016=CARTESIAN_POINT('Ctrl Pts',(-18.8779592717906,36.8879698200049,6.97067798306193));
#61017=CARTESIAN_POINT('Ctrl Pts',(-18.8182752023877,36.880222443173,6.91533984828336));
#61018=CARTESIAN_POINT('Ctrl Pts',(-18.7921358784013,36.8769218546092,6.89300656591906));
#61019=CARTESIAN_POINT('Ctrl Pts',(-18.7497019600452,36.8716700801893,6.85963177919455));
#61020=CARTESIAN_POINT('Ctrl Pts',(-18.7340003008718,36.8697482624859,6.84786082627717));
#61021=CARTESIAN_POINT('Ctrl Pts',(-18.7031998642669,36.8660133356724,6.82586677827817));
#61022=CARTESIAN_POINT('Ctrl Pts',(-18.6881411277803,36.8642026506752,6.8155957686715));
#61023=CARTESIAN_POINT('Ctrl Pts',(-18.6512752160318,36.8598020116876,6.79159683310471));
#61024=CARTESIAN_POINT('Ctrl Pts',(-18.6292622601431,36.857200518078,6.77820236505293));
#61025=CARTESIAN_POINT('Ctrl Pts',(-18.5411130850893,36.846871712437,6.72817383691675));
#61026=CARTESIAN_POINT('Ctrl Pts',(-18.4721800310458,36.8389725444363,6.69681236288029));
#61027=CARTESIAN_POINT('Ctrl Pts',(-18.3539279884323,36.825765135631,6.6552758874112));
#61028=CARTESIAN_POINT('Ctrl Pts',(-18.306042034625,36.8205074399493,6.64155633658014));
#61029=CARTESIAN_POINT('Ctrl Pts',(-18.2289893129242,36.8122663172098,6.62430489833243));
#61030=CARTESIAN_POINT('Ctrl Pts',(-18.2002911785705,36.8092442958246,6.61891080832345));
#61031=CARTESIAN_POINT('Ctrl Pts',(-18.1589274997324,36.8049758201063,6.61260392848126));
#61032=CARTESIAN_POINT('Ctrl Pts',(-18.1463968982248,36.8036941323454,6.61088441732415));
#61033=CARTESIAN_POINT('Ctrl Pts',(-18.1235837949876,36.8013836367081,6.60810044484617));
#61034=CARTESIAN_POINT('Ctrl Pts',(-18.1133113281566,36.8003519260606,6.60697391078077));
#61035=CARTESIAN_POINT('Ctrl Pts',(-18.0878478801805,36.7978143589703,6.6044956105997));
#61036=CARTESIAN_POINT('Ctrl Pts',(-18.0726441743024,36.7963163784605,6.60329180145362));
#61037=CARTESIAN_POINT('Ctrl Pts',(-17.9734381348069,36.7866304226467,6.59723277575915));
#61038=CARTESIAN_POINT('Ctrl Pts',(-17.889136446353,36.7788042788842,6.6004612007624));
#61039=CARTESIAN_POINT('Ctrl Pts',(-17.75885068255,36.7664798629953,6.61850661117242));
#61040=CARTESIAN_POINT('Ctrl Pts',(-17.7123447526007,36.7620352579744,6.62762211250088));
#61041=CARTESIAN_POINT('Ctrl Pts',(-17.6330090251657,36.7542433367545,6.64783438041513));
#61042=CARTESIAN_POINT('Ctrl Pts',(-17.599923818932,36.7509289237941,6.65771572445393));
#61043=CARTESIAN_POINT('Ctrl Pts',(-17.548704610305,36.7456607506856,6.67531582102457));
#61044=CARTESIAN_POINT('Ctrl Pts',(-17.5302760585709,36.7437366895387,6.68213036401836));
#61045=CARTESIAN_POINT('Ctrl Pts',(-17.4950787970975,36.7400005583082,6.69608207351858));
#61046=CARTESIAN_POINT('Ctrl Pts',(-17.4782909843485,36.7381909608358,6.7031581742054));
#61047=CARTESIAN_POINT('Ctrl Pts',(-17.4382055969771,36.733798626898,6.72107919684498));
#61048=CARTESIAN_POINT('Ctrl Pts',(-17.4150749112923,36.7312044668707,6.73227438049718));
#61049=CARTESIAN_POINT('Ctrl Pts',(-17.32281674823,36.7206001061223,6.78043404352908));
#61050=CARTESIAN_POINT('Ctrl Pts',(-17.2568533111328,36.7124025328118,6.82305312611031));
#61051=CARTESIAN_POINT('Ctrl Pts',(-17.1575295160172,36.6990870299596,6.90111200220858));
#61052=CARTESIAN_POINT('Ctrl Pts',(-17.1215172754823,36.6940212556487,6.93287167003138));
#61053=CARTESIAN_POINT('Ctrl Pts',(-17.0670477381074,36.6860329509701,6.98669048042444));
#61054=CARTESIAN_POINT('Ctrl Pts',(-17.0473905541815,36.6830740099175,7.00747026362907));
#61055=CARTESIAN_POINT('Ctrl Pts',(-17.0201302959756,36.6788760069471,7.03831018765475));
#61056=CARTESIAN_POINT('Ctrl Pts',(-17.0119504435492,36.6776032032986,7.04784557682713));
#61057=CARTESIAN_POINT('Ctrl Pts',(-16.99729089639,36.6753000145867,7.06545668032291));
#61058=CARTESIAN_POINT('Ctrl Pts',(-16.9907667213301,36.6742668789043,7.07349220079844));
#61059=CARTESIAN_POINT('Ctrl Pts',(-16.9747832282539,36.6717136155761,7.09367772513725));
#61060=CARTESIAN_POINT('Ctrl Pts',(-16.9654452237085,36.6702016169602,7.10592165387163));
#61061=CARTESIAN_POINT('Ctrl Pts',(-16.9073302830408,36.6606358596699,7.18506636991105));
#61062=CARTESIAN_POINT('Ctrl Pts',(-16.8649623719828,36.6529302928472,7.2564441831153));
#61063=CARTESIAN_POINT('Ctrl Pts',(-16.8095085789184,36.6406780216269,7.37487495377104));
#61064=CARTESIAN_POINT('Ctrl Pts',(-16.7916530830842,36.6361796085125,7.41941149503553));
#61065=CARTESIAN_POINT('Ctrl Pts',(-16.7652630475786,36.6283083658968,7.49781204108717));
#61066=CARTESIAN_POINT('Ctrl Pts',(-16.7555272425671,36.6249694765985,7.53121433434715));
#61067=CARTESIAN_POINT('Ctrl Pts',(-16.7424460264537,36.6196722749313,7.58408419675772));
#61068=CARTESIAN_POINT('Ctrl Pts',(-16.7381624142675,36.6177442512461,7.60330356405425));
#61069=CARTESIAN_POINT('Ctrl Pts',(-16.7307821959593,36.6140059355288,7.64046538635637));
#61070=CARTESIAN_POINT('Ctrl Pts',(-16.7276212725735,36.6121982010891,7.65839022750838));
#61071=CARTESIAN_POINT('Ctrl Pts',(-16.7209479723695,36.6078201962696,7.70164931981465));
#61072=CARTESIAN_POINT('Ctrl Pts',(-16.717813795412,36.6052387022558,7.72703251360151));
#61073=CARTESIAN_POINT('Ctrl Pts',(-16.7079743168088,36.594405074193,7.83291804248522));
#61074=CARTESIAN_POINT('Ctrl Pts',(-16.7081920118968,36.5859514542183,7.91385810299549));
#61075=CARTESIAN_POINT('Ctrl Pts',(-16.7206417298067,36.5725320596853,8.04053950811451));
#61076=CARTESIAN_POINT('Ctrl Pts',(-16.72773854774,36.5676188879509,8.08658412378216));
#61077=CARTESIAN_POINT('Ctrl Pts',(-16.7431489026897,36.5598331295398,8.15963634933817));
#61078=CARTESIAN_POINT('Ctrl Pts',(-16.74986174569,36.5569258739288,8.18693863095968));
#61079=CARTESIAN_POINT('Ctrl Pts',(-16.760859265411,36.5527857859602,8.22602230908645));
#61080=CARTESIAN_POINT('Ctrl Pts',(-16.7644199847385,36.5515204140374,8.23799631485117));
#61081=CARTESIAN_POINT('Ctrl Pts',(-16.7712579769957,36.549223202445,8.25980786643985));
#61082=CARTESIAN_POINT('Ctrl Pts',(-16.7744797254456,36.5481887401527,8.26966027626384));
#61083=CARTESIAN_POINT('Ctrl Pts',(-16.7828275022103,36.5456216919705,8.29416861512221));
#61084=CARTESIAN_POINT('Ctrl Pts',(-16.7881022984624,36.5440974564466,8.30877209899046));
#61085=CARTESIAN_POINT('Ctrl Pts',(-16.8227655921861,36.5346385604852,8.39949600316182));
#61086=CARTESIAN_POINT('Ctrl Pts',(-16.8591704031109,36.5270402547169,8.47274668098409));
#61087=CARTESIAN_POINT('Ctrl Pts',(-16.9280137570396,36.5148512223854,8.58314461087094));
#61088=CARTESIAN_POINT('Ctrl Pts',(-16.9559988727532,36.5103043101985,8.62277579333392));
#61089=CARTESIAN_POINT('Ctrl Pts',(-17.0079798538298,36.5023617768724,8.68810936894841));
#61090=CARTESIAN_POINT('Ctrl Pts',(-17.0309023673747,36.4990010438652,8.71459416298967));
#61091=CARTESIAN_POINT('Ctrl Pts',(-17.0684031917117,36.4936779423883,8.75446619112779));
#61092=CARTESIAN_POINT('Ctrl Pts',(-17.0822509992118,36.4917463930899,8.7685186750782));
#61093=CARTESIAN_POINT('Ctrl Pts',(-17.1094827118223,36.488006074352,8.79489479950156));
#61094=CARTESIAN_POINT('Ctrl Pts',(-17.1228152650211,36.4861999374116,8.80726462721867));
#61095=CARTESIAN_POINT('Ctrl Pts',(-17.1554451824731,36.4818343297839,8.83625976931501));
#61096=CARTESIAN_POINT('Ctrl Pts',(-17.1749851060158,36.479263808138,8.85259827481995));
#61097=CARTESIAN_POINT('Ctrl Pts',(-17.2597175161819,36.4682844937013,8.91922391837642));
#61098=CARTESIAN_POINT('Ctrl Pts',(-17.3292149065797,36.4596646582141,8.96368681569382));
#61099=CARTESIAN_POINT('Ctrl Pts',(-17.4431878199489,36.4461729472117,9.0218762634079));
#61100=CARTESIAN_POINT('Ctrl Pts',(-17.4849609601666,36.441353546678,9.04043711651855));
#61101=CARTESIAN_POINT('Ctrl Pts',(-17.5536199042152,36.4336929386438,9.066608841916));
#61102=CARTESIAN_POINT('Ctrl Pts',(-17.5799155932922,36.4308181332423,9.07565564446893));
#61103=CARTESIAN_POINT('Ctrl Pts',(-17.6183849679454,36.426714486714,9.08749310323339));
#61104=CARTESIAN_POINT('Ctrl Pts',(-17.6303339956639,36.4254538515313,9.09097854967112));
#61105=CARTESIAN_POINT('Ctrl Pts',(-17.6523359699693,36.4231603816222,9.097046841018));
#61106=CARTESIAN_POINT('Ctrl Pts',(-17.6623717367259,36.4221250062126,9.09968287401341));
#61107=CARTESIAN_POINT('Ctrl Pts',(-17.6875841674417,36.4195488420825,9.10597597755617));
#61108=CARTESIAN_POINT('Ctrl Pts',(-17.7027980894775,36.4180165496863,9.10947683338117));
#61109=CARTESIAN_POINT('Ctrl Pts',(-17.7971363448254,36.4086284813153,9.12936072449991));
#61110=CARTESIAN_POINT('Ctrl Pts',(-17.8776239742299,36.4011013495125,9.13844496382321));
#61111=CARTESIAN_POINT('Ctrl Pts',(-18.0072709902384,36.3889538622936,9.14064598757898));
#61112=CARTESIAN_POINT('Ctrl Pts',(-18.0561033284103,36.3843745128559,9.13865780454879));
#61113=CARTESIAN_POINT('Ctrl Pts',(-18.1396985224861,36.3763844063414,9.13041001537733));
#61114=CARTESIAN_POINT('Ctrl Pts',(-18.1745375629788,36.3730091784098,9.1255045472892));
#61115=CARTESIAN_POINT('Ctrl Pts',(-18.2285537059165,36.3676688940035,9.11559673799094));
#61116=CARTESIAN_POINT('Ctrl Pts',(-18.2478953351182,36.3657350109207,9.1115805093617));
#61117=CARTESIAN_POINT('Ctrl Pts',(-18.2848405354528,36.3619933362698,9.10300553632668));
#61118=CARTESIAN_POINT('Ctrl Pts',(-18.302455407725,36.3601882264317,9.09851651474221));
#61119=CARTESIAN_POINT('Ctrl Pts',(-18.3444389857517,36.3558306483336,9.08685222768028));
#61120=CARTESIAN_POINT('Ctrl Pts',(-18.3686993613928,36.3532672408232,9.079321167836));
#61121=CARTESIAN_POINT('Ctrl Pts',(-18.4529635048526,36.3441925586253,9.05036601957254));
#61122=CARTESIAN_POINT('Ctrl Pts',(-18.5115569067452,36.3375662304837,9.02516353539409));
#61123=CARTESIAN_POINT('Ctrl Pts',(-18.630387694666,36.3234718212738,8.96309175365081));
#61124=CARTESIAN_POINT('Ctrl Pts',(-18.6899572876904,36.3160106517275,8.92537443526061));
#61125=CARTESIAN_POINT('Ctrl Pts',(-18.7650544803624,36.3062300926824,8.86857619830278));
#61126=CARTESIAN_POINT('Ctrl Pts',(-18.7836076873836,36.303780808727,8.85370721682863));
#61127=CARTESIAN_POINT('Ctrl Pts',(-18.8046205043817,36.3009767161073,8.83587543275746));
#61128=CARTESIAN_POINT('Ctrl Pts',(-18.8074956526641,36.3005923650223,8.83341334503232));
#61129=CARTESIAN_POINT('Ctrl Pts',(-18.8103597855904,36.3002088453023,8.83093840930324));
#61130=CARTESIAN_POINT('Origin',(-17.98,42.93984859951,7.87));
#61131=CARTESIAN_POINT('',(-18.8103597331144,35.3371716890844,8.83093845464843));
#61132=CARTESIAN_POINT('',(-18.8103598667433,35.5078191442546,8.83093833917793));
#61133=CARTESIAN_POINT('',(-18.810359785549,42.93984859951,8.83093840933902));
#61134=CARTESIAN_POINT('',(-19.249999602058,36.0238536116147,7.87100537183017));
#61135=CARTESIAN_POINT('Ctrl Pts',(-18.8103597331144,35.3371716890844,8.83093845464842));
#61136=CARTESIAN_POINT('Ctrl Pts',(-18.8029956697976,35.3381039032762,8.83730183996292));
#61137=CARTESIAN_POINT('Ctrl Pts',(-18.7955565796168,35.3390391032005,8.8435821986446));
#61138=CARTESIAN_POINT('Ctrl Pts',(-18.7713328197171,35.3420651495102,8.86356004602031));
#61139=CARTESIAN_POINT('Ctrl Pts',(-18.7542732367335,35.3441671036122,8.87691112805407));
#61140=CARTESIAN_POINT('Ctrl Pts',(-18.7222434781508,35.3480696082538,8.90068274911866));
#61141=CARTESIAN_POINT('Ctrl Pts',(-18.7073739413221,35.3498647060492,8.91122974093067));
#61142=CARTESIAN_POINT('Ctrl Pts',(-18.6760355446539,35.3536185461378,8.93245925463771));
#61143=CARTESIAN_POINT('Ctrl Pts',(-18.6595358478061,35.3555787676672,8.94308716685412));
#61144=CARTESIAN_POINT('Ctrl Pts',(-18.6134743921102,35.3610126113409,8.9712683202844));
#61145=CARTESIAN_POINT('Ctrl Pts',(-18.5834385311958,35.3645141104188,8.98800853788757));
#61146=CARTESIAN_POINT('Ctrl Pts',(-18.5107815449443,35.3728988762175,9.02472227621389));
#61147=CARTESIAN_POINT('Ctrl Pts',(-18.4676577743919,35.3778103169822,9.04358487544163));
#61148=CARTESIAN_POINT('Ctrl Pts',(-18.3440389127559,35.3916826599067,9.0896654591862));
#61149=CARTESIAN_POINT('Ctrl Pts',(-18.2617063306697,35.4006992645921,9.11127041491082));
#61150=CARTESIAN_POINT('Ctrl Pts',(-18.1628460393603,35.4109699236396,9.12686011022758));
#61151=CARTESIAN_POINT('Ctrl Pts',(-18.1478226825295,35.4125153797218,9.12895418272427));
#61152=CARTESIAN_POINT('Ctrl Pts',(-18.1225131219588,35.4150897212408,9.13202085461177));
#61153=CARTESIAN_POINT('Ctrl Pts',(-18.112246771305,35.4161257696643,9.13313794059962));
#61154=CARTESIAN_POINT('Ctrl Pts',(-18.0893249091597,35.418420224268,9.13534950290855));
#61155=CARTESIAN_POINT('Ctrl Pts',(-18.0766646765985,35.4196752017724,9.13637959906825));
#61156=CARTESIAN_POINT('Ctrl Pts',(-18.0344920141824,35.4238215958568,9.13917476513125));
#61157=CARTESIAN_POINT('Ctrl Pts',(-18.0049307616604,35.42667267917,9.14009955023809));
#61158=CARTESIAN_POINT('Ctrl Pts',(-17.9244403009356,35.4343547962777,9.1398055063515));
#61159=CARTESIAN_POINT('Ctrl Pts',(-17.8735728240804,35.4391227063776,9.13655716953619));
#61160=CARTESIAN_POINT('Ctrl Pts',(-17.7496979184924,35.4508161047859,9.12112850845784));
#61161=CARTESIAN_POINT('Ctrl Pts',(-17.6773085518082,35.4577276824075,9.10561213661262));
#61162=CARTESIAN_POINT('Ctrl Pts',(-17.5820503463708,35.4673069610003,9.0763168395228));
#61163=CARTESIAN_POINT('Ctrl Pts',(-17.5576545089222,35.4698038877865,9.06799345243712));
#61164=CARTESIAN_POINT('Ctrl Pts',(-17.5164624164574,35.4741088464869,9.05252497425862));
#61165=CARTESIAN_POINT('Ctrl Pts',(-17.4995353348952,35.4759042050252,9.04574913369533));
#61166=CARTESIAN_POINT('Ctrl Pts',(-17.4647004079522,35.4796585465066,9.03092703092976));
#61167=CARTESIAN_POINT('Ctrl Pts',(-17.4468217270627,35.4816190081759,9.02282525080045));
#61168=CARTESIAN_POINT('Ctrl Pts',(-17.3981610543737,35.4870535516632,8.99940049174118));
#61169=CARTESIAN_POINT('Ctrl Pts',(-17.367805238143,35.4905555138391,8.98323808586637));
#61170=CARTESIAN_POINT('Ctrl Pts',(-17.2975490308109,35.4989417154952,8.94208868379074));
#61171=CARTESIAN_POINT('Ctrl Pts',(-17.2583099030781,35.5038541378178,8.91607641032244));
#61172=CARTESIAN_POINT('Ctrl Pts',(-17.1525867695386,35.5177235100106,8.83720692267497));
#61173=CARTESIAN_POINT('Ctrl Pts',(-17.0898175600356,35.5267359911759,8.77976900616148));
#61174=CARTESIAN_POINT('Ctrl Pts',(-17.0231318561428,35.5370032824597,8.70518470306968));
#61175=CARTESIAN_POINT('Ctrl Pts',(-17.0132230894874,35.5385491513627,8.69369449099255));
#61176=CARTESIAN_POINT('Ctrl Pts',(-16.9969186064675,35.5411240291385,8.67408807170242));
#61177=CARTESIAN_POINT('Ctrl Pts',(-16.9904121689215,35.5421602058701,8.66606696708533));
#61178=CARTESIAN_POINT('Ctrl Pts',(-16.9761238419704,35.5444547445802,8.6480063936147));
#61179=CARTESIAN_POINT('Ctrl Pts',(-16.9683934507036,35.5457096803836,8.63792807407111));
#61180=CARTESIAN_POINT('Ctrl Pts',(-16.9431783347996,35.5498557426464,8.60401268460402));
#61181=CARTESIAN_POINT('Ctrl Pts',(-16.9263729915382,35.5527065446568,8.57967905411403));
#61182=CARTESIAN_POINT('Ctrl Pts',(-16.8829791824265,35.5603875253468,8.51190131502678));
#61183=CARTESIAN_POINT('Ctrl Pts',(-16.858128629912,35.5651546029993,8.46740899265991));
#61184=CARTESIAN_POINT('Ctrl Pts',(-16.8039153275726,35.5768481598991,8.35496188064153));
#61185=CARTESIAN_POINT('Ctrl Pts',(-16.7776933687063,35.5837607076116,8.28571603037241));
#61186=CARTESIAN_POINT('Ctrl Pts',(-16.7506495586745,35.5933409564831,8.18978383798157));
#61187=CARTESIAN_POINT('Ctrl Pts',(-16.7444140584049,35.5958378199638,8.16477342713037));
#61188=CARTESIAN_POINT('Ctrl Pts',(-16.7350739721055,35.6001426482953,8.12177681882658));
#61189=CARTESIAN_POINT('Ctrl Pts',(-16.7315882065427,35.6019379398526,8.10388092929744));
#61190=CARTESIAN_POINT('Ctrl Pts',(-16.7251522593938,35.605692110058,8.06657656947097));
#61191=CARTESIAN_POINT('Ctrl Pts',(-16.7222645201945,35.6076524669644,8.0471625003438));
#61192=CARTESIAN_POINT('Ctrl Pts',(-16.71555945905,35.6130865515487,7.99357955754699));
#61193=CARTESIAN_POINT('Ctrl Pts',(-16.7126782946446,35.616588154165,7.95931358674854));
#61194=CARTESIAN_POINT('Ctrl Pts',(-16.70915422217,35.6249731437658,7.8779816692115));
#61195=CARTESIAN_POINT('Ctrl Pts',(-16.7097307103118,35.629884702584,7.83091533601337));
#61196=CARTESIAN_POINT('Ctrl Pts',(-16.7186646166168,35.6437564561438,7.69929521739378));
#61197=CARTESIAN_POINT('Ctrl Pts',(-16.7328922086987,35.652772319966,7.61537917200997));
#61198=CARTESIAN_POINT('Ctrl Pts',(-16.7594082120656,35.6630424204436,7.51887932323717));
#61199=CARTESIAN_POINT('Ctrl Pts',(-16.7636888660913,35.6645879821681,7.50432617793841));
#61200=CARTESIAN_POINT('Ctrl Pts',(-16.7713206211406,35.6671624774018,7.4799989787617));
#61201=CARTESIAN_POINT('Ctrl Pts',(-16.7745318614785,35.6681985749207,7.47018348886641));
#61202=CARTESIAN_POINT('Ctrl Pts',(-16.7819589917268,35.6704930831391,7.44838519445449));
#61203=CARTESIAN_POINT('Ctrl Pts',(-16.7862354811186,35.671748065688,7.436424604497));
#61204=CARTESIAN_POINT('Ctrl Pts',(-16.8010612671239,35.6758946422749,7.39684301050707));
#61205=CARTESIAN_POINT('Ctrl Pts',(-16.812396474241,35.6787458960329,7.36952370122193));
#61206=CARTESIAN_POINT('Ctrl Pts',(-16.8458244073198,35.6864287648063,7.29629339669386));
#61207=CARTESIAN_POINT('Ctrl Pts',(-16.8697415813981,35.6911972380777,7.25127494863602));
#61208=CARTESIAN_POINT('Ctrl Pts',(-16.9348281978171,35.7028902799841,7.14475794261385));
#61209=CARTESIAN_POINT('Ctrl Pts',(-16.9787807774362,35.7098009532432,7.08519551597135));
#61210=CARTESIAN_POINT('Ctrl Pts',(-17.0447073304089,35.7193791961335,7.01046999822976));
#61211=CARTESIAN_POINT('Ctrl Pts',(-17.0623404177004,35.7218760406653,6.99166926813579));
#61212=CARTESIAN_POINT('Ctrl Pts',(-17.0934023613919,35.7261808299377,6.96050728330895));
#61213=CARTESIAN_POINT('Ctrl Pts',(-17.1065486499346,35.7279761013246,6.94787472257021));
#61214=CARTESIAN_POINT('Ctrl Pts',(-17.1344024598995,35.7317302204077,6.92223948785534));
#61215=CARTESIAN_POINT('Ctrl Pts',(-17.1491485408131,35.7336905462279,6.90928623935327));
#61216=CARTESIAN_POINT('Ctrl Pts',(-17.1905335461279,35.7391245130915,6.87459834739053));
#61217=CARTESIAN_POINT('Ctrl Pts',(-17.2177616433662,35.742626027706,6.85359759321332));
#61218=CARTESIAN_POINT('Ctrl Pts',(-17.2841857517224,35.7510107725956,6.80653627524804));
#61219=CARTESIAN_POINT('Ctrl Pts',(-17.3240432455883,35.7559221728098,6.78149998640374));
#61220=CARTESIAN_POINT('Ctrl Pts',(-17.4394770515388,35.7697938540374,6.71763626619782));
#61221=CARTESIAN_POINT('Ctrl Pts',(-17.517700762349,35.7788098129969,6.68408719351732));
#61222=CARTESIAN_POINT('Ctrl Pts',(-17.613160724782,35.7890799663786,6.65403989419658));
#61223=CARTESIAN_POINT('Ctrl Pts',(-17.6277094375507,35.7906254940437,6.64974532635992));
#61224=CARTESIAN_POINT('Ctrl Pts',(-17.6522876320247,35.7931999554031,6.64296648724193));
#61225=CARTESIAN_POINT('Ctrl Pts',(-17.6622760933924,35.7942360524507,6.64034224483409));
#61226=CARTESIAN_POINT('Ctrl Pts',(-17.6846191907843,35.7965305994794,6.63476257766453));
#61227=CARTESIAN_POINT('Ctrl Pts',(-17.6969880241741,35.7977856207197,6.6318701272081));
#61228=CARTESIAN_POINT('Ctrl Pts',(-17.7382870306109,35.8019324462834,6.62286366361214));
#61229=CARTESIAN_POINT('Ctrl Pts',(-17.7673898961388,35.8047839047061,6.61757371819956));
#61230=CARTESIAN_POINT('Ctrl Pts',(-17.8470543708132,35.8124675966635,6.60595108007677));
#61231=CARTESIAN_POINT('Ctrl Pts',(-17.8978553997377,35.8172366733466,6.60163594318235));
#61232=CARTESIAN_POINT('Ctrl Pts',(-18.0226432308793,35.8289294517286,6.59856762193126));
#61233=CARTESIAN_POINT('Ctrl Pts',(-18.0965122990164,35.8358392745671,6.60320029460235));
#61234=CARTESIAN_POINT('Ctrl Pts',(-18.1950373029715,35.8454166261403,6.61807221981021));
#61235=CARTESIAN_POINT('Ctrl Pts',(-18.2203956408775,35.847913485061,6.62269333116675));
#61236=CARTESIAN_POINT('Ctrl Pts',(-18.2634221350487,35.8522183148961,6.63189488441529));
#61237=CARTESIAN_POINT('Ctrl Pts',(-18.281165026514,35.8540136126846,6.63609079573032));
#61238=CARTESIAN_POINT('Ctrl Pts',(-18.317808554755,35.8577678059678,6.64559378189925));
#61239=CARTESIAN_POINT('Ctrl Pts',(-18.3366885688891,35.8597281798652,6.65096006614578));
#61240=CARTESIAN_POINT('Ctrl Pts',(-18.3882768002448,35.8651623590966,6.66692398557671));
#61241=CARTESIAN_POINT('Ctrl Pts',(-18.4206878282985,35.8686640406985,6.67841470592225));
#61242=CARTESIAN_POINT('Ctrl Pts',(-18.4962523687805,35.8770493167417,6.70870917533902));
#61243=CARTESIAN_POINT('Ctrl Pts',(-18.5389038394608,35.8819610858919,6.72862435320042));
#61244=CARTESIAN_POINT('Ctrl Pts',(-18.6551505210169,35.8958321242142,6.79098314601182));
#61245=CARTESIAN_POINT('Ctrl Pts',(-18.7257473666319,35.9048470247851,6.83851127054129));
#61246=CARTESIAN_POINT('Ctrl Pts',(-18.8027503731567,35.9151163154596,6.90241956968076));
#61247=CARTESIAN_POINT('Ctrl Pts',(-18.8142486176276,35.9166619557591,6.91231561261081));
#61248=CARTESIAN_POINT('Ctrl Pts',(-18.8332728057225,35.9192365503464,6.92929167066815));
#61249=CARTESIAN_POINT('Ctrl Pts',(-18.8408941347874,35.9202726695755,6.93626129529115));
#61250=CARTESIAN_POINT('Ctrl Pts',(-18.8576976349681,35.9225671958382,6.95200862618872));
#61251=CARTESIAN_POINT('Ctrl Pts',(-18.8668346050775,35.9238221751267,6.96083239585717));
#61252=CARTESIAN_POINT('Ctrl Pts',(-18.8967938895666,35.9279686598064,6.99064627004785));
#61253=CARTESIAN_POINT('Ctrl Pts',(-18.9170175954944,35.9308198283914,7.01222818276626));
#61254=CARTESIAN_POINT('Ctrl Pts',(-18.9699733069114,35.9385023302184,7.07285127875576));
#61255=CARTESIAN_POINT('Ctrl Pts',(-19.0011406911917,35.9432705304673,7.1131870611411));
#61256=CARTESIAN_POINT('Ctrl Pts',(-19.0713902291101,35.9549636675338,7.21637312914291));
#61257=CARTESIAN_POINT('Ctrl Pts',(-19.1075608186877,35.9618747021449,7.28096248809144));
#61258=CARTESIAN_POINT('Ctrl Pts',(-19.1484957617063,35.971453340069,7.37182145462762));
#61259=CARTESIAN_POINT('Ctrl Pts',(-19.1583635555908,35.9739501980182,7.39563376928951));
#61260=CARTESIAN_POINT('Ctrl Pts',(-19.1739632914659,35.9782550179995,7.43677483999959));
#61261=CARTESIAN_POINT('Ctrl Pts',(-19.1800588512636,35.9800503067591,7.45395787733186));
#61262=CARTESIAN_POINT('Ctrl Pts',(-19.1919441142103,35.9838044719827,7.48989914072911));
#61263=CARTESIAN_POINT('Ctrl Pts',(-19.1976728906673,35.9857648267163,7.50867214411029));
#61264=CARTESIAN_POINT('Ctrl Pts',(-19.2084990379349,35.9898052828975,7.54733683714307));
#61265=CARTESIAN_POINT('Ctrl Pts',(-19.2135535197071,35.9918861425367,7.56723442577343));
#61266=CARTESIAN_POINT('Ctrl Pts',(-19.2393872838271,36.0037323841713,7.680354649335));
#61267=CARTESIAN_POINT('Ctrl Pts',(-19.2500751712369,36.0137975274248,7.77554533972636));
#61268=CARTESIAN_POINT('Ctrl Pts',(-19.249999602058,36.0238536116147,7.87100537183017));
#61269=CARTESIAN_POINT('Ctrl Pts',(-19.2499996010994,36.0238537391044,7.87100658206029));
#61270=CARTESIAN_POINT('Ctrl Pts',(-19.2499608072807,36.0290098734858,7.91995255092519));
#61271=CARTESIAN_POINT('Ctrl Pts',(-19.2470924523388,36.0341450524481,7.96886265353495));
#61272=CARTESIAN_POINT('Ctrl Pts',(-19.2400018586021,36.0404184819091,8.02950420490857));
#61273=CARTESIAN_POINT('Ctrl Pts',(-19.2384256559987,36.041654431005,8.04149688136434));
#61274=CARTESIAN_POINT('Ctrl Pts',(-19.2353003526182,36.0438503076806,8.06290412787031));
#61275=CARTESIAN_POINT('Ctrl Pts',(-19.2338160821336,36.044813277187,8.07232704043072));
#61276=CARTESIAN_POINT('Ctrl Pts',(-19.2304817502714,36.0468198382188,8.09204686891696));
#61277=CARTESIAN_POINT('Ctrl Pts',(-19.2286105127149,36.0478618398658,8.10233859804876));
#61278=CARTESIAN_POINT('Ctrl Pts',(-19.2233848830273,36.0505693722261,8.12918996442249));
#61279=CARTESIAN_POINT('Ctrl Pts',(-19.2198267922409,36.052224025085,8.14570823927836));
#61280=CARTESIAN_POINT('Ctrl Pts',(-19.2016843495377,36.059883368015,8.22245925370173));
#61281=CARTESIAN_POINT('Ctrl Pts',(-19.1830315643831,36.0657090962037,8.28165247600621));
#61282=CARTESIAN_POINT('Ctrl Pts',(-19.1363887348613,36.0775431016332,8.39895421121359));
#61283=CARTESIAN_POINT('Ctrl Pts',(-19.1081565416069,36.0835343947072,8.45676183324533));
#61284=CARTESIAN_POINT('Ctrl Pts',(-19.057635922448,36.0930337232955,8.54295863544918));
#61285=CARTESIAN_POINT('Ctrl Pts',(-19.0383114149812,36.0964556001011,8.57295728453371));
#61286=CARTESIAN_POINT('Ctrl Pts',(-19.0063172954067,36.1018514283087,8.61830895193234));
#61287=CARTESIAN_POINT('Ctrl Pts',(-18.9945051729102,36.1037930576693,8.63424644238579));
#61288=CARTESIAN_POINT('Ctrl Pts',(-18.9711775239964,36.1075399483639,8.66422708704646));
#61289=CARTESIAN_POINT('Ctrl Pts',(-18.9597244168299,36.1093423737212,8.67831276719533));
#61290=CARTESIAN_POINT('Ctrl Pts',(-18.9316618286343,36.1136766319416,8.71135290560143));
#61291=CARTESIAN_POINT('Ctrl Pts',(-18.9147831451959,36.1162190718351,8.73006696652725));
#61292=CARTESIAN_POINT('Ctrl Pts',(-18.8696590608875,36.1228626166517,8.7771997277421));
#61293=CARTESIAN_POINT('Ctrl Pts',(-18.8406242357173,36.1269929008927,8.8047865100712));
#61294=CARTESIAN_POINT('Ctrl Pts',(-18.8103594475449,36.1311618021068,8.83093870141285));
#61295=CARTESIAN_POINT('Ctrl Pts',(-18.8103597855904,36.3002088453023,8.83093840930324));
#61296=CARTESIAN_POINT('Ctrl Pts',(-18.8164268746474,36.2993964359777,8.82569575616366));
#61297=CARTESIAN_POINT('Ctrl Pts',(-18.822444535654,36.298587756557,8.82039545161663));
#61298=CARTESIAN_POINT('Ctrl Pts',(-18.83620292553,36.2967328724837,8.80804380032832));
#61299=CARTESIAN_POINT('Ctrl Pts',(-18.8439068972887,36.295690000473,8.80095354923604));
#61300=CARTESIAN_POINT('Ctrl Pts',(-18.8638623439902,36.2929748083373,8.78212670967425));
#61301=CARTESIAN_POINT('Ctrl Pts',(-18.8759681958865,36.2913134927087,8.77023823162753));
#61302=CARTESIAN_POINT('Ctrl Pts',(-18.929109337216,36.283934304214,8.71591690495378));
#61303=CARTESIAN_POINT('Ctrl Pts',(-18.9674006316583,36.2783769485685,8.67089086844673));
#61304=CARTESIAN_POINT('Ctrl Pts',(-19.0383431120129,36.2671604116637,8.57461064378817));
#61305=CARTESIAN_POINT('Ctrl Pts',(-19.0707272129343,36.2615158872613,8.52336048350766));
#61306=CARTESIAN_POINT('Ctrl Pts',(-19.1181189855404,36.2520090259425,8.4349483288327));
#61307=CARTESIAN_POINT('Ctrl Pts',(-19.1352478205279,36.2482064136738,8.39903992315327));
#61308=CARTESIAN_POINT('Ctrl Pts',(-19.1585969639633,36.2423613587935,8.34352717998947));
#61309=CARTESIAN_POINT('Ctrl Pts',(-19.1660735342583,36.2403613467927,8.32447579442566));
#61310=CARTESIAN_POINT('Ctrl Pts',(-19.1792522966141,36.2365734494003,8.288351095454));
#61311=CARTESIAN_POINT('Ctrl Pts',(-19.1850581854163,36.2347895534342,8.27132081305205));
#61312=CARTESIAN_POINT('Ctrl Pts',(-19.1975830718585,36.2306556863584,8.23185595201631));
#61313=CARTESIAN_POINT('Ctrl Pts',(-19.2040469118179,36.2282980054184,8.20934825354585));
#61314=CARTESIAN_POINT('Ctrl Pts',(-19.2366090703395,36.215036324851,8.08288583400888));
#61315=CARTESIAN_POINT('Ctrl Pts',(-19.2500815441936,36.203733902395,7.97615196007877));
#61316=CARTESIAN_POINT('Ctrl Pts',(-19.2499635734042,36.1874934391101,7.82187826498927));
#61317=CARTESIAN_POINT('Ctrl Pts',(-19.2473017254069,36.1825553388251,7.77475981211089));
#61318=CARTESIAN_POINT('Ctrl Pts',(-19.2403638736094,36.1761966483956,7.71314614950596));
#61319=CARTESIAN_POINT('Ctrl Pts',(-19.2384448668738,36.1746853386944,7.69842840176448));
#61320=CARTESIAN_POINT('Ctrl Pts',(-19.23475855701,36.172148419923,7.67356447320316));
#61321=CARTESIAN_POINT('Ctrl Pts',(-19.2331251927494,36.1711161823326,7.6634007742838));
#61322=CARTESIAN_POINT('Ctrl Pts',(-19.2291658921259,36.1688057287158,7.6405417357144));
#61323=CARTESIAN_POINT('Ctrl Pts',(-19.2267697600024,36.1675313161604,7.62786008781158));
#61324=CARTESIAN_POINT('Ctrl Pts',(-19.2179438796925,36.1632180532542,7.58476084343394));
#61325=CARTESIAN_POINT('Ctrl Pts',(-19.2105902430604,36.1602241808432,7.55454067269639));
#61326=CARTESIAN_POINT('Ctrl Pts',(-19.186925812673,36.1519315152939,7.47080433941823));
#61327=CARTESIAN_POINT('Ctrl Pts',(-19.1681791134797,36.1467087713969,7.41805032324011));
#61328=CARTESIAN_POINT('Ctrl Pts',(-19.1193460620872,36.1351649166607,7.30491689039958));
#61329=CARTESIAN_POINT('Ctrl Pts',(-19.0878131164039,36.1288521283137,7.24535881711062));
#61330=CARTESIAN_POINT('Ctrl Pts',(-19.0380002451793,36.1199258353162,7.16701436413346));
#61331=CARTESIAN_POINT('Ctrl Pts',(-19.0236391327178,36.1174488551599,7.14586570978843));
#61332=CARTESIAN_POINT('Ctrl Pts',(-18.9979776289267,36.1131671268238,7.11042594435977));
#61333=CARTESIAN_POINT('Ctrl Pts',(-18.9869894115542,36.1113746988024,7.09591768001499));
#61334=CARTESIAN_POINT('Ctrl Pts',(-18.9634689139916,36.107616390796,7.06621100168647));
#61335=CARTESIAN_POINT('Ctrl Pts',(-18.9508872715427,36.1056488911378,7.05105821188776));
#61336=CARTESIAN_POINT('Ctrl Pts',(-18.9151062214748,36.1001633652424,7.00994883224409));
#61337=CARTESIAN_POINT('Ctrl Pts',(-18.891186297287,36.0966165171022,6.98464662372967));
#61338=CARTESIAN_POINT('Ctrl Pts',(-18.8318728322982,36.0880833013343,6.92685754241105));
#61339=CARTESIAN_POINT('Ctrl Pts',(-18.7956172279711,36.0830671822959,6.89533467703813));
#61340=CARTESIAN_POINT('Ctrl Pts',(-18.69231568615,36.069322501654,6.81532489133015));
#61341=CARTESIAN_POINT('Ctrl Pts',(-18.6221714168987,36.0605488861438,6.77120448919014));
#61342=CARTESIAN_POINT('Ctrl Pts',(-18.5344484750624,36.0504779286096,6.72731702848951));
#61343=CARTESIAN_POINT('Ctrl Pts',(-18.5205409689291,36.0489068764641,6.72067279454311));
#61344=CARTESIAN_POINT('Ctrl Pts',(-18.4970946746568,36.0463043885496,6.70999126977089));
#61345=CARTESIAN_POINT('Ctrl Pts',(-18.4876218807714,36.0452653873125,6.70581478180152));
#61346=CARTESIAN_POINT('Ctrl Pts',(-18.4665503301956,36.042982278355,6.6968306336465));
#61347=CARTESIAN_POINT('Ctrl Pts',(-18.4549295716298,36.041741329982,6.69207829850181));
#61348=CARTESIAN_POINT('Ctrl Pts',(-18.4166700514419,36.0377083413326,6.67709030895712));
#61349=CARTESIAN_POINT('Ctrl Pts',(-18.3897540981057,36.0349536417919,6.66757900410528));
#61350=CARTESIAN_POINT('Ctrl Pts',(-18.3169525702975,36.027659387109,6.64458241206052));
#61351=CARTESIAN_POINT('Ctrl Pts',(-18.2705870755116,36.0231753831898,6.63276709074159));
#61352=CARTESIAN_POINT('Ctrl Pts',(-18.1464765668155,36.0113264641109,6.60850453180685));
#61353=CARTESIAN_POINT('Ctrl Pts',(-18.0680663209311,36.0039861333247,6.60061933193078));
#61354=CARTESIAN_POINT('Ctrl Pts',(-17.9637535984537,35.9939582351488,6.59984421703849));
#61355=CARTESIAN_POINT('Ctrl Pts',(-17.9380728503237,35.9914696700677,6.60043253173901));
#61356=CARTESIAN_POINT('Ctrl Pts',(-17.8942394906364,35.9871746699727,6.60276799484169));
#61357=CARTESIAN_POINT('Ctrl Pts',(-17.8760735574333,35.9853807628617,6.60412835236113));
#61358=CARTESIAN_POINT('Ctrl Pts',(-17.8383847868328,35.9816254872065,6.60776734598386));
#61359=CARTESIAN_POINT('Ctrl Pts',(-17.8188732099629,35.9796625848725,6.61010945415574));
#61360=CARTESIAN_POINT('Ctrl Pts',(-17.7652353021889,35.9742091622604,6.61781423415897));
#61361=CARTESIAN_POINT('Ctrl Pts',(-17.7312644369128,35.97069040714,6.62411753660487));
#61362=CARTESIAN_POINT('Ctrl Pts',(-17.6513758523523,35.962249225731,6.64233813743481));
#61363=CARTESIAN_POINT('Ctrl Pts',(-17.6057873463636,35.957298031662,6.65545838547015));
#61364=CARTESIAN_POINT('Ctrl Pts',(-17.4817090961854,35.9434753734014,6.69881735860065));
#61365=CARTESIAN_POINT('Ctrl Pts',(-17.4053158317851,35.9345523988724,6.7343489850474));
#61366=CARTESIAN_POINT('Ctrl Pts',(-17.3198558260985,35.9243585501369,6.78494582764722));
#61367=CARTESIAN_POINT('Ctrl Pts',(-17.3068642069141,35.9228031947767,6.79295721126881));
#61368=CARTESIAN_POINT('Ctrl Pts',(-17.285321667145,35.9202180860495,6.80678373750636));
#61369=CARTESIAN_POINT('Ctrl Pts',(-17.2766922227958,35.9191810129989,6.81247221497463));
#61370=CARTESIAN_POINT('Ctrl Pts',(-17.2576649619155,35.9168914696714,6.82535085005714));
#61371=CARTESIAN_POINT('Ctrl Pts',(-17.2473033964975,35.9156423184911,6.83259193723455));
#61372=CARTESIAN_POINT('Ctrl Pts',(-17.2134185257701,35.9115427840077,6.85703311962151));
#61373=CARTESIAN_POINT('Ctrl Pts',(-17.1903767653524,35.9087314870191,6.8748896369118));
#61374=CARTESIAN_POINT('Ctrl Pts',(-17.1298202301443,35.9012114130481,6.9252482458142));
#61375=CARTESIAN_POINT('Ctrl Pts',(-17.0935616311797,35.8965625404014,6.95918201285587));
#61376=CARTESIAN_POINT('Ctrl Pts',(-17.0071557819574,35.8848118837662,7.05010884769546));
#61377=CARTESIAN_POINT('Ctrl Pts',(-16.9599647513936,35.8777277220064,7.10962294529209));
#61378=CARTESIAN_POINT('Ctrl Pts',(-16.9042250413927,35.8679657750806,7.19452090244234));
#61379=CARTESIAN_POINT('Ctrl Pts',(-16.8907449286172,35.865469717203,7.21648110642693));
#61380=CARTESIAN_POINT('Ctrl Pts',(-16.8688844325569,35.861166123642,7.25465097661411));
#61381=CARTESIAN_POINT('Ctrl Pts',(-16.8601681089293,35.8593712506906,7.27065980086283));
#61382=CARTESIAN_POINT('Ctrl Pts',(-16.8427895410929,35.8556178684879,7.30428149450014));
#61383=CARTESIAN_POINT('Ctrl Pts',(-16.8341851579288,35.853657880225,7.32191853526637));
#61384=CARTESIAN_POINT('Ctrl Pts',(-16.8116424244363,35.8482247272423,7.370978970431));
#61385=CARTESIAN_POINT('Ctrl Pts',(-16.7985671545369,35.8447236954916,7.40277705829569));
#61386=CARTESIAN_POINT('Ctrl Pts',(-16.7706921627854,35.8363402297381,7.47924890907114));
#61387=CARTESIAN_POINT('Ctrl Pts',(-16.7570544639594,35.8314296349592,7.52429050096402));
#61388=CARTESIAN_POINT('Ctrl Pts',(-16.725887094001,35.8175569260029,7.65248894201771));
#61389=CARTESIAN_POINT('Ctrl Pts',(-16.7141513430886,35.8085390473888,7.73680857212909));
#61390=CARTESIAN_POINT('Ctrl Pts',(-16.7103427577419,35.7982674782518,7.83682750871485));
#61391=CARTESIAN_POINT('Ctrl Pts',(-16.7100371452135,35.7967223108948,7.85199026394879));
#61392=CARTESIAN_POINT('Ctrl Pts',(-16.7099800648641,35.7941484287091,7.87748038396702));
#61393=CARTESIAN_POINT('Ctrl Pts',(-16.7100828340201,35.7931125538241,7.88780509562494));
#61394=CARTESIAN_POINT('Ctrl Pts',(-16.7105927749681,35.7908185660214,7.91082305528718));
#61395=CARTESIAN_POINT('Ctrl Pts',(-16.7110643870074,35.7895638792921,7.92351339288237));
#61396=CARTESIAN_POINT('Ctrl Pts',(-16.7132667046723,35.7854186868468,7.96570875292727));
#61397=CARTESIAN_POINT('Ctrl Pts',(-16.7158370151808,35.782568489306,7.99516309626957));
#61398=CARTESIAN_POINT('Ctrl Pts',(-16.7256250195747,35.7748896784937,8.07502115993411));
#61399=CARTESIAN_POINT('Ctrl Pts',(-16.7348483212888,35.7701241291193,8.12512441530049));
#61400=CARTESIAN_POINT('Ctrl Pts',(-16.764785644149,35.7584295870054,8.24632604656152));
#61401=CARTESIAN_POINT('Ctrl Pts',(-16.7887489485983,35.7515145704087,8.31641463520439));
#61402=CARTESIAN_POINT('Ctrl Pts',(-16.8290996474445,35.7419319202978,8.40758019795731));
#61403=CARTESIAN_POINT('Ctrl Pts',(-16.8402435992797,35.7394352841977,8.43082013124674));
#61404=CARTESIAN_POINT('Ctrl Pts',(-16.8604634632196,35.7351310255058,8.46989182320388));
#61405=CARTESIAN_POINT('Ctrl Pts',(-16.8691881569258,35.7333360760363,8.48589708537482));
#61406=CARTESIAN_POINT('Ctrl Pts',(-16.8880132002418,35.7295828326834,8.5187293755671));
#61407=CARTESIAN_POINT('Ctrl Pts',(-16.8981651185921,35.7276230639687,8.53552096282337));
#61408=CARTESIAN_POINT('Ctrl Pts',(-16.927154037602,35.7221914437242,8.58105267893841));
#61409=CARTESIAN_POINT('Ctrl Pts',(-16.9467730912697,35.7186917529854,8.60927134511065));
#61410=CARTESIAN_POINT('Ctrl Pts',(-16.9958829819392,35.7103126427103,8.67412864765872));
#61411=CARTESIAN_POINT('Ctrl Pts',(-17.0263113784383,35.7054051079809,8.70999177571336));
#61412=CARTESIAN_POINT('Ctrl Pts',(-17.1171405413213,35.6915286050961,8.80573234895545));
#61413=CARTESIAN_POINT('Ctrl Pts',(-17.1816721347875,35.6825035459852,8.86136100023632));
#61414=CARTESIAN_POINT('Ctrl Pts',(-17.2636950793387,35.6722261089264,8.91882646908317));
#61415=CARTESIAN_POINT('Ctrl Pts',(-17.2762634913481,35.6706817201561,8.92730066870284));
#61416=CARTESIAN_POINT('Ctrl Pts',(-17.2976432801477,35.6681086889838,8.94116566584799));
#61417=CARTESIAN_POINT('Ctrl Pts',(-17.3063735263717,35.6670728988364,8.94667729097374));
#61418=CARTESIAN_POINT('Ctrl Pts',(-17.3259938012349,35.6647785381793,8.95873193959987));
#61419=CARTESIAN_POINT('Ctrl Pts',(-17.3369164084793,35.6635234023712,8.9652191045742));
#61420=CARTESIAN_POINT('Ctrl Pts',(-17.3735977247526,35.6593745232478,8.98626684396428));
#61421=CARTESIAN_POINT('Ctrl Pts',(-17.3997701741929,35.6565211869616,9.00009255500328));
#61422=CARTESIAN_POINT('Ctrl Pts',(-17.472304236726,35.6488294347508,9.03522356350001));
#61423=CARTESIAN_POINT('Ctrl Pts',(-17.5195049131126,35.6440543430188,9.054671313635));
#61424=CARTESIAN_POINT('Ctrl Pts',(-17.6375461686839,35.632364055603,9.09518181083352));
#61425=CARTESIAN_POINT('Ctrl Pts',(-17.7092870250348,35.6254625802331,9.11300340188724));
#61426=CARTESIAN_POINT('Ctrl Pts',(-17.8076171125583,35.6158944157863,9.12851029873159));
#61427=CARTESIAN_POINT('Ctrl Pts',(-17.8331853995243,35.6133978857198,9.13174850380631));
#61428=CARTESIAN_POINT('Ctrl Pts',(-17.876977140758,35.609093740034,9.13594571153269));
#61429=CARTESIAN_POINT('Ctrl Pts',(-17.8951559364666,35.6072987954106,9.13729383045634));
#61430=CARTESIAN_POINT('Ctrl Pts',(-17.932950590581,35.6035454968264,9.13927985469515));
#61431=CARTESIAN_POINT('Ctrl Pts',(-17.9525646351676,35.6015856671171,9.13985518317132));
#61432=CARTESIAN_POINT('Ctrl Pts',(-18.0065440733122,35.596153669798,9.14018744941228));
#61433=CARTESIAN_POINT('Ctrl Pts',(-18.0408953839286,35.592653656559,9.13900430669479));
#61434=CARTESIAN_POINT('Ctrl Pts',(-18.1220291241248,35.584273512291,9.1329083680634));
#61435=CARTESIAN_POINT('Ctrl Pts',(-18.168668276846,35.579365255559,9.12678680855988));
#61436=CARTESIAN_POINT('Ctrl Pts',(-18.2983541043188,35.5654896172384,9.10238368134162));
#61437=CARTESIAN_POINT('Ctrl Pts',(-18.3800714473173,35.5564662210263,9.07833118362491));
#61438=CARTESIAN_POINT('Ctrl Pts',(-18.4728195645737,35.5461901391829,9.04058046776377));
#61439=CARTESIAN_POINT('Ctrl Pts',(-18.4867565930735,35.5446455670261,9.0346147801621));
#61440=CARTESIAN_POINT('Ctrl Pts',(-18.5100011279264,35.5420723404975,9.02416869811904));
#61441=CARTESIAN_POINT('Ctrl Pts',(-18.5193661869721,35.5410365353539,9.01982204437786));
#61442=CARTESIAN_POINT('Ctrl Pts',(-18.5401327217626,35.5387422913517,9.00987395976245));
#61443=CARTESIAN_POINT('Ctrl Pts',(-18.5515049490686,35.5374872849198,9.00421490542589));
#61444=CARTESIAN_POINT('Ctrl Pts',(-18.5890711574812,35.5333393875388,8.98481262596709));
#61445=CARTESIAN_POINT('Ctrl Pts',(-18.6148723179907,35.5304868784653,8.97032379447077));
#61446=CARTESIAN_POINT('Ctrl Pts',(-18.6836917195907,35.5227985276337,8.92844985984082));
#61447=CARTESIAN_POINT('Ctrl Pts',(-18.7256057145195,35.5180259431793,8.89935473245868));
#61448=CARTESIAN_POINT('Ctrl Pts',(-18.7808448467063,35.5114400758792,8.85586055815525));
#61449=CARTESIAN_POINT('Ctrl Pts',(-18.795748290919,35.5096311151527,8.84356440024732));
#61450=CARTESIAN_POINT('Ctrl Pts',(-18.8103598667433,35.5078191442546,8.83093833917793));
#61451=CARTESIAN_POINT('Origin',(-17.98,42.93984859951,7.87));
#61452=CARTESIAN_POINT('',(-18.8103597424409,34.5453270911211,8.83093844658932));
#61453=CARTESIAN_POINT('',(-18.810359785549,34.7139132859163,8.83093840933901));
#61454=CARTESIAN_POINT('',(-18.810359785549,42.93984859951,8.83093840933902));
#61455=CARTESIAN_POINT('Ctrl Pts',(-18.8103597424409,34.5453270911211,8.83093844658933));
#61456=CARTESIAN_POINT('Ctrl Pts',(-18.7582784971811,34.5519273472422,8.87594254602299));
#61457=CARTESIAN_POINT('Ctrl Pts',(-18.7025978955493,34.5583389621438,8.91666128726311));
#61458=CARTESIAN_POINT('Ctrl Pts',(-18.6044300911063,34.5691275162025,8.9768541522636));
#61459=CARTESIAN_POINT('Ctrl Pts',(-18.563713770624,34.573469711912,8.99885637855351));
#61460=CARTESIAN_POINT('Ctrl Pts',(-18.4911605351903,34.5811062412763,9.03308617899149));
#61461=CARTESIAN_POINT('Ctrl Pts',(-18.4598640189898,34.5843694085406,9.04634375194037));
#61462=CARTESIAN_POINT('Ctrl Pts',(-18.4098461168205,34.5895694162822,9.06520371504832));
#61463=CARTESIAN_POINT('Ctrl Pts',(-18.3914611272229,34.5914775361062,9.07165687377777));
#61464=CARTESIAN_POINT('Ctrl Pts',(-18.355699923058,34.5951885374251,9.08329225970602));
#61465=CARTESIAN_POINT('Ctrl Pts',(-18.3383467571686,34.5969890583393,9.08853028430628));
#61466=CARTESIAN_POINT('Ctrl Pts',(-18.2961909528124,34.6013667488425,9.10027664080755));
#61467=CARTESIAN_POINT('Ctrl Pts',(-18.2712930498596,34.6039554378379,9.1064082839928));
#61468=CARTESIAN_POINT('Ctrl Pts',(-18.1685704784758,34.6146612288439,9.12843125013388));
#61469=CARTESIAN_POINT('Ctrl Pts',(-18.0895377763885,34.6229731015943,9.13775564639213));
#61470=CARTESIAN_POINT('Ctrl Pts',(-17.9624772255803,34.6363774925223,9.14077487216361));
#61471=CARTESIAN_POINT('Ctrl Pts',(-17.9147568068693,34.6414168289293,9.13922007761438));
#61472=CARTESIAN_POINT('Ctrl Pts',(-17.8388559332839,34.6493687218697,9.13245400583687));
#61473=CARTESIAN_POINT('Ctrl Pts',(-17.8105666896419,34.6523178104545,9.12896961935409));
#61474=CARTESIAN_POINT('Ctrl Pts',(-17.770066662084,34.6564999099261,9.12259102232216));
#61475=CARTESIAN_POINT('Ctrl Pts',(-17.7577463207581,34.6577667321182,9.1204637635419));
#61476=CARTESIAN_POINT('Ctrl Pts',(-17.7353154079887,34.660061063118,9.11624875756492));
#61477=CARTESIAN_POINT('Ctrl Pts',(-17.7251963607594,34.6610912911448,9.11421928858266));
#61478=CARTESIAN_POINT('Ctrl Pts',(-17.7001212278364,34.6636341012551,9.10887146293338));
#61479=CARTESIAN_POINT('Ctrl Pts',(-17.6851982998348,34.6651386474236,9.10540546612928));
#61480=CARTESIAN_POINT('Ctrl Pts',(-17.5892586478978,34.674777785137,9.081284861242));
#61481=CARTESIAN_POINT('Ctrl Pts',(-17.5103717906956,34.6825561351185,9.05293894812749));
#61482=CARTESIAN_POINT('Ctrl Pts',(-17.3917946895006,34.6948573568254,8.99658118356185));
#61483=CARTESIAN_POINT('Ctrl Pts',(-17.3499455762797,34.6993288234307,8.97372165576177));
#61484=CARTESIAN_POINT('Ctrl Pts',(-17.2800366682171,34.7071624624334,8.93026103435852));
#61485=CARTESIAN_POINT('Ctrl Pts',(-17.2513563524533,34.7104912566938,8.91075937964797));
#61486=CARTESIAN_POINT('Ctrl Pts',(-17.2076887698448,34.7157791761104,8.87837663626398));
#61487=CARTESIAN_POINT('Ctrl Pts',(-17.1921415677685,34.7177083223952,8.86627659903483));
#61488=CARTESIAN_POINT('Ctrl Pts',(-17.1627424760259,34.7214531395402,8.84227740064588));
#61489=CARTESIAN_POINT('Ctrl Pts',(-17.1488533809411,34.723266310387,8.83043136831113));
#61490=CARTESIAN_POINT('Ctrl Pts',(-17.1160070178157,34.7276665580663,8.80117054063338));
#61491=CARTESIAN_POINT('Ctrl Pts',(-17.0973155360445,34.7302650629381,8.78347158662414));
#61492=CARTESIAN_POINT('Ctrl Pts',(-17.0254233369961,34.7406567513275,8.71112926161933));
#61493=CARTESIAN_POINT('Ctrl Pts',(-16.9766622122373,34.7486249179249,8.65231948592174));
#61494=CARTESIAN_POINT('Ctrl Pts',(-16.9056933617137,34.7618219789575,8.54909514508476));
#61495=CARTESIAN_POINT('Ctrl Pts',(-16.8802727595058,34.7670001873093,8.50710705356034));
#61496=CARTESIAN_POINT('Ctrl Pts',(-16.8438101129522,34.775136787827,8.43816409611634));
#61497=CARTESIAN_POINT('Ctrl Pts',(-16.8311541505679,34.7781326271269,8.41211761480097));
#61498=CARTESIAN_POINT('Ctrl Pts',(-16.8142684713525,34.7823741707503,8.37411270525194));
#61499=CARTESIAN_POINT('Ctrl Pts',(-16.8093108953179,34.7836543310606,8.36249028807224));
#61500=CARTESIAN_POINT('Ctrl Pts',(-16.8006015595804,34.7859667131828,8.34119724755845));
#61501=CARTESIAN_POINT('Ctrl Pts',(-16.7967937163622,34.787001760402,8.33155220348613));
#61502=CARTESIAN_POINT('Ctrl Pts',(-16.7876269695703,34.7895567082208,8.30747402249677));
#61503=CARTESIAN_POINT('Ctrl Pts',(-16.7824115344412,34.7910685242448,8.29298807496062));
#61504=CARTESIAN_POINT('Ctrl Pts',(-16.7508127296122,34.8006414901204,8.19994714233014));
#61505=CARTESIAN_POINT('Ctrl Pts',(-16.7319030157318,34.8083541747029,8.11904946444439));
#61506=CARTESIAN_POINT('Ctrl Pts',(-16.7147190815839,34.8206084640349,7.98940313888672));
#61507=CARTESIAN_POINT('Ctrl Pts',(-16.7111174353948,34.8251014430528,7.94161960789952));
#61508=CARTESIAN_POINT('Ctrl Pts',(-16.7095721672306,34.8329647416264,7.85900178640592));
#61509=CARTESIAN_POINT('Ctrl Pts',(-16.7103489075829,34.8363012606013,7.82424560786309));
#61510=CARTESIAN_POINT('Ctrl Pts',(-16.7137967816126,34.841596540539,7.7699137009731));
#61511=CARTESIAN_POINT('Ctrl Pts',(-16.715500969673,34.8435251032127,7.75029221378086));
#61512=CARTESIAN_POINT('Ctrl Pts',(-16.7196584425836,34.84726574084,7.71261181284371));
#61513=CARTESIAN_POINT('Ctrl Pts',(-16.7220456171656,34.8490752747315,7.69455039120294));
#61514=CARTESIAN_POINT('Ctrl Pts',(-16.7287229801233,34.8534601084332,7.65122554098748));
#61515=CARTESIAN_POINT('Ctrl Pts',(-16.7333907122903,34.8560466933605,7.62602974709626));
#61516=CARTESIAN_POINT('Ctrl Pts',(-16.7558234819504,34.866836993304,7.52252558737143));
#61517=CARTESIAN_POINT('Ctrl Pts',(-16.780229679866,34.8752391929057,7.44586257015318));
#61518=CARTESIAN_POINT('Ctrl Pts',(-16.8300833161191,34.8886434046107,7.32889929835048));
#61519=CARTESIAN_POINT('Ctrl Pts',(-16.8508429649672,34.8935927622566,7.28681633197213));
#61520=CARTESIAN_POINT('Ctrl Pts',(-16.8877523411963,34.9014272139768,7.22139245582048));
#61521=CARTESIAN_POINT('Ctrl Pts',(-16.9024386638579,34.9043474033965,7.1972752165736));
#61522=CARTESIAN_POINT('Ctrl Pts',(-16.9247780382346,34.9085022707195,7.16320219648806));
#61523=CARTESIAN_POINT('Ctrl Pts',(-16.9317924709225,34.9097697903486,7.15284064129368));
#61524=CARTESIAN_POINT('Ctrl Pts',(-16.9448929367575,34.9120685326634,7.13409193200277));
#61525=CARTESIAN_POINT('Ctrl Pts',(-16.950929882046,34.9131024179989,7.12567344040614));
#61526=CARTESIAN_POINT('Ctrl Pts',(-16.9662462111649,34.9156649159831,7.10485753645008));
#61527=CARTESIAN_POINT('Ctrl Pts',(-16.9756505664244,34.9171852417243,7.09255416205871));
#61528=CARTESIAN_POINT('Ctrl Pts',(-17.0362275249785,34.9266755801127,7.01623817326308));
#61529=CARTESIAN_POINT('Ctrl Pts',(-17.0932797509064,34.9343054734622,6.95712100496252));
#61530=CARTESIAN_POINT('Ctrl Pts',(-17.192401465746,34.9465127958986,6.87254145042423));
#61531=CARTESIAN_POINT('Ctrl Pts',(-17.2309175522031,34.9510451173478,6.84330145160162));
#61532=CARTESIAN_POINT('Ctrl Pts',(-17.2999942708169,34.958965891441,6.7968209763161));
#61533=CARTESIAN_POINT('Ctrl Pts',(-17.3297747032316,34.9623197173172,6.7785204597929));
#61534=CARTESIAN_POINT('Ctrl Pts',(-17.3774719532837,34.9676339506004,6.75185492942376));
#61535=CARTESIAN_POINT('Ctrl Pts',(-17.3948954246397,34.9695636781307,6.74263981984578));
#61536=CARTESIAN_POINT('Ctrl Pts',(-17.4287882394581,34.9733014371869,6.72571154580774));
#61537=CARTESIAN_POINT('Ctrl Pts',(-17.4452227994205,34.9751068530225,6.7179393552003));
#61538=CARTESIAN_POINT('Ctrl Pts',(-17.485071867192,34.9794721250435,6.70013038357828));
#61539=CARTESIAN_POINT('Ctrl Pts',(-17.5086314127971,34.9820430575475,6.69044067927907));
#61540=CARTESIAN_POINT('Ctrl Pts',(-17.6094686881542,34.9930185163473,6.65247095108091));
#61541=CARTESIAN_POINT('Ctrl Pts',(-17.6890925513004,35.0016339805726,6.63103361726451));
#61542=CARTESIAN_POINT('Ctrl Pts',(-17.8153177617025,35.0151280362244,6.60989229414256));
#61543=CARTESIAN_POINT('Ctrl Pts',(-17.8608018147034,35.019954053307,6.60477910414765));
#61544=CARTESIAN_POINT('Ctrl Pts',(-17.934235990077,35.0276233928326,6.60051999286205));
#61545=CARTESIAN_POINT('Ctrl Pts',(-17.9620559272994,35.0305004308103,6.59982197968922));
#61546=CARTESIAN_POINT('Ctrl Pts',(-18.0023232713462,35.0346061401043,6.6001352313657));
#61547=CARTESIAN_POINT('Ctrl Pts',(-18.0147659640791,35.0358666883445,6.60041493694181));
#61548=CARTESIAN_POINT('Ctrl Pts',(-18.0375706508963,35.0381598992813,6.60126312890693));
#61549=CARTESIAN_POINT('Ctrl Pts',(-18.0479323017599,35.0391951057469,6.60177571074422));
#61550=CARTESIAN_POINT('Ctrl Pts',(-18.0738559734803,35.0417700405367,6.60337679294815));
#61551=CARTESIAN_POINT('Ctrl Pts',(-18.0894064426217,35.0433012896209,6.60462511246133));
#61552=CARTESIAN_POINT('Ctrl Pts',(-18.1854685485735,35.0527012443381,6.61412090268889));
#61553=CARTESIAN_POINT('Ctrl Pts',(-18.2650761425341,35.0602400872971,6.62976366321933));
#61554=CARTESIAN_POINT('Ctrl Pts',(-18.3894177446848,35.0723950200306,6.66681382525117));
#61555=CARTESIAN_POINT('Ctrl Pts',(-18.4353252783679,35.0769696586715,6.68342587210011));
#61556=CARTESIAN_POINT('Ctrl Pts',(-18.5124730463806,35.0849532609214,6.71648009005298));
#61557=CARTESIAN_POINT('Ctrl Pts',(-18.544192813886,35.0883267981926,6.73165835359463));
#61558=CARTESIAN_POINT('Ctrl Pts',(-18.5926914165297,35.093665707833,6.7573906596634));
#61559=CARTESIAN_POINT('Ctrl Pts',(-18.6099237814297,35.095599961785,6.76705565007722));
#61560=CARTESIAN_POINT('Ctrl Pts',(-18.6425747631823,35.0993432015768,6.78638313170576));
#61561=CARTESIAN_POINT('Ctrl Pts',(-18.6580250047332,35.1011495162876,6.79598284968859));
#61562=CARTESIAN_POINT('Ctrl Pts',(-18.6945722295729,35.10551174424,6.8197936555465));
#61563=CARTESIAN_POINT('Ctrl Pts',(-18.7154577407295,35.1080786384736,6.83431254224653));
#61564=CARTESIAN_POINT('Ctrl Pts',(-18.7876516225825,35.1172289600729,6.88778429350393));
#61565=CARTESIAN_POINT('Ctrl Pts',(-18.8364102981971,35.1239304278364,6.92999612845889));
#61566=CARTESIAN_POINT('Ctrl Pts',(-18.9310181066678,35.138057438036,7.02539364014778));
#61567=CARTESIAN_POINT('Ctrl Pts',(-18.9760980848497,35.1454731876961,7.07906080627513));
#61568=CARTESIAN_POINT('Ctrl Pts',(-19.0301070089641,35.1551793704443,7.15534805556078));
#61569=CARTESIAN_POINT('Ctrl Pts',(-19.0431509260181,35.1575999794428,7.17490110336863));
#61570=CARTESIAN_POINT('Ctrl Pts',(-19.061898831167,35.161187353366,7.20476827642656));
#61571=CARTESIAN_POINT('Ctrl Pts',(-19.0680134478401,35.1623762189782,7.21481674045736));
#61572=CARTESIAN_POINT('Ctrl Pts',(-19.0793201371124,35.1646091493566,7.23399257344724));
#61573=CARTESIAN_POINT('Ctrl Pts',(-19.0845398081925,35.165654646545,7.24310125223147));
#61574=CARTESIAN_POINT('Ctrl Pts',(-19.0979726723103,35.1683873982777,7.26723127769947));
#61575=CARTESIAN_POINT('Ctrl Pts',(-19.105996381601,35.1700633786177,7.28235615901021));
#61576=CARTESIAN_POINT('Ctrl Pts',(-19.1428132450866,35.1779937768631,7.35528183623477));
#61577=CARTESIAN_POINT('Ctrl Pts',(-19.1674805005846,35.1840542108112,7.41506896214857));
#61578=CARTESIAN_POINT('Ctrl Pts',(-19.2050970514825,35.1954307883825,7.53049402873927));
#61579=CARTESIAN_POINT('Ctrl Pts',(-19.2190544804919,35.2007355109395,7.58562262149037));
#61580=CARTESIAN_POINT('Ctrl Pts',(-19.2361847440921,35.2097678230603,7.67927779760022));
#61581=CARTESIAN_POINT('Ctrl Pts',(-19.2413768717436,35.2134440816518,7.71734731961988));
#61582=CARTESIAN_POINT('Ctrl Pts',(-19.2466615981022,35.2191406475658,7.7757714159675));
#61583=CARTESIAN_POINT('Ctrl Pts',(-19.2480037007771,35.2211220256234,7.79599236003234));
#61584=CARTESIAN_POINT('Ctrl Pts',(-19.2496250406539,35.2248961886384,7.83425648268014));
#61585=CARTESIAN_POINT('Ctrl Pts',(-19.2500045800062,35.2266853465713,7.85229056311728));
#61586=CARTESIAN_POINT('Ctrl Pts',(-19.2499937487628,35.2309070600604,7.89455639469));
#61587=CARTESIAN_POINT('Ctrl Pts',(-19.2492940751784,35.2333486649948,7.91877993259425));
#61588=CARTESIAN_POINT('Ctrl Pts',(-19.2435720632792,35.2434726577152,8.01820835210988));
#61589=CARTESIAN_POINT('Ctrl Pts',(-19.2325539622436,35.2513313838714,8.09289910684355));
#61590=CARTESIAN_POINT('Ctrl Pts',(-19.1976127157057,35.2671125093263,8.23860514393419));
#61591=CARTESIAN_POINT('Ctrl Pts',(-19.1738965453011,35.275002471338,8.30939017136547));
#61592=CARTESIAN_POINT('Ctrl Pts',(-19.1376021076899,35.2843391281057,8.3926109659689));
#61593=CARTESIAN_POINT('Ctrl Pts',(-19.1308094942068,35.2860006878031,8.40740344350387));
#61594=CARTESIAN_POINT('Ctrl Pts',(-19.119228242271,35.2886947545547,8.43139686737016));
#61595=CARTESIAN_POINT('Ctrl Pts',(-19.114608242428,35.289736378826,8.44067644774265));
#61596=CARTESIAN_POINT('Ctrl Pts',(-19.1043597959818,35.291976041947,8.46064449327679));
#61597=CARTESIAN_POINT('Ctrl Pts',(-19.0986916046772,35.2931716665292,8.47131107114716));
#61598=CARTESIAN_POINT('Ctrl Pts',(-19.0806262279321,35.2968575851035,8.50416706076701));
#61599=CARTESIAN_POINT('Ctrl Pts',(-19.0677135440715,35.2993189743541,8.52606821481939));
#61600=CARTESIAN_POINT('Ctrl Pts',(-19.0331663233633,35.3055271128824,8.58083591132089));
#61601=CARTESIAN_POINT('Ctrl Pts',(-19.0106459031221,35.3092368971343,8.61311277935803));
#61602=CARTESIAN_POINT('Ctrl Pts',(-18.9343301341607,35.3209909553499,8.7123309709433));
#61603=CARTESIAN_POINT('Ctrl Pts',(-18.8752576533315,35.3289562841321,8.77485929635222));
#61604=CARTESIAN_POINT('Ctrl Pts',(-18.8103597331144,35.3371716890844,8.83093845464842));
#61605=CARTESIAN_POINT('',(-19.2499996766479,35.3992235994469,7.87090626388281));
#61606=CARTESIAN_POINT('Ctrl Pts',(-18.8103598667433,35.5078191442546,8.83093833917793));
#61607=CARTESIAN_POINT('Ctrl Pts',(-18.8515678132402,35.5027089767599,8.7953299930782));
#61608=CARTESIAN_POINT('Ctrl Pts',(-18.8904541978799,35.497572108699,8.75709794336919));
#61609=CARTESIAN_POINT('Ctrl Pts',(-18.9439507250691,35.4898573324745,8.69726237873332));
#61610=CARTESIAN_POINT('Ctrl Pts',(-18.9605359892294,35.487360783695,8.67753513813323));
#61611=CARTESIAN_POINT('Ctrl Pts',(-18.9878084884195,35.483056640536,8.64301636285372));
#61612=CARTESIAN_POINT('Ctrl Pts',(-18.9987984684321,35.4812617180433,8.62847336212095));
#61613=CARTESIAN_POINT('Ctrl Pts',(-19.0209607232215,35.4775085024284,8.59779512631827));
#61614=CARTESIAN_POINT('Ctrl Pts',(-19.0320794515118,35.475548734079,8.58162749378194));
#61615=CARTESIAN_POINT('Ctrl Pts',(-19.0607753997425,35.4702736331078,8.53775789192916));
#61616=CARTESIAN_POINT('Ctrl Pts',(-19.0776597715214,35.4669341866036,8.50962379455912));
#61617=CARTESIAN_POINT('Ctrl Pts',(-19.1259370268866,35.4566062555776,8.42162882851243));
#61618=CARTESIAN_POINT('Ctrl Pts',(-19.1536546971673,35.4495123832065,8.35989594194129));
#61619=CARTESIAN_POINT('Ctrl Pts',(-19.1973008243931,35.435801773586,8.23740060329115));
#61620=CARTESIAN_POINT('Ctrl Pts',(-19.2139032321815,35.4292084285488,8.1770652332666));
#61621=CARTESIAN_POINT('Ctrl Pts',(-19.2292579596607,35.4210399546256,8.09921288195888));
#61622=CARTESIAN_POINT('Ctrl Pts',(-19.2321897530893,35.4193178642095,8.08261448104668));
#61623=CARTESIAN_POINT('Ctrl Pts',(-19.2364031339202,35.4165548032125,8.05563510989243));
#61624=CARTESIAN_POINT('Ctrl Pts',(-19.2378883742103,35.4155037624647,8.04528864374251));
#61625=CARTESIAN_POINT('Ctrl Pts',(-19.240484634935,35.4135075085774,8.02546537682624));
#61626=CARTESIAN_POINT('Ctrl Pts',(-19.2416168867057,35.4125609966872,8.01599263969534));
#61627=CARTESIAN_POINT('Ctrl Pts',(-19.243943451768,35.4104255878687,7.99447279776066));
#61628=CARTESIAN_POINT('Ctrl Pts',(-19.2450725099584,35.4092400452403,7.9824193440969));
#61629=CARTESIAN_POINT('Ctrl Pts',(-19.2486494174628,35.4048342121886,7.93729296580199));
#61630=CARTESIAN_POINT('Ctrl Pts',(-19.2499742154868,35.4016628870377,7.90414157193482));
#61631=CARTESIAN_POINT('Ctrl Pts',(-19.2499996272734,35.3985194419833,7.870972998107));
#61632=CARTESIAN_POINT('Ctrl Pts',(-19.2499996766479,35.3992235994469,7.87090626388281));
#61633=CARTESIAN_POINT('Ctrl Pts',(-19.2500344912314,35.394352505386,7.82211858663167));
#61634=CARTESIAN_POINT('Ctrl Pts',(-19.2472537597015,35.3894814113251,7.77322280597972));
#61635=CARTESIAN_POINT('Ctrl Pts',(-19.2416465304584,35.3846103172642,7.72457636993151));
#61636=CARTESIAN_POINT('Ctrl Pts',(-19.2360459798721,35.3797450250644,7.67598787566496));
#61637=CARTESIAN_POINT('Ctrl Pts',(-19.2276256512387,35.3748797328647,7.62764869637825));
#61638=CARTESIAN_POINT('Ctrl Pts',(-19.2164265935117,35.370014440665,7.57991504889593));
#61639=CARTESIAN_POINT('Ctrl Pts',(-19.2052357867004,35.3651527329735,7.5322165692205));
#61640=CARTESIAN_POINT('Ctrl Pts',(-19.1912704296199,35.3602910252821,7.48512328742696));
#61641=CARTESIAN_POINT('Ctrl Pts',(-19.1746228287216,35.3554293175907,7.43898225431278));
#61642=CARTESIAN_POINT('Ctrl Pts',(-19.1579799320472,35.3505689837046,7.39285425957897));
#61643=CARTESIAN_POINT('Ctrl Pts',(-19.1386564860787,35.3457086498184,7.34767851120752));
#61644=CARTESIAN_POINT('Ctrl Pts',(-19.1167940742142,35.3408483159322,7.30378517077739));
#61645=CARTESIAN_POINT('Ctrl Pts',(-19.0949127015831,35.3359837667904,7.25985376266356));
#61646=CARTESIAN_POINT('Ctrl Pts',(-19.070488219198,35.3311192176485,7.2172074898685));
#61647=CARTESIAN_POINT('Ctrl Pts',(-19.0437087262131,35.3262546685067,7.17615293776065));
#61648=CARTESIAN_POINT('Ctrl Pts',(-19.0169162706987,35.3213877646951,7.13507851332577));
#61649=CARTESIAN_POINT('Ctrl Pts',(-18.9877668730102,35.3165208608835,7.09559779715689));
#61650=CARTESIAN_POINT('Ctrl Pts',(-18.9564904780592,35.3116539570719,7.05798624010442));
#61651=CARTESIAN_POINT('Ctrl Pts',(-18.9251571018419,35.3067781864347,7.02030615999646));
#61652=CARTESIAN_POINT('Ctrl Pts',(-18.8916893857305,35.3019024157974,6.98450244311401));
#61653=CARTESIAN_POINT('Ctrl Pts',(-18.8563545143047,35.2970266451602,6.95081407470642));
#61654=CARTESIAN_POINT('Ctrl Pts',(-18.8398140587157,35.2947442690135,6.9350443566057));
#61655=CARTESIAN_POINT('Ctrl Pts',(-18.8228649403526,35.2924618928668,6.91973758270855));
#61656=CARTESIAN_POINT('Ctrl Pts',(-18.8055368501529,35.2901795167202,6.90491507677324));
#61657=CARTESIAN_POINT('Ctrl Pts',(-18.767971321095,35.2852315584356,6.87278139839276));
#61658=CARTESIAN_POINT('Ctrl Pts',(-18.728443728258,35.2802836001511,6.84277327078661));
#61659=CARTESIAN_POINT('Ctrl Pts',(-18.6872241374823,35.2753356418666,6.81513791452987));
#61660=CARTESIAN_POINT('Ctrl Pts',(-18.6460804186891,35.2703967911786,6.78755342605774));
#61661=CARTESIAN_POINT('Ctrl Pts',(-18.6032513303603,35.2654579404907,6.7623333493862));
#61662=CARTESIAN_POINT('Ctrl Pts',(-18.5590397616473,35.2605190898028,6.73968457746013));
#61663=CARTESIAN_POINT('Ctrl Pts',(-18.5148731026843,35.255585255959,6.71705881197143));
#61664=CARTESIAN_POINT('Ctrl Pts',(-18.469327228762,35.2506514221152,6.69699942920419));
#61665=CARTESIAN_POINT('Ctrl Pts',(-18.4227319086503,35.2457175882714,6.67966876162019));
#61666=CARTESIAN_POINT('Ctrl Pts',(-18.3761640900494,35.2407866664772,6.66234832295057));
#61667=CARTESIAN_POINT('Ctrl Pts',(-18.3285485649792,35.2358557446831,6.64775359959792));
#61668=CARTESIAN_POINT('Ctrl Pts',(-18.280235100339,35.2309248228889,6.63599883123053));
#61669=CARTESIAN_POINT('Ctrl Pts',(-18.2319295917507,35.2259947130976,6.62424599858743));
#61670=CARTESIAN_POINT('Ctrl Pts',(-18.18292690417,35.2210646033062,6.61533232101275));
#61671=CARTESIAN_POINT('Ctrl Pts',(-18.1335894622256,35.2161344935149,6.60932150129652));
#61672=CARTESIAN_POINT('Ctrl Pts',(-18.0842038074302,35.21119956599,6.60330480777039));
#61673=CARTESIAN_POINT('Ctrl Pts',(-18.0344832902771,35.2062646384652,6.6001967012733));
#61674=CARTESIAN_POINT('Ctrl Pts',(-17.9847961574757,35.2013297109403,6.60000905638132));
#61675=CARTESIAN_POINT('Ctrl Pts',(-17.9350822971657,35.1963921288385,6.59982131055213));
#61676=CARTESIAN_POINT('Ctrl Pts',(-17.8854024046964,35.1914545467366,6.60255712443852));
#61677=CARTESIAN_POINT('Ctrl Pts',(-17.8361218523175,35.1865169646348,6.60817628861261));
#61678=CARTESIAN_POINT('Ctrl Pts',(-17.7867492134293,35.18157015608,6.61380595285597));
#61679=CARTESIAN_POINT('Ctrl Pts',(-17.7377779441546,35.1766233475252,6.62232962690223));
#61680=CARTESIAN_POINT('Ctrl Pts',(-17.6895638312621,35.1716765389703,6.63365586025215));
#61681=CARTESIAN_POINT('Ctrl Pts',(-17.6650865304908,35.1691651473136,6.63940595298807));
#61682=CARTESIAN_POINT('Ctrl Pts',(-17.6408041417708,35.1666537556569,6.64587757037487));
#61683=CARTESIAN_POINT('Ctrl Pts',(-17.6167614138093,35.1641423640002,6.65305393319909));
#61684=CARTESIAN_POINT('Ctrl Pts',(-17.5693934527408,35.1591945268656,6.66719249831603));
#61685=CARTESIAN_POINT('Ctrl Pts',(-17.5227474291937,35.1542466897311,6.68413207344764));
#61686=CARTESIAN_POINT('Ctrl Pts',(-17.4771774928875,35.1492988525965,6.70377981223909));
#61687=CARTESIAN_POINT('Ctrl Pts',(-17.4316914400847,35.144360123263,6.72339138417806));
#61688=CARTESIAN_POINT('Ctrl Pts',(-17.3872780450423,35.1394213939295,6.7457010174851));
#61689=CARTESIAN_POINT('Ctrl Pts',(-17.3442753732749,35.134482664596,6.77056641902512));
#61690=CARTESIAN_POINT('Ctrl Pts',(-17.3013163845637,35.129548952132,6.79540656174545));
#61691=CARTESIAN_POINT('Ctrl Pts',(-17.259765754346,35.1246152396679,6.8227970601231));
#61692=CARTESIAN_POINT('Ctrl Pts',(-17.2199386839969,35.1196815272039,6.85254887295969));
#61693=CARTESIAN_POINT('Ctrl Pts',(-17.1801351193651,35.1147507265897,6.88228312644039));
#61694=CARTESIAN_POINT('Ctrl Pts',(-17.142053537651,35.1098199259756,6.91437560618114));
#61695=CARTESIAN_POINT('Ctrl Pts',(-17.1059795762881,35.1048891253614,6.94859438956857));
#61696=CARTESIAN_POINT('Ctrl Pts',(-17.0699115524682,35.0999591363255,6.98280754076345));
#61697=CARTESIAN_POINT('Ctrl Pts',(-17.0358508897038,35.0950291472895,7.01914592315566));
#61698=CARTESIAN_POINT('Ctrl Pts',(-17.0040476272454,35.0900991582536,7.0573395751517));
#61699=CARTESIAN_POINT('Ctrl Pts',(-16.9722132754166,35.0851643498927,7.09557056346179));
#61700=CARTESIAN_POINT('Ctrl Pts',(-16.9426410804493,35.0802295415318,7.1356600198791));
#61701=CARTESIAN_POINT('Ctrl Pts',(-16.9155406916189,35.0752947331709,7.17730498716906));
#61702=CARTESIAN_POINT('Ctrl Pts',(-16.8884257206899,35.0703572695027,7.21897236266217));
#61703=CARTESIAN_POINT('Ctrl Pts',(-16.8637854760545,35.0654198058345,7.26219643912664));
#61704=CARTESIAN_POINT('Ctrl Pts',(-16.8417842860779,35.0604823421662,7.3066484325213));
#61705=CARTESIAN_POINT('Ctrl Pts',(-16.8197419720682,35.0555356495236,7.35118351438731));
#61706=CARTESIAN_POINT('Ctrl Pts',(-16.8003487719911,35.050588956881,7.39695058922179));
#61707=CARTESIAN_POINT('Ctrl Pts',(-16.7837207625441,35.0456422642383,7.44360114208405));
#61708=CARTESIAN_POINT('Ctrl Pts',(-16.7752756459888,35.0431299132523,7.46729425806099));
#61709=CARTESIAN_POINT('Ctrl Pts',(-16.7675430004651,35.0406175622662,7.49121502811406));
#61710=CARTESIAN_POINT('Ctrl Pts',(-16.760533003051,35.0381052112801,7.5153166999249));
#61711=CARTESIAN_POINT('Ctrl Pts',(-16.7467269258535,35.0331571764077,7.56278455503975));
#61712=CARTESIAN_POINT('Ctrl Pts',(-16.7356659974402,35.0282091415352,7.6111646853601));
#61713=CARTESIAN_POINT('Ctrl Pts',(-16.7274642386308,35.0232611066628,7.66010915577047));
#61714=CARTESIAN_POINT('Ctrl Pts',(-16.7192775789955,35.0183221809633,7.70896352098631));
#61715=CARTESIAN_POINT('Ctrl Pts',(-16.7139397392205,35.0133832552638,7.75837962969513));
#61716=CARTESIAN_POINT('Ctrl Pts',(-16.7115144718757,35.0084443295642,7.80799625060427));
#61717=CARTESIAN_POINT('Ctrl Pts',(-16.7090916685677,35.0035104217424,7.85756246173853));
#61718=CARTESIAN_POINT('Ctrl Pts',(-16.7095756062566,34.9985765139205,7.90732823709241));
#61719=CARTESIAN_POINT('Ctrl Pts',(-16.7129783607682,34.9936426060986,7.95692620846578));
#61720=CARTESIAN_POINT('Ctrl Pts',(-16.716379106136,34.9887116114841,8.00649489490266));
#61721=CARTESIAN_POINT('Ctrl Pts',(-16.7226952167604,34.9837806168697,8.05589542796928));
#61722=CARTESIAN_POINT('Ctrl Pts',(-16.7318867077665,34.9788496222552,8.10476202791346));
#61723=CARTESIAN_POINT('Ctrl Pts',(-16.7410766827878,34.9739194409269,8.15362056811811));
#61724=CARTESIAN_POINT('Ctrl Pts',(-16.7531409944929,34.9689892595987,8.2019448119657));
#61725=CARTESIAN_POINT('Ctrl Pts',(-16.7679883939252,34.9640590782704,8.24937826339945));
#61726=CARTESIAN_POINT('Ctrl Pts',(-16.7828502946507,34.9591240816878,8.29685804256821));
#61727=CARTESIAN_POINT('Ctrl Pts',(-16.8005005453532,34.9541890851052,8.3434447685477));
#61728=CARTESIAN_POINT('Ctrl Pts',(-16.8207982721191,34.9492540885226,8.38879798966256));
#61729=CARTESIAN_POINT('Ctrl Pts',(-16.8411069118241,34.9443164386715,8.43417559463809));
#61730=CARTESIAN_POINT('Ctrl Pts',(-16.864065608919,34.9393787888205,8.47831788748006));
#61731=CARTESIAN_POINT('Ctrl Pts',(-16.8894872135768,34.9344411389694,8.52090849022546));
#61732=CARTESIAN_POINT('Ctrl Pts',(-16.9149563064051,34.9294942654694,8.56357865324362));
#61733=CARTESIAN_POINT('Ctrl Pts',(-16.9428971811849,34.9245473919694,8.60469088746089));
#61734=CARTESIAN_POINT('Ctrl Pts',(-16.9730799447014,34.9196005184694,8.64395865667199));
#61735=CARTESIAN_POINT('Ctrl Pts',(-16.9883994157531,34.9170896984997,8.66388928540193));
#61736=CARTESIAN_POINT('Ctrl Pts',(-17.0042957956781,34.9145788785299,8.68334529920754));
#61737=CARTESIAN_POINT('Ctrl Pts',(-17.020735385823,34.9120680585602,8.7022928571049));
#61738=CARTESIAN_POINT('Ctrl Pts',(-17.0531329800926,34.9071199712936,8.73963291776023));
#61739=CARTESIAN_POINT('Ctrl Pts',(-17.0877856780777,34.902171884027,8.77516103834506));
#61740=CARTESIAN_POINT('Ctrl Pts',(-17.1244629481944,34.8972237967604,8.80859275140382));
#61741=CARTESIAN_POINT('Ctrl Pts',(-17.161072725266,34.892284814901,8.84196294385018));
#61742=CARTESIAN_POINT('Ctrl Pts',(-17.1996992836833,34.8873458330415,8.87324401392446));
#61743=CARTESIAN_POINT('Ctrl Pts',(-17.2400736637485,34.8824068511821,8.90218652235024));
#61744=CARTESIAN_POINT('Ctrl Pts',(-17.2804070430736,34.8774728849269,8.93109963925923));
#61745=CARTESIAN_POINT('Ctrl Pts',(-17.3224842870685,34.8725389186717,8.95767857817394));
#61746=CARTESIAN_POINT('Ctrl Pts',(-17.3660032597972,34.8676049524165,8.98171399335457));
#61747=CARTESIAN_POINT('Ctrl Pts',(-17.4094965560649,34.8626738972317,9.00573522749272));
#61748=CARTESIAN_POINT('Ctrl Pts',(-17.4544294171664,34.8577428420468,9.02721564641119));
#61749=CARTESIAN_POINT('Ctrl Pts',(-17.5004728137367,34.852811786862,9.04599050916));
#61750=CARTESIAN_POINT('Ctrl Pts',(-17.5465086350115,34.8478815429597,9.06476228297218));
#61751=CARTESIAN_POINT('Ctrl Pts',(-17.5936541215318,34.8429512990573,9.08082917843513));
#61752=CARTESIAN_POINT('Ctrl Pts',(-17.6415602480993,34.8380210551549,9.09407456240763));
#61753=CARTESIAN_POINT('Ctrl Pts',(-17.6895131876216,34.8330859935121,9.10733288951712));
#61754=CARTESIAN_POINT('Ctrl Pts',(-17.7382277218037,34.8281509318693,9.11776405488851));
#61755=CARTESIAN_POINT('Ctrl Pts',(-17.7873413986063,34.8232158702265,9.1253018215987));
#61756=CARTESIAN_POINT('Ctrl Pts',(-17.8364814957183,34.8182781538067,9.13284364319018));
#61757=CARTESIAN_POINT('Ctrl Pts',(-17.8860206168876,34.813340437387,9.13748891546799));
#61758=CARTESIAN_POINT('Ctrl Pts',(-17.9355914456565,34.8084027209673,9.13922333743952));
#61759=CARTESIAN_POINT('Ctrl Pts',(-17.9852548879054,34.803455779382,9.14096099984214));
#61760=CARTESIAN_POINT('Ctrl Pts',(-18.0349496078833,34.7985088377967,9.13977697070298));
#61761=CARTESIAN_POINT('Ctrl Pts',(-18.0843101863803,34.7935618962114,9.13570904437683));
#61762=CARTESIAN_POINT('Ctrl Pts',(-18.109358258,34.7910515660877,9.13364477136659));
#61763=CARTESIAN_POINT('Ctrl Pts',(-18.1343204007753,34.7885412359639,9.13083870360194));
#61764=CARTESIAN_POINT('Ctrl Pts',(-18.1591499362204,34.7860309058402,9.12730079947171));
#61765=CARTESIAN_POINT('Ctrl Pts',(-18.2080779265591,34.7810841597235,9.12032916121915));
#61766=CARTESIAN_POINT('Ctrl Pts',(-18.256706745439,34.7761374136069,9.11048175221321));
#61767=CARTESIAN_POINT('Ctrl Pts',(-18.3046725750274,34.7711906674902,9.09779791457107));
#61768=CARTESIAN_POINT('Ctrl Pts',(-18.3525545270608,34.7662525717185,9.08513625707881));
#61769=CARTESIAN_POINT('Ctrl Pts',(-18.3997752627025,34.7613144759467,9.0696481430095));
#61770=CARTESIAN_POINT('Ctrl Pts',(-18.4459794440344,34.756376380175,9.05142420736049));
#61771=CARTESIAN_POINT('Ctrl Pts',(-18.4921354873705,34.7514434291764,9.03321925838572));
#61772=CARTESIAN_POINT('Ctrl Pts',(-18.5372765661141,34.7465104781779,9.01228433207194));
#61773=CARTESIAN_POINT('Ctrl Pts',(-18.5810630567823,34.7415775271793,8.988759671141));
#61774=CARTESIAN_POINT('Ctrl Pts',(-18.6248340498064,34.736646322133,8.96524333644988));
#61775=CARTESIAN_POINT('Ctrl Pts',(-18.6672509155311,34.7317151170866,8.93913932917656));
#61776=CARTESIAN_POINT('Ctrl Pts',(-18.7079966954101,34.7267839120402,8.91063481177208));
#61777=CARTESIAN_POINT('Ctrl Pts',(-18.7434460223,34.7224937033323,8.88583553296801));
#61778=CARTESIAN_POINT('Ctrl Pts',(-18.7776306342101,34.7182034946243,8.85922010858513));
#61779=CARTESIAN_POINT('Ctrl Pts',(-18.810359785549,34.7139132859163,8.83093840933901));
#61780=CARTESIAN_POINT('Origin',(-17.98,41.616,7.87));
#61781=CARTESIAN_POINT('',(-19.6843398922845,41.2062399153875,7.87060594373627));
#61782=CARTESIAN_POINT('',(-17.1849388579978,41.466,9.37753196187617));
#61783=CARTESIAN_POINT('Ctrl Pts',(-19.6843398922843,41.2062399154299,7.87060594430517));
#61784=CARTESIAN_POINT('Ctrl Pts',(-19.6843297548994,41.2083658452999,7.89911937250543));
#61785=CARTESIAN_POINT('Ctrl Pts',(-19.6836041205795,41.2104917751699,7.92762031499746));
#61786=CARTESIAN_POINT('Ctrl Pts',(-19.6821646062297,41.2126177050399,7.95608419656944));
#61787=CARTESIAN_POINT('Ctrl Pts',(-19.6790461708081,41.217223129787,8.01774580941962));
#61788=CARTESIAN_POINT('Ctrl Pts',(-19.6725665498035,41.2218285545341,8.0793623765154));
#61789=CARTESIAN_POINT('Ctrl Pts',(-19.662730990455,41.2264339792812,8.1405388130422));
#61790=CARTESIAN_POINT('Ctrl Pts',(-19.6527449850825,41.2311098492178,8.20265101247922));
#61791=CARTESIAN_POINT('Ctrl Pts',(-19.639299442682,41.2357857191544,8.26430897234697));
#61792=CARTESIAN_POINT('Ctrl Pts',(-19.6224549301031,41.240461589091,8.32510069015551));
#61793=CARTESIAN_POINT('Ctrl Pts',(-19.6059100966222,41.2450542710768,8.38481086837807));
#61794=CARTESIAN_POINT('Ctrl Pts',(-19.5860863879309,41.2496469530625,8.44368486568653));
#61795=CARTESIAN_POINT('Ctrl Pts',(-19.5630928339961,41.2542396350482,8.50134136134915));
#61796=CARTESIAN_POINT('Ctrl Pts',(-19.5401135995693,41.2588294568868,8.55896195074625));
#61797=CARTESIAN_POINT('Ctrl Pts',(-19.5139686221421,41.2634192787255,8.61536607210285));
#61798=CARTESIAN_POINT('Ctrl Pts',(-19.4848161204918,41.2680091005641,8.67018952699211));
#61799=CARTESIAN_POINT('Ctrl Pts',(-19.4556711671333,41.2725977339862,8.72499878675562));
#61800=CARTESIAN_POINT('Ctrl Pts',(-19.4235204735083,41.2771863674083,8.77822774507018));
#61801=CARTESIAN_POINT('Ctrl Pts',(-19.388568653054,41.2817750008305,8.82953592180468));
#61802=CARTESIAN_POINT('Ctrl Pts',(-19.3524639576039,41.2865149889079,8.88253648289208));
#61803=CARTESIAN_POINT('Ctrl Pts',(-19.3133703749539,41.2912549769854,8.93348681834103));
#61804=CARTESIAN_POINT('Ctrl Pts',(-19.2715611413291,41.2959949650628,8.98204525708659));
#61805=CARTESIAN_POINT('Ctrl Pts',(-19.231038090852,41.3005891362416,9.02910988596817));
#61806=CARTESIAN_POINT('Ctrl Pts',(-19.1879644814571,41.3051833074203,9.07392733321175));
#61807=CARTESIAN_POINT('Ctrl Pts',(-19.1426275072298,41.309777478599,9.11622314014492));
#61808=CARTESIAN_POINT('Ctrl Pts',(-19.0951320706632,41.3145903751258,9.16053262152224));
#61809=CARTESIAN_POINT('Ctrl Pts',(-19.0451528230316,41.3194032716526,9.20207392159138));
#61810=CARTESIAN_POINT('Ctrl Pts',(-18.993057510963,41.3242161681794,9.24057991926101));
#61811=CARTESIAN_POINT('Ctrl Pts',(-18.9409621988943,41.3290290647063,9.27908591693065));
#61812=CARTESIAN_POINT('Ctrl Pts',(-18.8867513907459,41.3338419612331,9.31455632656212));
#61813=CARTESIAN_POINT('Ctrl Pts',(-18.8308232061203,41.3386548577599,9.34677848966159));
#61814=CARTESIAN_POINT('Ctrl Pts',(-18.7773644336064,41.3432552491776,9.37757793896555));
#61815=CARTESIAN_POINT('Ctrl Pts',(-18.7221236056583,41.3478556405953,9.40553281345446));
#61816=CARTESIAN_POINT('Ctrl Pts',(-18.6654351944846,41.352456032013,9.43043373129454));
#61817=CARTESIAN_POINT('Ctrl Pts',(-18.607808944907,41.3571325311158,9.45574660347523));
#61818=CARTESIAN_POINT('Ctrl Pts',(-18.5486871913394,41.3618090302186,9.47790320675449));
#61819=CARTESIAN_POINT('Ctrl Pts',(-18.4884499478873,41.3664855293214,9.49673092000287));
#61820=CARTESIAN_POINT('Ctrl Pts',(-18.429352925331,41.3710735077401,9.51520224655699));
#61821=CARTESIAN_POINT('Ctrl Pts',(-18.3691827828313,41.3756614861588,9.53046945305033));
#61822=CARTESIAN_POINT('Ctrl Pts',(-18.3083186592228,41.3802494645776,9.54241791834642));
#61823=CARTESIAN_POINT('Ctrl Pts',(-18.2474906919437,41.3848347175079,9.55435928565732));
#61824=CARTESIAN_POINT('Ctrl Pts',(-18.1859700586657,41.3894199704383,9.5629857235566));
#61825=CARTESIAN_POINT('Ctrl Pts',(-18.124148111573,41.3940052233687,9.56823324591469));
#61826=CARTESIAN_POINT('Ctrl Pts',(-18.0623402869642,41.398589428853,9.57347956953909));
#61827=CARTESIAN_POINT('Ctrl Pts',(-18.0002317912689,41.4031736343372,9.57534846713863));
#61828=CARTESIAN_POINT('Ctrl Pts',(-17.9382191172373,41.4077578398214,9.57382780627491));
#61829=CARTESIAN_POINT('Ctrl Pts',(-17.8740378725548,41.4125023540429,9.57225396820878));
#61830=CARTESIAN_POINT('Ctrl Pts',(-17.8099598551421,41.4172468682645,9.56704906035075));
#61831=CARTESIAN_POINT('Ctrl Pts',(-17.7464220591415,41.421991382486,9.5582583277284));
#61832=CARTESIAN_POINT('Ctrl Pts',(-17.684951616891,41.4265815226202,9.54975362256054));
#61833=CARTESIAN_POINT('Ctrl Pts',(-17.623987280821,41.4311716627544,9.53789304749754));
#61834=CARTESIAN_POINT('Ctrl Pts',(-17.5639146254392,41.4357618028886,9.52276973492276));
#61835=CARTESIAN_POINT('Ctrl Pts',(-17.5008114542963,41.4405835041538,9.50688348891632));
#61836=CARTESIAN_POINT('Ctrl Pts',(-17.4386929277687,41.445405205419,9.48739676187291));
#61837=CARTESIAN_POINT('Ctrl Pts',(-17.3779852245854,41.4502269066842,9.46447579027794));
#61838=CARTESIAN_POINT('Ctrl Pts',(-17.3172775214021,41.4550486079494,9.44155481868298));
#61839=CARTESIAN_POINT('Ctrl Pts',(-17.2579811963998,41.4598703092146,9.41519993318898));
#61840=CARTESIAN_POINT('Ctrl Pts',(-17.2004925879047,41.4646920104799,9.38563288103963));
#61841=CARTESIAN_POINT('Ctrl Pts',(-17.1952942499942,41.4651280069866,9.38295931610016));
#61842=CARTESIAN_POINT('Ctrl Pts',(-17.1901096143734,41.4655640034933,9.38025898032286));
#61843=CARTESIAN_POINT('Ctrl Pts',(-17.1849388579978,41.466,9.37753196187617));
#61844=CARTESIAN_POINT('',(-18.7752089275578,41.466,9.37745401161438));
#61845=CARTESIAN_POINT('Origin',(-17.98,41.466,7.87));
#61846=CARTESIAN_POINT('',(-19.6846890250508,41.3288850845701,7.87133229203072));
#61847=CARTESIAN_POINT('Ctrl Pts',(-18.7752089275578,41.466,9.3774540116144));
#61848=CARTESIAN_POINT('Ctrl Pts',(-19.276531813104,41.42398761576,9.11299723143809));
#61849=CARTESIAN_POINT('Ctrl Pts',(-19.6623171952346,41.3782826439501,8.53412813453988));
#61850=CARTESIAN_POINT('Ctrl Pts',(-19.6866056581082,41.3325776721401,7.92091522847425));
#61851=CARTESIAN_POINT('Ctrl Pts',(-19.6862873905421,41.3288850845701,7.87133354122607));
#61852=CARTESIAN_POINT('',(-19.6843397066618,40.5351350846263,7.8709999479683));
#61853=CARTESIAN_POINT('Ctrl Pts',(-19.6843394794834,41.3288850845701,7.87133201884495));
#61854=CARTESIAN_POINT('Ctrl Pts',(-19.6843866948718,41.3243806806803,7.81091917197142));
#61855=CARTESIAN_POINT('Ctrl Pts',(-19.6812175888757,41.3198762767905,7.75035564495815));
#61856=CARTESIAN_POINT('Ctrl Pts',(-19.6748105177055,41.3153718729006,7.69002182167091));
#61857=CARTESIAN_POINT('Ctrl Pts',(-19.6684144011613,41.310875170511,7.62979115541847));
#61858=CARTESIAN_POINT('Ctrl Pts',(-19.6587913527375,41.3063784681213,7.56978993681637));
#61859=CARTESIAN_POINT('Ctrl Pts',(-19.6459717276017,41.3018817657316,7.51039877860063));
#61860=CARTESIAN_POINT('Ctrl Pts',(-19.6331641670414,41.2973892951978,7.45106351352582));
#61861=CARTESIAN_POINT('Ctrl Pts',(-19.6171660950037,41.292896824664,7.39233768859054));
#61862=CARTESIAN_POINT('Ctrl Pts',(-19.5980594616066,41.2884043541301,7.33459509312552));
#61863=CARTESIAN_POINT('Ctrl Pts',(-19.5789631759451,41.2839143166203,7.27688376978966));
#61864=CARTESIAN_POINT('Ctrl Pts',(-19.5567618295966,41.2794242791104,7.22015512428743));
#61865=CARTESIAN_POINT('Ctrl Pts',(-19.5315874972659,41.2749342416005,7.16476877981176));
#61866=CARTESIAN_POINT('Ctrl Pts',(-19.5064167450557,41.270444842633,7.10939031200142));
#61867=CARTESIAN_POINT('Ctrl Pts',(-19.4782740666417,41.2659554436654,7.05535424892268));
#61868=CARTESIAN_POINT('Ctrl Pts',(-19.4473391225447,41.2614660446978,7.00299899939525));
#61869=CARTESIAN_POINT('Ctrl Pts',(-19.4163750901459,41.2569724243231,6.95059451993223));
#61870=CARTESIAN_POINT('Ctrl Pts',(-19.3826138226266,41.2524788039485,6.89987446610507));
#61871=CARTESIAN_POINT('Ctrl Pts',(-19.3462794884679,41.2479851835738,6.85115006257451));
#61872=CARTESIAN_POINT('Ctrl Pts',(-19.309926421075,41.243489246381,6.80240053774533));
#61873=CARTESIAN_POINT('Ctrl Pts',(-19.2709979904377,41.2389933091883,6.7556491157724));
#61874=CARTESIAN_POINT('Ctrl Pts',(-19.2297579082109,41.2344973719955,6.7111730040837));
#61875=CARTESIAN_POINT('Ctrl Pts',(-19.1884442914886,41.2299934181729,6.66661758779002));
#61876=CARTESIAN_POINT('Ctrl Pts',(-19.144811183237,41.2254894643503,6.62434594199744));
#61877=CARTESIAN_POINT('Ctrl Pts',(-19.0991572632189,41.2209855105278,6.58459661748367));
#61878=CARTESIAN_POINT('Ctrl Pts',(-19.0753035348257,41.2186322385385,6.56382798271176));
#61879=CARTESIAN_POINT('Ctrl Pts',(-19.0508986500405,41.2162789665492,6.54374723572351));
#61880=CARTESIAN_POINT('Ctrl Pts',(-19.0259882433092,41.2139256945599,6.52438362433455));
#61881=CARTESIAN_POINT('Ctrl Pts',(-18.9772850169631,41.2093247284022,6.48652513577091));
#61882=CARTESIAN_POINT('Ctrl Pts',(-18.9264242815211,41.2047237622444,6.45123686267388));
#61883=CARTESIAN_POINT('Ctrl Pts',(-18.8737080489061,41.2001227960866,6.41877267152234));
#61884=CARTESIAN_POINT('Ctrl Pts',(-18.8201272098375,41.1954463688263,6.38577603053915));
#61885=CARTESIAN_POINT('Ctrl Pts',(-18.7646298188562,41.1907699415661,6.35569734333755));
#61886=CARTESIAN_POINT('Ctrl Pts',(-18.7075679961142,41.1860935143058,6.32876035392596));
#61887=CARTESIAN_POINT('Ctrl Pts',(-18.6515825471548,41.181505299855,6.30233148479151));
#61888=CARTESIAN_POINT('Ctrl Pts',(-18.5940916556415,41.1769170854042,6.27892704307211));
#61889=CARTESIAN_POINT('Ctrl Pts',(-18.535454767159,41.1723288709535,6.25871329762815));
#61890=CARTESIAN_POINT('Ctrl Pts',(-18.4768543255166,41.1677435083921,6.23851211641068));
#61891=CARTESIAN_POINT('Ctrl Pts',(-18.4171097787433,41.1631581458306,6.22149786398388));
#61892=CARTESIAN_POINT('Ctrl Pts',(-18.3565997339616,41.1585727832692,6.20778837809981));
#61893=CARTESIAN_POINT('Ctrl Pts',(-18.2961051769494,41.1539885943483,6.19408240120928));
#61894=CARTESIAN_POINT('Ctrl Pts',(-18.234846006181,41.1494044054274,6.18367962387388));
#61895=CARTESIAN_POINT('Ctrl Pts',(-18.1732131575983,41.1448202165064,6.17664725726418));
#61896=CARTESIAN_POINT('Ctrl Pts',(-18.1094275867881,41.1400759102842,6.16936926300203));
#61897=CARTESIAN_POINT('Ctrl Pts',(-18.04524231703,41.135331604062,6.16570161710359));
#61898=CARTESIAN_POINT('Ctrl Pts',(-17.9810963851869,41.1305872978398,6.16566035264695));
#61899=CARTESIAN_POINT('Ctrl Pts',(-17.9190393268576,41.1259974870833,6.16562043194241));
#61900=CARTESIAN_POINT('Ctrl Pts',(-17.8570196058036,41.1214076763267,6.16897422181227));
#61901=CARTESIAN_POINT('Ctrl Pts',(-17.7954320279454,41.1168178655701,6.17568317623543));
#61902=CARTESIAN_POINT('Ctrl Pts',(-17.7307348442592,41.1119963116151,6.18273087110756));
#61903=CARTESIAN_POINT('Ctrl Pts',(-17.6665152310406,41.1071747576601,6.19348144054158));
#61904=CARTESIAN_POINT('Ctrl Pts',(-17.6032185001076,41.1023532037051,6.20782957042942));
#61905=CARTESIAN_POINT('Ctrl Pts',(-17.5399217691746,41.0975316497501,6.22217770031727));
#61906=CARTESIAN_POINT('Ctrl Pts',(-17.4775485166543,41.092710095795,6.24012314150737));
#61907=CARTESIAN_POINT('Ctrl Pts',(-17.4165222859492,41.08788854184,6.26150141393656));
#61908=CARTESIAN_POINT('Ctrl Pts',(-17.3582416607155,41.0832839123905,6.28191786550494));
#61909=CARTESIAN_POINT('Ctrl Pts',(-17.3009568035062,41.078679282941,6.30554629026167));
#61910=CARTESIAN_POINT('Ctrl Pts',(-17.2450450522227,41.0740746534915,6.33226918469528));
#61911=CARTESIAN_POINT('Ctrl Pts',(-17.1882670556202,41.0693986841427,6.35940609911008));
#61912=CARTESIAN_POINT('Ctrl Pts',(-17.1329056035329,41.0647227147939,6.38973409954295));
#61913=CARTESIAN_POINT('Ctrl Pts',(-17.0793386582792,41.0600467454451,6.42307775498139));
#61914=CARTESIAN_POINT('Ctrl Pts',(-17.0267296199213,41.0554543937687,6.45582514499298));
#61915=CARTESIAN_POINT('Ctrl Pts',(-16.975851882681,41.0508620420924,6.49148093951536));
#61916=CARTESIAN_POINT('Ctrl Pts',(-16.9270400206117,41.0462696904161,6.52983205626807));
#61917=CARTESIAN_POINT('Ctrl Pts',(-16.8782567130356,41.0416800252235,6.56816073796811));
#61918=CARTESIAN_POINT('Ctrl Pts',(-16.8315372819656,41.0370903600309,6.60918130230569));
#61919=CARTESIAN_POINT('Ctrl Pts',(-16.7871858627384,41.0325006948383,6.65263839819519));
#61920=CARTESIAN_POINT('Ctrl Pts',(-16.7428442520281,41.0279120446709,6.69608588335138));
#61921=CARTESIAN_POINT('Ctrl Pts',(-16.7008699753855,41.0233233945036,6.74196847535455));
#61922=CARTESIAN_POINT('Ctrl Pts',(-16.661531204894,41.0187347443362,6.78999311486839));
#61923=CARTESIAN_POINT('Ctrl Pts',(-16.6208925062568,41.0139944647348,6.83960470231698));
#61924=CARTESIAN_POINT('Ctrl Pts',(-16.5830669622976,41.0092541851335,6.89150198562179));
#61925=CARTESIAN_POINT('Ctrl Pts',(-16.5483043515794,41.0045139055321,6.94532578391436));
#61926=CARTESIAN_POINT('Ctrl Pts',(-16.5146099480799,40.9999192882037,6.99749565090883));
#61927=CARTESIAN_POINT('Ctrl Pts',(-16.4837931429944,40.9953246708752,7.05147484627626));
#61928=CARTESIAN_POINT('Ctrl Pts',(-16.4560352914342,40.9907300535467,7.10690996425982));
#61929=CARTESIAN_POINT('Ctrl Pts',(-16.4269574370992,40.9859169428089,7.16498125563029));
#61930=CARTESIAN_POINT('Ctrl Pts',(-16.4012370162303,40.9811038320712,7.22464983658376));
#61931=CARTESIAN_POINT('Ctrl Pts',(-16.3790253705987,40.9762907213334,7.2854873212552));
#61932=CARTESIAN_POINT('Ctrl Pts',(-16.3568137249671,40.9714776105956,7.34632480592664));
#61933=CARTESIAN_POINT('Ctrl Pts',(-16.3381109649799,40.9666644998578,7.40833056814371));
#61934=CARTESIAN_POINT('Ctrl Pts',(-16.3230075849423,40.96185138912,7.47106269660345));
#61935=CARTESIAN_POINT('Ctrl Pts',(-16.3085974875573,40.9572592121183,7.53091526457315));
#61936=CARTESIAN_POINT('Ctrl Pts',(-16.297404288211,40.9526670351166,7.59167509726248));
#61937=CARTESIAN_POINT('Ctrl Pts',(-16.2895355067767,40.948074858115,7.65296398282477));
#61938=CARTESIAN_POINT('Ctrl Pts',(-16.2815204783959,40.9433973322102,7.71539196628199));
#61939=CARTESIAN_POINT('Ctrl Pts',(-16.2769549193851,40.9387198063054,7.77836837361361));
#61940=CARTESIAN_POINT('Ctrl Pts',(-16.2758986568412,40.9340422804006,7.84147899292875));
#61941=CARTESIAN_POINT('Ctrl Pts',(-16.2748645615653,40.9294629194556,7.90326514039034));
#61942=CARTESIAN_POINT('Ctrl Pts',(-16.277193903632,40.9248835585105,7.96517938415097));
#61943=CARTESIAN_POINT('Ctrl Pts',(-16.2828906552653,40.9203041975655,8.0268269989961));
#61944=CARTESIAN_POINT('Ctrl Pts',(-16.2885838605718,40.9157276873521,8.08843623713104));
#61945=CARTESIAN_POINT('Ctrl Pts',(-16.2976402723845,40.9111511771387,8.1497786683519));
#61946=CARTESIAN_POINT('Ctrl Pts',(-16.310011835137,40.9065746669254,8.21046198733116));
#61947=CARTESIAN_POINT('Ctrl Pts',(-16.3223802683048,40.9019993144135,8.27112995549418));
#61948=CARTESIAN_POINT('Ctrl Pts',(-16.3380620859271,40.8974239619016,8.33113864254121));
#61949=CARTESIAN_POINT('Ctrl Pts',(-16.3569580144493,40.8928486093897,8.3901053246598));
#61950=CARTESIAN_POINT('Ctrl Pts',(-16.376587056374,40.8880957449739,8.45135976230815));
#61951=CARTESIAN_POINT('Ctrl Pts',(-16.3996846056663,40.8833428805581,8.51148910210795));
#61952=CARTESIAN_POINT('Ctrl Pts',(-16.4260830286562,40.8785900161422,8.57008348200035));
#61953=CARTESIAN_POINT('Ctrl Pts',(-16.4515275362989,40.8740088979823,8.62656053548045));
#61954=CARTESIAN_POINT('Ctrl Pts',(-16.4800381188257,40.8694277798224,8.68161123322365));
#61955=CARTESIAN_POINT('Ctrl Pts',(-16.5114173684656,40.8648466616624,8.73489299335561));
#61956=CARTESIAN_POINT('Ctrl Pts',(-16.5428188313569,40.8602623005464,8.78821247144266));
#61957=CARTESIAN_POINT('Ctrl Pts',(-16.5770927170495,40.8556779394304,8.83976009758077));
#61958=CARTESIAN_POINT('Ctrl Pts',(-16.6139988800237,40.8510935783143,8.88922312366992));
#61959=CARTESIAN_POINT('Ctrl Pts',(-16.6509666238722,40.8465015678264,8.93876868276023));
#61960=CARTESIAN_POINT('Ctrl Pts',(-16.6905750740438,40.8419095573385,8.98622231814517));
#61961=CARTESIAN_POINT('Ctrl Pts',(-16.7325454664175,40.8373175468506,9.03130617075968));
#61962=CARTESIAN_POINT('Ctrl Pts',(-16.737125488584,40.836816443367,9.03622594950479));
#61963=CARTESIAN_POINT('Ctrl Pts',(-16.7417336040733,40.8363153398835,9.04111754694237));
#61964=CARTESIAN_POINT('Ctrl Pts',(-16.7463694267337,40.8358142364,9.04598063092151));
#61965=CARTESIAN_POINT('Ctrl Pts',(-16.7889058330266,40.8312163164769,9.09060229381292));
#61966=CARTESIAN_POINT('Ctrl Pts',(-16.8339535664908,40.8266183965537,9.13300456901429));
#61967=CARTESIAN_POINT('Ctrl Pts',(-16.8812518847845,40.8220204766306,9.17289194291406));
#61968=CARTESIAN_POINT('Ctrl Pts',(-16.929361716829,40.817343668591,9.21346367840577));
#61969=CARTESIAN_POINT('Ctrl Pts',(-16.9797997930329,40.8126668605514,9.2514329514709));
#61970=CARTESIAN_POINT('Ctrl Pts',(-17.032250656482,40.8079900525118,9.28652603839862));
#61971=CARTESIAN_POINT('Ctrl Pts',(-17.0836748790441,40.8034047854314,9.32093223486302));
#61972=CARTESIAN_POINT('Ctrl Pts',(-17.1370333614423,40.7988195183511,9.35257352756306));
#61973=CARTESIAN_POINT('Ctrl Pts',(-17.1919955569535,40.7942342512708,9.38123255435389));
#61974=CARTESIAN_POINT('Ctrl Pts',(-17.2469241148445,40.789651790437,9.40987404142584));
#61975=CARTESIAN_POINT('Ctrl Pts',(-17.3034539893868,40.7850693296032,9.43553664692506));
#61976=CARTESIAN_POINT('Ctrl Pts',(-17.3612285269365,40.7804868687695,9.45804807853));
#61977=CARTESIAN_POINT('Ctrl Pts',(-17.418988908309,40.7759055307509,9.48055399428266));
#61978=CARTESIAN_POINT('Ctrl Pts',(-17.477992873332,40.7713241927323,9.49991008424874));
#61979=CARTESIAN_POINT('Ctrl Pts',(-17.5378641048536,40.7667428547137,9.51599231037787));
#61980=CARTESIAN_POINT('Ctrl Pts',(-17.5999022192742,40.7619957071275,9.53265659069048));
#61981=CARTESIAN_POINT('Ctrl Pts',(-17.662871036358,40.7572485595414,9.54580527134963));
#61982=CARTESIAN_POINT('Ctrl Pts',(-17.7263375990724,40.7525014119553,9.55535759468299));
#61983=CARTESIAN_POINT('Ctrl Pts',(-17.7876647122538,40.7479142900937,9.56458791044543));
#61984=CARTESIAN_POINT('Ctrl Pts',(-17.8494560127494,40.7433271682322,9.57046051341741));
#61985=CARTESIAN_POINT('Ctrl Pts',(-17.9113157728559,40.7387400463706,9.57295546405114));
#61986=CARTESIAN_POINT('Ctrl Pts',(-17.9764125800368,40.7339128859222,9.57558097245999));
#61987=CARTESIAN_POINT('Ctrl Pts',(-18.0415845644202,40.7290857254738,9.57446561933227));
#61988=CARTESIAN_POINT('Ctrl Pts',(-18.106373948019,40.7242585650253,9.56964833446866));
#61989=CARTESIAN_POINT('Ctrl Pts',(-18.1711633316178,40.7194314045769,9.56483104960505));
#61990=CARTESIAN_POINT('Ctrl Pts',(-18.2355694820098,40.7146042441284,9.55631199444223));
#61991=CARTESIAN_POINT('Ctrl Pts',(-18.2991476115092,40.70977708368,9.5441922343829));
#61992=CARTESIAN_POINT('Ctrl Pts',(-18.3597066094884,40.7051791503632,9.53264800477561));
#61993=CARTESIAN_POINT('Ctrl Pts',(-18.4197622963201,40.7005812170465,9.51779011094725));
#61994=CARTESIAN_POINT('Ctrl Pts',(-18.4789249876019,40.6959832837297,9.49967748108222));
#61995=CARTESIAN_POINT('Ctrl Pts',(-18.5391025569833,40.6913064773643,9.48125414676847));
#61996=CARTESIAN_POINT('Ctrl Pts',(-18.5983556664829,40.6866296709989,9.45946336625983));
#61997=CARTESIAN_POINT('Ctrl Pts',(-18.6562832944428,40.6819528646335,9.43442185527358));
#61998=CARTESIAN_POINT('Ctrl Pts',(-18.7130778238389,40.6773675393586,9.40987017100962));
#61999=CARTESIAN_POINT('Ctrl Pts',(-18.7685977698348,40.6727822140837,9.38219399544168));
#62000=CARTESIAN_POINT('Ctrl Pts',(-18.822481286114,40.6681968888088,9.35155327887583));
#62001=CARTESIAN_POINT('Ctrl Pts',(-18.8763320202996,40.6636143531915,9.3209312037593));
#62002=CARTESIAN_POINT('Ctrl Pts',(-18.9285478574583,40.6590318175742,9.28734841497482));
#62003=CARTESIAN_POINT('Ctrl Pts',(-18.9787906759488,40.6544492819569,9.25101123139448));
#62004=CARTESIAN_POINT('Ctrl Pts',(-19.0290213649992,40.6498678526389,9.214682820206));
#62005=CARTESIAN_POINT('Ctrl Pts',(-19.0772795688207,40.6452864233208,9.17560163236285));
#62006=CARTESIAN_POINT('Ctrl Pts',(-19.1232570588381,40.6407049940028,9.13401666643163));
#62007=CARTESIAN_POINT('Ctrl Pts',(-19.1708970425558,40.6359579054159,9.09092803547077));
#62008=CARTESIAN_POINT('Ctrl Pts',(-19.2160877418717,40.631210816829,9.0451514317453));
#62009=CARTESIAN_POINT('Ctrl Pts',(-19.2585266288888,40.6264637282421,8.99700687434557));
#62010=CARTESIAN_POINT('Ctrl Pts',(-19.2995365939041,40.621876474651,8.95048334949812));
#62011=CARTESIAN_POINT('Ctrl Pts',(-19.3379768509753,40.6172892210598,8.90174926454744));
#62012=CARTESIAN_POINT('Ctrl Pts',(-19.3736161279271,40.6127019674687,8.85112635454431));
#62013=CARTESIAN_POINT('Ctrl Pts',(-19.4111180892393,40.6078749613839,8.79785764162936));
#62014=CARTESIAN_POINT('Ctrl Pts',(-19.4455179006577,40.6030479552991,8.74249778810949));
#62015=CARTESIAN_POINT('Ctrl Pts',(-19.4766001645925,40.5982209492143,8.68545250195326));
#62016=CARTESIAN_POINT('Ctrl Pts',(-19.5076824285273,40.5933939431296,8.62840721579704));
#62017=CARTESIAN_POINT('Ctrl Pts',(-19.5354469380275,40.5885669370448,8.56967711579668));
#62018=CARTESIAN_POINT('Ctrl Pts',(-19.5597375386922,40.58373993096,8.50969066309164));
#62019=CARTESIAN_POINT('Ctrl Pts',(-19.5856975325918,40.578581184569,8.44558158782522));
#62020=CARTESIAN_POINT('Ctrl Pts',(-19.6077811078423,40.573422438178,8.37981635125834));
#62021=CARTESIAN_POINT('Ctrl Pts',(-19.625800376658,40.568263691787,8.3128498117788));
#62022=CARTESIAN_POINT('Ctrl Pts',(-19.6437505923802,40.5631247146442,8.24613990017688));
#62023=CARTESIAN_POINT('Ctrl Pts',(-19.6576674377672,40.5579857375013,8.17823812217481));
#62024=CARTESIAN_POINT('Ctrl Pts',(-19.6674119112357,40.5528467603585,8.10961610425827));
#62025=CARTESIAN_POINT('Ctrl Pts',(-19.6770963151771,40.5477394622928,8.04141710480199));
#62026=CARTESIAN_POINT('Ctrl Pts',(-19.6826595011998,40.5426321642272,7.97250698363599));
#62027=CARTESIAN_POINT('Ctrl Pts',(-19.6840133521854,40.5375248661615,7.90336661765679));
#62028=CARTESIAN_POINT('Ctrl Pts',(-19.6842245145942,40.5367282723164,7.89258267881568));
#62029=CARTESIAN_POINT('Ctrl Pts',(-19.6843333742035,40.5359316784714,7.88179316972827));
#62030=CARTESIAN_POINT('Ctrl Pts',(-19.6843397066618,40.5351350846263,7.8709999479683));
#62031=CARTESIAN_POINT('',(-19.6843394289759,39.7413850845213,7.86860485198167));
#62032=CARTESIAN_POINT('Ctrl Pts',(-19.6843397066623,40.5351350845702,7.870999947208));
#62033=CARTESIAN_POINT('Ctrl Pts',(-19.6843764767214,40.5305095784063,7.80832796688859));
#62034=CARTESIAN_POINT('Ctrl Pts',(-19.6809520465325,40.5258840722424,7.74564882250062));
#62035=CARTESIAN_POINT('Ctrl Pts',(-19.6740904775037,40.5212585660785,7.68336589370801));
#62036=CARTESIAN_POINT('Ctrl Pts',(-19.6672272265936,40.5166319261284,7.62106769836471));
#62037=CARTESIAN_POINT('Ctrl Pts',(-19.6569252202841,40.5120052861783,7.55916640317225));
#62038=CARTESIAN_POINT('Ctrl Pts',(-19.6432602041901,40.5073786462282,7.4980587025382));
#62039=CARTESIAN_POINT('Ctrl Pts',(-19.629576420193,40.5027456519256,7.4368670749337));
#62040=CARTESIAN_POINT('Ctrl Pts',(-19.612520516517,40.4981126576229,7.37647170126624));
#62041=CARTESIAN_POINT('Ctrl Pts',(-19.5922188435867,40.4934796633203,7.3172566273723));
#62042=CARTESIAN_POINT('Ctrl Pts',(-19.5719019880193,40.4888432042258,7.25799726939485));
#62043=CARTESIAN_POINT('Ctrl Pts',(-19.5483347177753,40.4842067451313,7.19992042690849));
#62044=CARTESIAN_POINT('Ctrl Pts',(-19.5216913956772,40.4795702860367,7.1433897357627));
#62045=CARTESIAN_POINT('Ctrl Pts',(-19.4949939983899,40.4749244168018,7.0867443101328));
#62046=CARTESIAN_POINT('Ctrl Pts',(-19.4652083192726,40.4702785475669,7.03165173711978));
#62047=CARTESIAN_POINT('Ctrl Pts',(-19.4325540921733,40.4656326783319,6.97844997621524));
#62048=CARTESIAN_POINT('Ctrl Pts',(-19.4139752396213,40.4629893783013,6.94818045955054));
#62049=CARTESIAN_POINT('Ctrl Pts',(-19.3944685912067,40.4603460782706,6.91852247669673));
#62050=CARTESIAN_POINT('Ctrl Pts',(-19.374080442917,40.45770277824,6.88953350170625));
#62051=CARTESIAN_POINT('Ctrl Pts',(-19.338621087469,40.4531055134953,6.83911546699063));
#62052=CARTESIAN_POINT('Ctrl Pts',(-19.3003502955231,40.4485082487506,6.79052003030235));
#62053=CARTESIAN_POINT('Ctrl Pts',(-19.2594821054512,40.4439109840059,6.74407798785612));
#62054=CARTESIAN_POINT('Ctrl Pts',(-19.2179060732883,40.439234094069,6.69683156350846));
#62055=CARTESIAN_POINT('Ctrl Pts',(-19.1736420396137,40.4345572041321,6.65181432598553));
#62056=CARTESIAN_POINT('Ctrl Pts',(-19.1269615127042,40.4298803141952,6.60934377248382));
#62057=CARTESIAN_POINT('Ctrl Pts',(-19.0812019895078,40.4252956989879,6.56771116019797));
#62058=CARTESIAN_POINT('Ctrl Pts',(-19.0331208560809,40.4207110837805,6.52852601220936));
#62059=CARTESIAN_POINT('Ctrl Pts',(-18.9830127669683,40.4161264685732,6.49205216902143));
#62060=CARTESIAN_POINT('Ctrl Pts',(-18.9329353153014,40.4115446565241,6.4556006269311));
#62061=CARTESIAN_POINT('Ctrl Pts',(-18.8808337760716,40.4069628444749,6.42185740148218));
#62062=CARTESIAN_POINT('Ctrl Pts',(-18.827035295064,40.4023810324258,6.39104562459966));
#62063=CARTESIAN_POINT('Ctrl Pts',(-18.7732499487917,40.3978003390121,6.36024137031863));
#62064=CARTESIAN_POINT('Ctrl Pts',(-18.7177689247181,40.3932196455984,6.33236739669762));
#62065=CARTESIAN_POINT('Ctrl Pts',(-18.6609459569101,40.3886389521846,6.30760202273307));
#62066=CARTESIAN_POINT('Ctrl Pts',(-18.6020503339371,40.3838911749626,6.28193331544677));
#62067=CARTESIAN_POINT('Ctrl Pts',(-18.5417134868834,40.3791433977405,6.25960465799173));
#62068=CARTESIAN_POINT('Ctrl Pts',(-18.4803519018833,40.3743956205185,6.2407600514713));
#62069=CARTESIAN_POINT('Ctrl Pts',(-18.4210747686482,40.3698091251898,6.22255559584208));
#62070=CARTESIAN_POINT('Ctrl Pts',(-18.3608419357492,40.3652226298612,6.20760232376056));
#62071=CARTESIAN_POINT('Ctrl Pts',(-18.3000417372015,40.3606361345325,6.19597845830795));
#62072=CARTESIAN_POINT('Ctrl Pts',(-18.2360345242219,40.3558077163638,6.1837414714322));
#62073=CARTESIAN_POINT('Ctrl Pts',(-18.17139907354,40.350979298195,6.17519494178607));
#62074=CARTESIAN_POINT('Ctrl Pts',(-18.1065943178466,40.3461508800263,6.1703680650538));
#62075=CARTESIAN_POINT('Ctrl Pts',(-18.0417895621532,40.3413224618575,6.16554118832153));
#62076=CARTESIAN_POINT('Ctrl Pts',(-17.976816152265,40.3364940436887,6.16443389803849));
#62077=CARTESIAN_POINT('Ctrl Pts',(-17.912129343232,40.33166562552,6.16701191737878));
#62078=CARTESIAN_POINT('Ctrl Pts',(-17.8505401687129,40.3270684241169,6.16946648401203));
#62079=CARTESIAN_POINT('Ctrl Pts',(-17.7889578794678,40.3224712227139,6.17527149008939));
#62080=CARTESIAN_POINT('Ctrl Pts',(-17.7277764699386,40.3178740213108,6.18442646957086));
#62081=CARTESIAN_POINT('Ctrl Pts',(-17.6655344279044,40.3131971234562,6.19374015851809));
#62082=CARTESIAN_POINT('Ctrl Pts',(-17.6037078310183,40.3085202256015,6.20652115043136));
#62083=CARTESIAN_POINT('Ctrl Pts',(-17.5427106807571,40.3038433277469,6.2227134776014));
#62084=CARTESIAN_POINT('Ctrl Pts',(-17.4829178855075,40.299258772655,6.23858609622287));
#62085=CARTESIAN_POINT('Ctrl Pts',(-17.4239225966,40.294674217563,6.25773642800875));
#62086=CARTESIAN_POINT('Ctrl Pts',(-17.36610626441,40.2900896624711,6.28005996433722));
#62087=CARTESIAN_POINT('Ctrl Pts',(-17.3083252657952,40.2855079091605,6.30236985797478));
#62088=CARTESIAN_POINT('Ctrl Pts',(-17.2517222691486,40.2809261558499,6.32784892791736));
#62089=CARTESIAN_POINT('Ctrl Pts',(-17.1966621383518,40.2763444025394,6.35634329185628));
#62090=CARTESIAN_POINT('Ctrl Pts',(-17.1416154327199,40.2717637663855,6.38483070809043));
#62091=CARTESIAN_POINT('Ctrl Pts',(-17.0881112980373,40.2671831302316,6.41633172495502));
#62092=CARTESIAN_POINT('Ctrl Pts',(-17.0364913621257,40.2626024940777,6.45064582085491));
#62093=CARTESIAN_POINT('Ctrl Pts',(-16.9829872339476,40.2578546589712,6.4862124242015));
#62094=CARTESIAN_POINT('Ctrl Pts',(-16.9315080360422,40.2531068238647,6.52480117070112));
#62095=CARTESIAN_POINT('Ctrl Pts',(-16.8824006114525,40.2483589887583,6.56614018473609));
#62096=CARTESIAN_POINT('Ctrl Pts',(-16.8349624902802,40.2437725463014,6.60607396610043));
#62097=CARTESIAN_POINT('Ctrl Pts',(-16.7897378088916,40.2391861038445,6.64857361098501));
#62098=CARTESIAN_POINT('Ctrl Pts',(-16.7470028516324,40.2345996613876,6.69335524999374));
#62099=CARTESIAN_POINT('Ctrl Pts',(-16.7020121892007,40.2297711299563,6.7405006254192));
#62100=CARTESIAN_POINT('Ctrl Pts',(-16.6597817923486,40.2249425985251,6.79017508808613));
#62101=CARTESIAN_POINT('Ctrl Pts',(-16.620585057557,40.2201140670938,6.84200882792571));
#62102=CARTESIAN_POINT('Ctrl Pts',(-16.5813883227654,40.2152855356625,6.89384256776529));
#62103=CARTESIAN_POINT('Ctrl Pts',(-16.5452255471153,40.2104570042313,6.94783500177105));
#62104=CARTESIAN_POINT('Ctrl Pts',(-16.5123147928673,40.2056284728,7.00358499068649));
#62105=CARTESIAN_POINT('Ctrl Pts',(-16.4809818950911,40.2010314380252,7.05666213047317));
#62106=CARTESIAN_POINT('Ctrl Pts',(-16.4524675419473,40.1964344032503,7.1115501949038));
#62107=CARTESIAN_POINT('Ctrl Pts',(-16.4269849961933,40.1918373684755,7.16791792961851));
#62108=CARTESIAN_POINT('Ctrl Pts',(-16.4010596333957,40.1871604497923,7.22526518160277));
#62109=CARTESIAN_POINT('Ctrl Pts',(-16.3782728046745,40.1824835311092,7.28414361158134));
#62110=CARTESIAN_POINT('Ctrl Pts',(-16.3588020123882,40.177806612426,7.34417500956728));
#62111=CARTESIAN_POINT('Ctrl Pts',(-16.3397164722956,40.173222232,7.4030186167629));
#62112=CARTESIAN_POINT('Ctrl Pts',(-16.3238171057571,40.1686378515739,7.46296947427151));
#62113=CARTESIAN_POINT('Ctrl Pts',(-16.3112229569419,40.1640534711478,7.52365044223742));
#62114=CARTESIAN_POINT('Ctrl Pts',(-16.2986365120407,40.1594718950138,7.5842942913029));
#62115=CARTESIAN_POINT('Ctrl Pts',(-16.2893513791435,40.1548903188799,7.64566686782294));
#62116=CARTESIAN_POINT('Ctrl Pts',(-16.2834361246219,40.1503087427459,7.70737819223101));
#62117=CARTESIAN_POINT('Ctrl Pts',(-16.2775223153285,40.1457282859929,7.76907443919016));
#62118=CARTESIAN_POINT('Ctrl Pts',(-16.2749767985288,40.1411478292399,7.83110876319327));
#62119=CARTESIAN_POINT('Ctrl Pts',(-16.2758163540269,40.1365673724869,7.89308541526515));
#62120=CARTESIAN_POINT('Ctrl Pts',(-16.2766866194582,40.1318193681197,7.95732909893502));
#62121=CARTESIAN_POINT('Ctrl Pts',(-16.2811944559054,40.1270713637524,8.02151022654404));
#62122=CARTESIAN_POINT('Ctrl Pts',(-16.2892995083944,40.1223233593852,8.08518987728147));
#62123=CARTESIAN_POINT('Ctrl Pts',(-16.2971284553907,40.1177370998168,8.14670022666516));
#62124=CARTESIAN_POINT('Ctrl Pts',(-16.3083132948938,40.1131508402485,8.20774221166161));
#62125=CARTESIAN_POINT('Ctrl Pts',(-16.3227653397069,40.1085645806801,8.26792978818296));
#62126=CARTESIAN_POINT('Ctrl Pts',(-16.3379819105069,40.1037357039134,8.33130134087745));
#62127=CARTESIAN_POINT('Ctrl Pts',(-16.3568207839431,40.0989068271467,8.39372495573301));
#62128=CARTESIAN_POINT('Ctrl Pts',(-16.3791194418188,40.09407795038,8.45477027458433));
#62129=CARTESIAN_POINT('Ctrl Pts',(-16.4014180996945,40.0892490736134,8.51581559343565));
#62130=CARTESIAN_POINT('Ctrl Pts',(-16.4271762130323,40.0844201968467,8.57548205017607));
#62131=CARTESIAN_POINT('Ctrl Pts',(-16.4561749107507,40.07959132008,8.63336880534534));
#62132=CARTESIAN_POINT('Ctrl Pts',(-16.4837819774528,40.0749941783639,8.68847760804556));
#62133=CARTESIAN_POINT('Ctrl Pts',(-16.5144390938614,40.0703970366478,8.7422000535105));
#62134=CARTESIAN_POINT('Ctrl Pts',(-16.5479835516064,40.0657998949317,8.79417732450549));
#62135=CARTESIAN_POINT('Ctrl Pts',(-16.5821100289745,40.0611229896162,8.84705643722659));
#62136=CARTESIAN_POINT('Ctrl Pts',(-16.6192248450111,40.0564460843007,8.89812872126577));
#62137=CARTESIAN_POINT('Ctrl Pts',(-16.6591064655308,40.0517691789852,8.94703997428014));
#62138=CARTESIAN_POINT('Ctrl Pts',(-16.6982000360492,40.0471846880499,8.99498475420501));
#62139=CARTESIAN_POINT('Ctrl Pts',(-16.7399517260247,40.0426001971145,9.04085271512015));
#62140=CARTESIAN_POINT('Ctrl Pts',(-16.78410918698,40.0380157061792,9.08433932610881));
#62141=CARTESIAN_POINT('Ctrl Pts',(-16.8282396470474,40.0334340185148,9.1277993464131));
#62142=CARTESIAN_POINT('Ctrl Pts',(-16.8747725992589,40.0288523308503,9.16888054760084));
#62143=CARTESIAN_POINT('Ctrl Pts',(-16.923417536701,40.0242706431859,9.20731385016716));
#62144=CARTESIAN_POINT('Ctrl Pts',(-16.9720505983018,40.0196900740633,9.2457377698907));
#62145=CARTESIAN_POINT('Ctrl Pts',(-17.0227942223191,40.0151095049406,9.28151475881925));
#62146=CARTESIAN_POINT('Ctrl Pts',(-17.0753249742169,40.010528935818,9.31441612194144));
#62147=CARTESIAN_POINT('Ctrl Pts',(-17.1297746751559,40.0057810384465,9.34851937228089));
#62148=CARTESIAN_POINT('Ctrl Pts',(-17.1861441389438,40.001033141075,9.37953247427002));
#62149=CARTESIAN_POINT('Ctrl Pts',(-17.24404273101,39.9962852437035,9.40725135674708));
#62150=CARTESIAN_POINT('Ctrl Pts',(-17.2999715986737,39.9916988709733,9.43402723599598));
#62151=CARTESIAN_POINT('Ctrl Pts',(-17.3573267010973,39.987112498243,9.45772931458685));
#62152=CARTESIAN_POINT('Ctrl Pts',(-17.4157355711229,39.9825261255128,9.47822277371764));
#62153=CARTESIAN_POINT('Ctrl Pts',(-17.4772300402698,39.9776974658207,9.49979885265356));
#62154=CARTESIAN_POINT('Ctrl Pts',(-17.5398920824226,39.9728688061285,9.51781771632805));
#62155=CARTESIAN_POINT('Ctrl Pts',(-17.6032720539256,39.9680401464364,9.53218256826576));
#62156=CARTESIAN_POINT('Ctrl Pts',(-17.6666520254286,39.9632114867443,9.54654742020348));
#62157=CARTESIAN_POINT('Ctrl Pts',(-17.7307492725042,39.9583828270522,9.55725822984731));
#62158=CARTESIAN_POINT('Ctrl Pts',(-17.795108396834,39.95355416736,9.56428153819804));
#62159=CARTESIAN_POINT('Ctrl Pts',(-17.8563815022406,39.9489570418185,9.57096807903211));
#62160=CARTESIAN_POINT('Ctrl Pts',(-17.9181436440668,39.9443599162769,9.57434018552573));
#62161=CARTESIAN_POINT('Ctrl Pts',(-17.9800051116147,39.9397627907354,9.57433999999233));
#62162=CARTESIAN_POINT('Ctrl Pts',(-18.042940167196,39.9350858833981,9.57433981123906));
#62163=CARTESIAN_POINT('Ctrl Pts',(-18.1059775118455,39.9304089760608,9.57084901194266));
#62164=CARTESIAN_POINT('Ctrl Pts',(-18.168699409273,39.9257320687235,9.56386167337833));
#62165=CARTESIAN_POINT('Ctrl Pts',(-18.2301816966983,39.9211475938755,9.55701242972387));
#62166=CARTESIAN_POINT('Ctrl Pts',(-18.2913603616633,39.9165631190275,9.54680365645155));
#62167=CARTESIAN_POINT('Ctrl Pts',(-18.3518426985217,39.9119786441795,9.53328224999732));
#62168=CARTESIAN_POINT('Ctrl Pts',(-18.4122880532494,39.9073969725243,9.51976911125306));
#62169=CARTESIAN_POINT('Ctrl Pts',(-18.4720374283351,39.9028153008691,9.5029474664673));
#62170=CARTESIAN_POINT('Ctrl Pts',(-18.5307072137617,39.8982336292138,9.4829154969529));
#62171=CARTESIAN_POINT('Ctrl Pts',(-18.5893626772443,39.8936530759954,9.46288841746398));
#62172=CARTESIAN_POINT('Ctrl Pts',(-18.6469385926822,39.8890725227769,9.43965273337322));
#62173=CARTESIAN_POINT('Ctrl Pts',(-18.7030674270037,39.8844919695584,9.41335619077589));
#62174=CARTESIAN_POINT('Ctrl Pts',(-18.7612470407707,39.8797440566485,9.38609885129586));
#62175=CARTESIAN_POINT('Ctrl Pts',(-18.8178712281102,39.8749961437387,9.3555528437369));
#62176=CARTESIAN_POINT('Ctrl Pts',(-18.8725566990867,39.8702482308288,9.32193573360373));
#62177=CARTESIAN_POINT('Ctrl Pts',(-18.9253814059612,39.8656618735524,9.28946250155435));
#62178=CARTESIAN_POINT('Ctrl Pts',(-18.9763968279962,39.8610755162759,9.25412418089979));
#62179=CARTESIAN_POINT('Ctrl Pts',(-19.0252877213073,39.8564891589995,9.21616062016546));
#62180=CARTESIAN_POINT('Ctrl Pts',(-19.0767619063556,39.8516604682729,9.17619114491172));
#62181=CARTESIAN_POINT('Ctrl Pts',(-19.1258803315661,39.8468317775464,9.13331172815551));
#62182=CARTESIAN_POINT('Ctrl Pts',(-19.1723178427938,39.8420030868198,9.08784769054079));
#62183=CARTESIAN_POINT('Ctrl Pts',(-19.2187553540215,39.8371743960932,9.04238365292608));
#62184=CARTESIAN_POINT('Ctrl Pts',(-19.2625115710664,39.8323457053667,8.99433552723391));
#62185=CARTESIAN_POINT('Ctrl Pts',(-19.3033114389676,39.8275170146401,8.94406781494346));
#62186=CARTESIAN_POINT('Ctrl Pts',(-19.3420164456719,39.8229362520896,8.89638108845889));
#62187=CARTESIAN_POINT('Ctrl Pts',(-19.3782245727256,39.8183554895392,8.84649586219358));
#62188=CARTESIAN_POINT('Ctrl Pts',(-19.4116758245007,39.8137747269888,8.79470490922245));
#62189=CARTESIAN_POINT('Ctrl Pts',(-19.4450771820822,39.8092007968718,8.7429912050149));
#62190=CARTESIAN_POINT('Ctrl Pts',(-19.4757295390519,39.8046268667549,8.68937783439572));
#62191=CARTESIAN_POINT('Ctrl Pts',(-19.5034132813638,39.800052936638,8.63419029682698));
#62192=CARTESIAN_POINT('Ctrl Pts',(-19.5310660730067,39.7954841202154,8.57906445941373));
#62193=CARTESIAN_POINT('Ctrl Pts',(-19.5557566030015,39.7909153037929,8.52236840080617));
#62194=CARTESIAN_POINT('Ctrl Pts',(-19.5773098418524,39.7863464873703,8.46445445975392));
#62195=CARTESIAN_POINT('Ctrl Pts',(-19.5988492724775,39.7817805979904,8.40657762165346));
#62196=CARTESIAN_POINT('Ctrl Pts',(-19.6172552172746,39.7772147086105,8.34748492686722));
#62197=CARTESIAN_POINT('Ctrl Pts',(-19.6324005160062,39.7726488192305,8.28754924296698));
#62198=CARTESIAN_POINT('Ctrl Pts',(-19.6475403841638,39.7680845670188,8.22763504990537));
#62199=CARTESIAN_POINT('Ctrl Pts',(-19.6594218054773,39.763520314807,8.16687896538041));
#62200=CARTESIAN_POINT('Ctrl Pts',(-19.6679679164472,39.7589560625952,8.10566745351237));
#62201=CARTESIAN_POINT('Ctrl Pts',(-19.6765164524315,39.7543905152473,8.04443857248084));
#62202=CARTESIAN_POINT('Ctrl Pts',(-19.6817277211054,39.7498249678993,7.98275451434472));
#62203=CARTESIAN_POINT('Ctrl Pts',(-19.683576521035,39.7452594205514,7.92100855397197));
#62204=CARTESIAN_POINT('Ctrl Pts',(-19.6840994865959,39.7439679752243,7.9035426236221));
#62205=CARTESIAN_POINT('Ctrl Pts',(-19.6843537271266,39.7426765298973,7.88607175389086));
#62206=CARTESIAN_POINT('Ctrl Pts',(-19.6843394289765,39.7413850845702,7.86860485264345));
#62207=CARTESIAN_POINT('',(-19.6843399884914,38.9476350846074,7.8698019364786));
#62208=CARTESIAN_POINT('Ctrl Pts',(-19.6843394289759,39.7413850845213,7.86860485198167));
#62209=CARTESIAN_POINT('Ctrl Pts',(-19.684279410828,39.7359640951663,7.79528553776752));
#62210=CARTESIAN_POINT('Ctrl Pts',(-19.6794842803753,39.7305431058113,7.72216833145521));
#62211=CARTESIAN_POINT('Ctrl Pts',(-19.6700551719018,39.7251221164563,7.64979929262621));
#62212=CARTESIAN_POINT('Ctrl Pts',(-19.6605095703009,39.7196341527945,7.57653616124495));
#62213=CARTESIAN_POINT('Ctrl Pts',(-19.6462148775261,39.7141461891327,7.5040398728715));
#62214=CARTESIAN_POINT('Ctrl Pts',(-19.6273250408721,39.7086582254709,7.43285580718068));
#62215=CARTESIAN_POINT('Ctrl Pts',(-19.6190889492313,39.7062654376206,7.40181909155751));
#62216=CARTESIAN_POINT('Ctrl Pts',(-19.6099799283487,39.7038726497703,7.37103155567359));
#62217=CARTESIAN_POINT('Ctrl Pts',(-19.600013546114,39.70147986192,7.34053711555268));
#62218=CARTESIAN_POINT('Ctrl Pts',(-19.5808657271779,39.6968827405744,7.28194995681868));
#62219=CARTESIAN_POINT('Ctrl Pts',(-19.558496309674,39.6922856192287,7.22428251621042));
#62220=CARTESIAN_POINT('Ctrl Pts',(-19.5330131080486,39.6876884978831,7.16791373619111));
#62221=CARTESIAN_POINT('Ctrl Pts',(-19.5070876261949,39.6830115900213,7.11056663338234));
#62222=CARTESIAN_POINT('Ctrl Pts',(-19.4779393198059,39.6783346821595,7.05456423330453));
#62223=CARTESIAN_POINT('Ctrl Pts',(-19.4457348669613,39.6736577742977,7.00028962557989));
#62224=CARTESIAN_POINT('Ctrl Pts',(-19.4141669253492,39.6690733040998,6.94708773899801));
#62225=CARTESIAN_POINT('Ctrl Pts',(-19.3796628177758,39.6644888339019,6.89554642685218));
#62226=CARTESIAN_POINT('Ctrl Pts',(-19.3424270458154,39.659904363704,6.84600420878273));
#62227=CARTESIAN_POINT('Ctrl Pts',(-19.3052140430898,39.6553226968554,6.79649228519452));
#62228=CARTESIAN_POINT('Ctrl Pts',(-19.2652729933165,39.6507410300069,6.74897743790462));
#62229=CARTESIAN_POINT('Ctrl Pts',(-19.2228513827234,39.6461593631584,6.70376877247154));
#62230=CARTESIAN_POINT('Ctrl Pts',(-19.1804401291069,39.6415788148957,6.65857114445736));
#62231=CARTESIAN_POINT('Ctrl Pts',(-19.1355498650892,39.6369982666331,6.61567895164971));
#62232=CARTESIAN_POINT('Ctrl Pts',(-19.0884666183234,39.6324177183705,6.57536623261146));
#62233=CARTESIAN_POINT('Ctrl Pts',(-19.0396629915074,39.6276698009396,6.5335805225973));
#62234=CARTESIAN_POINT('Ctrl Pts',(-18.9885034211213,39.6229218835088,6.49456686603282));
#62235=CARTESIAN_POINT('Ctrl Pts',(-18.9353440481846,39.6181739660779,6.45858489975546));
#62236=CARTESIAN_POINT('Ctrl Pts',(-18.8839936192567,39.6135876140741,6.42382735278048));
#62237=CARTESIAN_POINT('Ctrl Pts',(-18.8307778008058,39.6090012620703,6.39189867932567));
#62238=CARTESIAN_POINT('Ctrl Pts',(-18.7760450056889,39.6044149100665,6.36298733100289));
#62239=CARTESIAN_POINT('Ctrl Pts',(-18.7184200664199,39.5995862099221,6.33254827362012));
#62240=CARTESIAN_POINT('Ctrl Pts',(-18.659113969525,39.5947575097777,6.30545454127591));
#62241=CARTESIAN_POINT('Ctrl Pts',(-18.5985570975186,39.5899288096332,6.2818684082516));
#62242=CARTESIAN_POINT('Ctrl Pts',(-18.5380002255122,39.5851001094888,6.25828227522728));
#62243=CARTESIAN_POINT('Ctrl Pts',(-18.4761932205006,39.5802714093444,6.23820386849679));
#62244=CARTESIAN_POINT('Ctrl Pts',(-18.4135815295858,39.5754427092,6.22173367054894));
#62245=CARTESIAN_POINT('Ctrl Pts',(-18.3539726614825,39.5708455909013,6.2060533743812));
#62246=CARTESIAN_POINT('Ctrl Pts',(-18.2933896582679,39.5662484726026,6.19357863723256));
#62247=CARTESIAN_POINT('Ctrl Pts',(-18.2322093762423,39.5616513543039,6.18442435170193));
#62248=CARTESIAN_POINT('Ctrl Pts',(-18.1699672178508,39.5569744460612,6.17511117969463));
#62249=CARTESIAN_POINT('Ctrl Pts',(-18.1071073384429,39.5522975378185,6.16923504833745));
#62250=CARTESIAN_POINT('Ctrl Pts',(-18.0440419983898,39.5476206295759,6.16686364079612));
#62251=CARTESIAN_POINT('Ctrl Pts',(-17.982223172164,39.5430361624552,6.16453910515444));
#62252=CARTESIAN_POINT('Ctrl Pts',(-17.9202074668202,39.5384516953346,6.16558202959813));
#62253=CARTESIAN_POINT('Ctrl Pts',(-17.8583902029577,39.5338672282139,6.1700041491629));
#62254=CARTESIAN_POINT('Ctrl Pts',(-17.7966107396829,39.5292855644453,6.17442356464944));
#62255=CARTESIAN_POINT('Ctrl Pts',(-17.7350299840039,39.5247039006766,6.1822180417638));
#62256=CARTESIAN_POINT('Ctrl Pts',(-17.6740418505353,39.520122236908,6.19334724931603));
#62257=CARTESIAN_POINT('Ctrl Pts',(-17.613068606923,39.5155416917228,6.20447373974457));
#62258=CARTESIAN_POINT('Ctrl Pts',(-17.5526881988819,39.5109611465375,6.21893325305502));
#62259=CARTESIAN_POINT('Ctrl Pts',(-17.4932859760176,39.5063806013523,6.23663405984485));
#62260=CARTESIAN_POINT('Ctrl Pts',(-17.4317131686996,39.5016326809463,6.25498166222892));
#62261=CARTESIAN_POINT('Ctrl Pts',(-17.3711919934313,39.4968847605403,6.27681191536764));
#62262=CARTESIAN_POINT('Ctrl Pts',(-17.3121337194731,39.4921368401342,6.30196636932268));
#62263=CARTESIAN_POINT('Ctrl Pts',(-17.2550851949196,39.4875504911655,6.3262648187677));
#62264=CARTESIAN_POINT('Ctrl Pts',(-17.1994020424159,39.4829641421968,6.35366454761002));
#62265=CARTESIAN_POINT('Ctrl Pts',(-17.1454315278639,39.4783777932282,6.38397499990192));
#62266=CARTESIAN_POINT('Ctrl Pts',(-17.0886090409689,39.4735490871035,6.41588715216574));
#62267=CARTESIAN_POINT('Ctrl Pts',(-17.0336857643878,39.4687203809788,6.45102584457634));
#62268=CARTESIAN_POINT('Ctrl Pts',(-16.9810314190361,39.4638916748541,6.48911745255183));
#62269=CARTESIAN_POINT('Ctrl Pts',(-16.9283770736844,39.4590629687294,6.52720906052732));
#62270=CARTESIAN_POINT('Ctrl Pts',(-16.8779921144322,39.4542342626047,6.56825311340285));
#62271=CARTESIAN_POINT('Ctrl Pts',(-16.8302025118619,39.44940555648,6.61192982235833));
#62272=CARTESIAN_POINT('Ctrl Pts',(-16.7847049478526,39.4448084400745,6.65351175136677));
#62273=CARTESIAN_POINT('Ctrl Pts',(-16.7413725326871,39.4402113236689,6.69765036902677));
#62274=CARTESIAN_POINT('Ctrl Pts',(-16.7005061503624,39.4356142072634,6.74409133392642));
#62275=CARTESIAN_POINT('Ctrl Pts',(-16.6589304509126,39.4309372987841,6.79133837388919));
#62276=CARTESIAN_POINT('Ctrl Pts',(-16.619907662227,39.4262603903048,6.84096815918623));
#62277=CARTESIAN_POINT('Ctrl Pts',(-16.5837182001836,39.4215834818255,6.89267100160617));
#62278=CARTESIAN_POINT('Ctrl Pts',(-16.5482440558587,39.4169990167072,6.94335189019769));
#62279=CARTESIAN_POINT('Ctrl Pts',(-16.5154925571735,39.4124145515888,6.99602419278973));
#62280=CARTESIAN_POINT('Ctrl Pts',(-16.4856879253843,39.4078300864705,7.05036211699453));
#62281=CARTESIAN_POINT('Ctrl Pts',(-16.4559015190412,39.4032484247394,7.10466681371581));
#62282=CARTESIAN_POINT('Ctrl Pts',(-16.4290586508097,39.3986667630082,7.16063466705732));
#62283=CARTESIAN_POINT('Ctrl Pts',(-16.4053390325209,39.394085101277,7.21791283320578));
#62284=CARTESIAN_POINT('Ctrl Pts',(-16.3816252053903,39.3895045581612,7.27517701485755));
#62285=CARTESIAN_POINT('Ctrl Pts',(-16.3610333091326,39.3849240150453,7.33375040411154));
#62286=CARTESIAN_POINT('Ctrl Pts',(-16.3436952254678,39.3803434719295,7.39325948311146));
#62287=CARTESIAN_POINT('Ctrl Pts',(-16.3257235848103,39.375595549582,7.45494310422659));
#62288=CARTESIAN_POINT('Ctrl Pts',(-16.3112483819578,39.3708476272346,7.51763158045874));
#62289=CARTESIAN_POINT('Ctrl Pts',(-16.3003594938038,39.3660997048871,7.5808934356591));
#62290=CARTESIAN_POINT('Ctrl Pts',(-16.2898411630142,39.3615133580437,7.64200244054137));
#62291=CARTESIAN_POINT('Ctrl Pts',(-16.282668953038,39.3569270112002,7.70364589102187));
#62292=CARTESIAN_POINT('Ctrl Pts',(-16.2788710588162,39.3523406643567,7.76542867952014));
#62293=CARTESIAN_POINT('Ctrl Pts',(-16.2748724667317,39.3475119542573,7.83047634926123));
#62294=CARTESIAN_POINT('Ctrl Pts',(-16.2746147232969,39.3426832441578,7.8956778461991));
#62295=CARTESIAN_POINT('Ctrl Pts',(-16.2780684035736,39.3378545340584,7.96057415020563));
#62296=CARTESIAN_POINT('Ctrl Pts',(-16.2815220838503,39.333025823959,8.02547045421216));
#62297=CARTESIAN_POINT('Ctrl Pts',(-16.2886870390274,39.3281971138595,8.0900609278755));
#62298=CARTESIAN_POINT('Ctrl Pts',(-16.2994713322898,39.3233684037601,8.1538982786211));
#62299=CARTESIAN_POINT('Ctrl Pts',(-16.3097383953178,39.3187712855504,8.21467389809844));
#62300=CARTESIAN_POINT('Ctrl Pts',(-16.3233276849758,39.3141741673408,8.27501667102926));
#62301=CARTESIAN_POINT('Ctrl Pts',(-16.3401886515697,39.3095770491311,8.33453587284437));
#62302=CARTESIAN_POINT('Ctrl Pts',(-16.3573422661242,39.3049001408773,8.39508812178211));
#62303=CARTESIAN_POINT('Ctrl Pts',(-16.3778822159995,39.3002232326235,8.45478739934842));
#62304=CARTESIAN_POINT('Ctrl Pts',(-16.4017003494219,39.2955463243697,8.51323016765784));
#62305=CARTESIAN_POINT('Ctrl Pts',(-16.4250477063735,39.29096185738,8.57051778750443));
#62306=CARTESIAN_POINT('Ctrl Pts',(-16.4515446352578,39.2863773903903,8.62659762266767));
#62307=CARTESIAN_POINT('Ctrl Pts',(-16.4810389818213,39.2817929234006,8.6811046181478));
#62308=CARTESIAN_POINT('Ctrl Pts',(-16.5105152928122,39.2772112597782,8.73557828300733));
#62309=CARTESIAN_POINT('Ctrl Pts',(-16.5429851453509,39.2726295961559,8.78848056844859));
#62310=CARTESIAN_POINT('Ctrl Pts',(-16.5782495209855,39.2680479325335,8.83946914864923));
#62311=CARTESIAN_POINT('Ctrl Pts',(-16.6135052869354,39.2634673875097,8.89044528015084));
#62312=CARTESIAN_POINT('Ctrl Pts',(-16.651553932126,39.2588868424858,8.93950821541387));
#62313=CARTESIAN_POINT('Ctrl Pts',(-16.6921531316782,39.254306297462,8.9863446060038));
#62314=CARTESIAN_POINT('Ctrl Pts',(-16.7342358472203,39.2495583769268,9.03489242280685));
#62315=CARTESIAN_POINT('Ctrl Pts',(-16.7790587895914,39.2448104563917,9.08104734483284));
#62316=CARTESIAN_POINT('Ctrl Pts',(-16.8263081600114,39.2400625358565,9.12449988997354));
#62317=CARTESIAN_POINT('Ctrl Pts',(-16.871949634076,39.2354761870853,9.16647374474567));
#62318=CARTESIAN_POINT('Ctrl Pts',(-16.9198545831394,39.230889838314,9.20592592255711));
#62319=CARTESIAN_POINT('Ctrl Pts',(-16.9697063184792,39.2263034895428,9.24261848766481));
#62320=CARTESIAN_POINT('Ctrl Pts',(-17.0221923823066,39.2214747831257,9.28125000773333));
#62321=CARTESIAN_POINT('Ctrl Pts',(-17.0768361526629,39.2166460767085,9.3168218107131));
#62322=CARTESIAN_POINT('Ctrl Pts',(-17.1332359974883,39.2118173702914,9.34910971859778));
#62323=CARTESIAN_POINT('Ctrl Pts',(-17.1896358423137,39.2069886638743,9.38139762648245));
#62324=CARTESIAN_POINT('Ctrl Pts',(-17.2477911453543,39.2021599574571,9.41040141867307));
#62325=CARTESIAN_POINT('Ctrl Pts',(-17.307276231525,39.19733125104,9.43595579980049));
#62326=CARTESIAN_POINT('Ctrl Pts',(-17.3639083642674,39.1927341333355,9.46028457188976));
#62327=CARTESIAN_POINT('Ctrl Pts',(-17.4219782762463,39.188137015631,9.48158723566076));
#62328=CARTESIAN_POINT('Ctrl Pts',(-17.4811302627633,39.1835398979265,9.49969439493097));
#62329=CARTESIAN_POINT('Ctrl Pts',(-17.5413089302432,39.1788629896096,9.51811583402182));
#62330=CARTESIAN_POINT('Ctrl Pts',(-17.6026071429664,39.1741860812926,9.53322948742616));
#62331=CARTESIAN_POINT('Ctrl Pts',(-17.6646271955617,39.1695091729757,9.54490740932767));
#62332=CARTESIAN_POINT('Ctrl Pts',(-17.7254213853687,39.1649247065002,9.55635451023976));
#62333=CARTESIAN_POINT('Ctrl Pts',(-17.786908615016,39.1603402400248,9.56450036319615));
#62334=CARTESIAN_POINT('Ctrl Pts',(-17.8486996531526,39.1557557735493,9.56927486137992));
#62335=CARTESIAN_POINT('Ctrl Pts',(-17.9104529065007,39.1511741104431,9.57404643999138));
#62336=CARTESIAN_POINT('Ctrl Pts',(-17.9725090934622,39.1465924473369,9.57545071245706));
#62337=CARTESIAN_POINT('Ctrl Pts',(-18.0344726682356,39.1420107842307,9.5734692729883));
#62338=CARTESIAN_POINT('Ctrl Pts',(-18.0964211147838,39.1374302397241,9.57148831728218));
#62339=CARTESIAN_POINT('Ctrl Pts',(-18.1582764854426,39.1328496952175,9.56612330684676));
#62340=CARTESIAN_POINT('Ctrl Pts',(-18.2196440990188,39.1282691507109,9.55740793568285));
#62341=CARTESIAN_POINT('Ctrl Pts',(-18.2832541311443,39.1235212296783,9.54837409833094));
#62342=CARTESIAN_POINT('Ctrl Pts',(-18.3463394845881,39.1187733086458,9.53574032947628));
#62343=CARTESIAN_POINT('Ctrl Pts',(-18.4084699699796,39.1140253876132,9.51960247345403));
#62344=CARTESIAN_POINT('Ctrl Pts',(-18.4684861415732,39.1094390393559,9.50401379214759));
#62345=CARTESIAN_POINT('Ctrl Pts',(-18.5276109124083,39.1048526910985,9.48515592536526));
#62346=CARTESIAN_POINT('Ctrl Pts',(-18.5854726409809,39.1002663428412,9.46316594133305));
#62347=CARTESIAN_POINT('Ctrl Pts',(-18.6463919917205,39.095437635421,9.44001392733237));
#62348=CARTESIAN_POINT('Ctrl Pts',(-18.705910516523,39.0906089280008,9.41338984409157));
#62349=CARTESIAN_POINT('Ctrl Pts',(-18.7636220728151,39.0857802205807,9.38350959118104));
#62350=CARTESIAN_POINT('Ctrl Pts',(-18.8213336291072,39.0809515131605,9.35362933827051));
#62351=CARTESIAN_POINT('Ctrl Pts',(-18.877237697375,39.0761228057403,9.32049331386066));
#62352=CARTESIAN_POINT('Ctrl Pts',(-18.9309645721965,39.0712940983201,9.28436954790013));
#62353=CARTESIAN_POINT('Ctrl Pts',(-18.9819503591381,39.066711746405,9.2500887779705));
#62354=CARTESIAN_POINT('Ctrl Pts',(-19.0311881697655,39.06212939449,9.21297482694768));
#62355=CARTESIAN_POINT('Ctrl Pts',(-19.0783440253598,39.0575470425749,9.17323261068636));
#62356=CARTESIAN_POINT('Ctrl Pts',(-19.125472229701,39.0529673776596,9.13351369846791));
#62357=CARTESIAN_POINT('Ctrl Pts',(-19.170520476064,39.0483877127443,9.09116986210096));
#62358=CARTESIAN_POINT('Ctrl Pts',(-19.2131832258037,39.043808047829,9.0464497299912));
#62359=CARTESIAN_POINT('Ctrl Pts',(-19.2557543917755,39.039238214042,9.00182559821491));
#62360=CARTESIAN_POINT('Ctrl Pts',(-19.2959499050033,39.0346683802551,8.95483569878509));
#62361=CARTESIAN_POINT('Ctrl Pts',(-19.3335001504166,39.0300985464681,8.90576646905679));
#62362=CARTESIAN_POINT('Ctrl Pts',(-19.3710276077472,39.0255314859719,8.85672701792641));
#62363=CARTESIAN_POINT('Ctrl Pts',(-19.4059126688167,39.0209644254758,8.80561114451897));
#62364=CARTESIAN_POINT('Ctrl Pts',(-19.4379256173855,39.0163973649796,8.75273876643729));
#62365=CARTESIAN_POINT('Ctrl Pts',(-19.4699310998572,39.0118313696186,8.69987871931291));
#62366=CARTESIAN_POINT('Ctrl Pts',(-19.4990655340768,39.0072653742576,8.64526341917988));
#62367=CARTESIAN_POINT('Ctrl Pts',(-19.5251433765955,39.0026993788966,8.58924041972287));
#62368=CARTESIAN_POINT('Ctrl Pts',(-19.5513508421705,38.9981106877058,8.53293895120119));
#62369=CARTESIAN_POINT('Ctrl Pts',(-19.5744710062061,38.993521996515,8.47521621476008));
#62370=CARTESIAN_POINT('Ctrl Pts',(-19.5943640075944,38.9889333053243,8.41644641693734));
#62371=CARTESIAN_POINT('Ctrl Pts',(-19.6141837333932,38.9843615165127,8.35789309683448));
#62372=CARTESIAN_POINT('Ctrl Pts',(-19.6307999302125,38.9797897277011,8.29830092486713));
#62373=CARTESIAN_POINT('Ctrl Pts',(-19.6441247463646,38.9752179388895,8.2380538875451));
#62374=CARTESIAN_POINT('Ctrl Pts',(-19.6575234573653,38.9706207965091,8.17747274086993));
#62375=CARTESIAN_POINT('Ctrl Pts',(-19.6675940856779,38.9660236541288,8.11622996014002));
#62376=CARTESIAN_POINT('Ctrl Pts',(-19.6742999999685,38.9614265117484,8.05472234761063));
#62377=CARTESIAN_POINT('Ctrl Pts',(-19.6810059142591,38.9568293693681,7.99321473508123));
#62378=CARTESIAN_POINT('Ctrl Pts',(-19.6843471518562,38.9522322269878,7.93144281335181));
#62379=CARTESIAN_POINT('Ctrl Pts',(-19.6843399884914,38.9476350846074,7.8698019364786));
#62380=CARTESIAN_POINT('',(-19.6843393239652,38.1538850846314,7.87151802034673));
#62381=CARTESIAN_POINT('Ctrl Pts',(-19.6843399884913,38.9476350845702,7.86980193597941));
#62382=CARTESIAN_POINT('Ctrl Pts',(-19.684338753266,38.9468423715801,7.85917282777021));
#62383=CARTESIAN_POINT('Ctrl Pts',(-19.6842380866645,38.9460496585901,7.84854438188443));
#62384=CARTESIAN_POINT('Ctrl Pts',(-19.6840380186188,38.9452569456001,7.83791781332828));
#62385=CARTESIAN_POINT('Ctrl Pts',(-19.6828777798244,38.94065982785,7.77629199471976));
#62386=CARTESIAN_POINT('Ctrl Pts',(-19.678367839255,38.9360627100999,7.71460262236847));
#62387=CARTESIAN_POINT('Ctrl Pts',(-19.6705003692328,38.9314655923497,7.65324359934786));
#62388=CARTESIAN_POINT('Ctrl Pts',(-19.6624963462916,38.9267886840385,7.59081958927602));
#62389=CARTESIAN_POINT('Ctrl Pts',(-19.6510170464113,38.9221117757273,7.52873803761941));
#62390=CARTESIAN_POINT('Ctrl Pts',(-19.6361097136432,38.917434867416,7.46741404398989));
#62391=CARTESIAN_POINT('Ctrl Pts',(-19.6214970329153,38.9128504008982,7.40730215450473));
#62392=CARTESIAN_POINT('Ctrl Pts',(-19.6035907260735,38.9082659343803,7.34791866715934));
#62393=CARTESIAN_POINT('Ctrl Pts',(-19.5824872499946,38.9036814678624,7.2896471338876));
#62394=CARTESIAN_POINT('Ctrl Pts',(-19.5613966785499,38.8990998047151,7.23141123326809));
#62395=CARTESIAN_POINT('Ctrl Pts',(-19.5371129874217,38.8945181415678,7.17428641613707));
#62396=CARTESIAN_POINT('Ctrl Pts',(-19.5097823452457,38.8899364784205,7.11864069063157));
#62397=CARTESIAN_POINT('Ctrl Pts',(-19.4824583757741,38.8853559338742,7.06300855088364));
#62398=CARTESIAN_POINT('Ctrl Pts',(-19.4520891563378,38.8807753893279,7.00885524262533));
#62399=CARTESIAN_POINT('Ctrl Pts',(-19.4188679733629,38.8761948447816,6.95652652428732));
#62400=CARTESIAN_POINT('Ctrl Pts',(-19.3844328640819,38.8714469237898,6.90228567633601));
#62401=CARTESIAN_POINT('Ctrl Pts',(-19.3469335888698,38.866699002798,6.8500058692463));
#62402=CARTESIAN_POINT('Ctrl Pts',(-19.3066346934272,38.8619510818062,6.80003961484771));
#62403=CARTESIAN_POINT('Ctrl Pts',(-19.2677071774373,38.8573647335131,6.7517737220559));
#62404=CARTESIAN_POINT('Ctrl Pts',(-19.2261679418072,38.85277838522,6.70566678501357));
#62405=CARTESIAN_POINT('Ctrl Pts',(-19.1822949778855,38.8481920369269,6.66200098437487));
#62406=CARTESIAN_POINT('Ctrl Pts',(-19.1361036096275,38.8433633295858,6.61602772664873));
#62407=CARTESIAN_POINT('Ctrl Pts',(-19.0873255031391,38.8385346222446,6.5727611943697));
#62408=CARTESIAN_POINT('Ctrl Pts',(-19.0363246941023,38.8337059149035,6.53248253236469));
#62409=CARTESIAN_POINT('Ctrl Pts',(-18.9853238850656,38.8288772075624,6.49220387035968));
#62410=CARTESIAN_POINT('Ctrl Pts',(-18.9321009503056,38.8240485002212,6.45491338799462));
#62411=CARTESIAN_POINT('Ctrl Pts',(-18.8770524174963,38.8192197928801,6.42083755366625));
#62412=CARTESIAN_POINT('Ctrl Pts',(-18.8246440677802,38.8146226752078,6.38839603068258));
#62413=CARTESIAN_POINT('Ctrl Pts',(-18.7703659552456,38.8100255575355,6.35873453058484));
#62414=CARTESIAN_POINT('Ctrl Pts',(-18.714544800395,38.8054284398633,6.33207322287024));
#62415=CARTESIAN_POINT('Ctrl Pts',(-18.6577547762499,38.8007515315423,6.30494916366897));
#62416=CARTESIAN_POINT('Ctrl Pts',(-18.5993680358662,38.7960746232213,6.2809307968082));
#62417=CARTESIAN_POINT('Ctrl Pts',(-18.5397589719614,38.7913977149004,6.26020351320154));
#62418=CARTESIAN_POINT('Ctrl Pts',(-18.4813281167611,38.7868132484621,6.23988591671902));
#62419=CARTESIAN_POINT('Ctrl Pts',(-18.421723322332,38.7822287820238,6.22273066249775));
#62420=CARTESIAN_POINT('Ctrl Pts',(-18.3613191598753,38.7776443155856,6.20886468524928));
#62421=CARTESIAN_POINT('Ctrl Pts',(-18.3009519341659,38.7730626525183,6.19500718695452));
#62422=CARTESIAN_POINT('Ctrl Pts',(-18.2397868048023,38.7684809894511,6.18443509104636));
#62423=CARTESIAN_POINT('Ctrl Pts',(-18.1782122388083,38.7638993263838,6.17722513487865));
#62424=CARTESIAN_POINT('Ctrl Pts',(-18.116652706087,38.7593187819179,6.17001693900329));
#62425=CARTESIAN_POINT('Ctrl Pts',(-18.0546844405703,38.754738237452,6.16616931252695));
#62426=CARTESIAN_POINT('Ctrl Pts',(-17.9927027640976,38.750157692986,6.16570733869318));
#62427=CARTESIAN_POINT('Ctrl Pts',(-17.9284562296966,38.7454097719172,6.16522848398171));
#62428=CARTESIAN_POINT('Ctrl Pts',(-17.8641958670951,38.7406618508484,6.16838756877484));
#62429=CARTESIAN_POINT('Ctrl Pts',(-17.8003613125996,38.7359139297795,6.17515346488567));
#62430=CARTESIAN_POINT('Ctrl Pts',(-17.7386990628092,38.7313275815667,6.18168911598151));
#62431=CARTESIAN_POINT('Ctrl Pts',(-17.6774346141508,38.7267412333538,6.19158987077987));
#62432=CARTESIAN_POINT('Ctrl Pts',(-17.6169558001157,38.7221548851409,6.20477516697284));
#62433=CARTESIAN_POINT('Ctrl Pts',(-17.5532810660628,38.7173261776441,6.21865722206749));
#62434=CARTESIAN_POINT('Ctrl Pts',(-17.4904779260827,38.7124974701473,6.23618041750083));
#62435=CARTESIAN_POINT('Ctrl Pts',(-17.4289800006369,38.7076687626505,6.25719133313902));
#62436=CARTESIAN_POINT('Ctrl Pts',(-17.3674820751911,38.7028400551537,6.27820224877722));
#62437=CARTESIAN_POINT('Ctrl Pts',(-17.3072899369963,38.6980113476569,6.30270056771319));
#62438=CARTESIAN_POINT('Ctrl Pts',(-17.2488088849698,38.6931826401601,6.33047592129877));
#62439=CARTESIAN_POINT('Ctrl Pts',(-17.1931326450915,38.6885855225027,6.35691914000543));
#62440=CARTESIAN_POINT('Ctrl Pts',(-17.1387783624963,38.6839884048453,6.38644082732598));
#62441=CARTESIAN_POINT('Ctrl Pts',(-17.0861081909103,38.6793912871879,6.41888585244221));
#62442=CARTESIAN_POINT('Ctrl Pts',(-17.0325238404077,38.6747143788651,6.45189401523234));
#62443=CARTESIAN_POINT('Ctrl Pts',(-16.9806831395575,38.6700374705423,6.48792782068988));
#62444=CARTESIAN_POINT('Ctrl Pts',(-16.9309448705333,38.6653605622195,6.52677322430665));
#62445=CARTESIAN_POINT('Ctrl Pts',(-16.8821897082562,38.6607760957974,6.5648508252005));
#62446=CARTESIAN_POINT('Ctrl Pts',(-16.8354550433037,38.6561916293753,6.60562956146449));
#62447=CARTESIAN_POINT('Ctrl Pts',(-16.7910506385862,38.6516071629532,6.64886354096122));
#62448=CARTESIAN_POINT('Ctrl Pts',(-16.7466733868738,38.6470254999025,6.6920710831603));
#62449=CARTESIAN_POINT('Ctrl Pts',(-16.7046239339443,38.6424438368519,6.73773053721606));
#62450=CARTESIAN_POINT('Ctrl Pts',(-16.6651774008687,38.6378621738012,6.78555711611273));
#62451=CARTESIAN_POINT('Ctrl Pts',(-16.6257404985668,38.6332816293523,6.83337201826824));
#62452=CARTESIAN_POINT('Ctrl Pts',(-16.5889055783388,38.6287010849034,6.88335260237634));
#62453=CARTESIAN_POINT('Ctrl Pts',(-16.5549080774639,38.6241205404544,6.93518031261509));
#62454=CARTESIAN_POINT('Ctrl Pts',(-16.519668281622,38.6193726193699,6.98890184745642));
#62455=CARTESIAN_POINT('Ctrl Pts',(-16.4874776552696,38.6146246982854,7.04460766067788));
#62456=CARTESIAN_POINT('Ctrl Pts',(-16.4585484351101,38.6098767772009,7.1019114821232));
#62457=CARTESIAN_POINT('Ctrl Pts',(-16.430603683228,38.6052904290058,7.15726524082667));
#62458=CARTESIAN_POINT('Ctrl Pts',(-16.4057020633575,38.6007040808107,7.21410947465085));
#62459=CARTESIAN_POINT('Ctrl Pts',(-16.3839861867937,38.5961177326157,7.27207463370862));
#62460=CARTESIAN_POINT('Ctrl Pts',(-16.3611227642605,38.5912890250864,7.33310288278007));
#62461=CARTESIAN_POINT('Ctrl Pts',(-16.3417913177011,38.5864603175571,7.39537319680126));
#62462=CARTESIAN_POINT('Ctrl Pts',(-16.326098069667,38.5816316100279,7.4584380478703));
#62463=CARTESIAN_POINT('Ctrl Pts',(-16.3104048216329,38.5768029024986,7.52150289893934));
#62464=CARTESIAN_POINT('Ctrl Pts',(-16.2983498164063,38.5719741949694,7.58536163400675));
#62465=CARTESIAN_POINT('Ctrl Pts',(-16.289976070027,38.5671454874401,7.64955964135714));
#62466=CARTESIAN_POINT('Ctrl Pts',(-16.2820039372485,38.5625483697549,7.71067864538824));
#62467=CARTESIAN_POINT('Ctrl Pts',(-16.2773352205106,38.5579512520697,7.77235620365296));
#62468=CARTESIAN_POINT('Ctrl Pts',(-16.2760359524258,38.5533541343845,7.83420390838896));
#62469=CARTESIAN_POINT('Ctrl Pts',(-16.2747141333794,38.5486772260651,7.89712508305084));
#62470=CARTESIAN_POINT('Ctrl Pts',(-16.2768800061052,38.5440003177458,7.96022185310059));
#62471=CARTESIAN_POINT('Ctrl Pts',(-16.2825482745709,38.5393234094264,8.0230766978926));
#62472=CARTESIAN_POINT('Ctrl Pts',(-16.2881045063467,38.5347389429754,8.08468917937825));
#62473=CARTESIAN_POINT('Ctrl Pts',(-16.2970258922303,38.5301544765243,8.14606868051974));
#62474=CARTESIAN_POINT('Ctrl Pts',(-16.3092737966711,38.5255700100732,8.20682159834258));
#62475=CARTESIAN_POINT('Ctrl Pts',(-16.3215142115988,38.5209883469932,8.26753736615562));
#62476=CARTESIAN_POINT('Ctrl Pts',(-16.3370770112835,38.5164066839133,8.32762681238334));
#62477=CARTESIAN_POINT('Ctrl Pts',(-16.3558720955259,38.5118250208333,8.38670435019317));
#62478=CARTESIAN_POINT('Ctrl Pts',(-16.3746625909961,38.5072444763548,8.44576746437193));
#62479=CARTESIAN_POINT('Ctrl Pts',(-16.3966836501738,38.5026639318762,8.50381867567267));
#62480=CARTESIAN_POINT('Ctrl Pts',(-16.4217952812562,38.4980833873977,8.5604874293457));
#62481=CARTESIAN_POINT('Ctrl Pts',(-16.4478245104311,38.4933354663412,8.61922690236418));
#62482=CARTESIAN_POINT('Ctrl Pts',(-16.4771743701782,38.4885875452847,8.67648037150759));
#62483=CARTESIAN_POINT('Ctrl Pts',(-16.5096353933687,38.4838396242283,8.73186005776232));
#62484=CARTESIAN_POINT('Ctrl Pts',(-16.5409917605711,38.4792532760032,8.7853551607221));
#62485=CARTESIAN_POINT('Ctrl Pts',(-16.5752505814897,38.4746669277781,8.83710156953606));
#62486=CARTESIAN_POINT('Ctrl Pts',(-16.6121786835575,38.470080579553,8.88677907230902));
#62487=CARTESIAN_POINT('Ctrl Pts',(-16.6510582002527,38.4652518720808,8.93908171420726));
#62488=CARTESIAN_POINT('Ctrl Pts',(-16.6928965253649,38.4604231646087,8.9890902262784));
#62489=CARTESIAN_POINT('Ctrl Pts',(-16.7373752360294,38.4555944571365,9.03647268787872));
#62490=CARTESIAN_POINT('Ctrl Pts',(-16.7818539466939,38.4507657496644,9.08385514947904));
#62491=CARTESIAN_POINT('Ctrl Pts',(-16.8289725182177,38.4459370421923,9.12861116928819));
#62492=CARTESIAN_POINT('Ctrl Pts',(-16.8783723022766,38.4411083347201,9.17045809283064));
#62493=CARTESIAN_POINT('Ctrl Pts',(-16.9254028216628,38.4365112170463,9.2102979946927));
#62494=CARTESIAN_POINT('Ctrl Pts',(-16.9746939146925,38.4319140993725,9.2476651759781));
#62495=CARTESIAN_POINT('Ctrl Pts',(-17.0259550395338,38.4273169816987,9.28229354208289));
#62496=CARTESIAN_POINT('Ctrl Pts',(-17.0781058867199,38.4226400733779,9.31752294125477));
#62497=CARTESIAN_POINT('Ctrl Pts',(-17.1322954609214,38.4179631650572,9.34991712971022));
#62498=CARTESIAN_POINT('Ctrl Pts',(-17.1881809263176,38.4132862567364,9.37923735381575));
#62499=CARTESIAN_POINT('Ctrl Pts',(-17.2429617821702,38.408701790297,9.40797804621053));
#62500=CARTESIAN_POINT('Ctrl Pts',(-17.2993716261166,38.4041173238577,9.43376493771716));
#62501=CARTESIAN_POINT('Ctrl Pts',(-17.3570587952702,38.3995328574183,9.45641706087959));
#62502=CARTESIAN_POINT('Ctrl Pts',(-17.4147106890981,38.3949511943502,9.4790553324172));
#62503=CARTESIAN_POINT('Ctrl Pts',(-17.4736378865083,38.390369531282,9.4985624508343));
#62504=CARTESIAN_POINT('Ctrl Pts',(-17.533467553412,38.3857878682138,9.5148050370011));
#62505=CARTESIAN_POINT('Ctrl Pts',(-17.5932826130535,38.3812073237471,9.53104365758143));
#62506=CARTESIAN_POINT('Ctrl Pts',(-17.6539992137182,38.3766267792804,9.54401919480753));
#62507=CARTESIAN_POINT('Ctrl Pts',(-17.7152300980239,38.3720462348137,9.55364834054133));
#62508=CARTESIAN_POINT('Ctrl Pts',(-17.778698405713,38.3672983137459,9.56362934263113));
#62509=CARTESIAN_POINT('Ctrl Pts',(-17.8427187439572,38.3625503926781,9.57001450583138));
#62510=CARTESIAN_POINT('Ctrl Pts',(-17.9068517104591,38.3578024716103,9.57276955673316));
#62511=CARTESIAN_POINT('Ctrl Pts',(-17.9688022172439,38.3532161233971,9.57543085261408));
#62512=CARTESIAN_POINT('Ctrl Pts',(-18.0308572821878,38.3486297751839,9.57470522713874));
#62513=CARTESIAN_POINT('Ctrl Pts',(-18.0926214200226,38.3440434269707,9.57061496269793));
#62514=CARTESIAN_POINT('Ctrl Pts',(-18.1576493990214,38.3392147194756,9.56630855384191));
#62515=CARTESIAN_POINT('Ctrl Pts',(-18.2223542086077,38.3343860119805,9.55827211271781));
#62516=CARTESIAN_POINT('Ctrl Pts',(-18.2862842989164,38.3295573044854,9.54659320165545));
#62517=CARTESIAN_POINT('Ctrl Pts',(-18.3502143892252,38.3247285969903,9.53491429059309));
#62518=CARTESIAN_POINT('Ctrl Pts',(-18.4133691469486,38.3198998894952,9.51959313825781));
#62519=CARTESIAN_POINT('Ctrl Pts',(-18.4753166045076,38.3150711820001,9.50077781959992));
#62520=CARTESIAN_POINT('Ctrl Pts',(-18.5342929977205,38.3104740643271,9.48286490314912));
#62521=CARTESIAN_POINT('Ctrl Pts',(-18.5924175507923,38.3058769466541,9.46171178475844));
#62522=CARTESIAN_POINT('Ctrl Pts',(-18.6493091405794,38.3012798289812,9.43741829450116));
#62523=CARTESIAN_POINT('Ctrl Pts',(-18.7071881788355,38.2966029206603,9.41270315018474));
#62524=CARTESIAN_POINT('Ctrl Pts',(-18.7637905101237,38.2919260123394,9.38473764481648));
#62525=CARTESIAN_POINT('Ctrl Pts',(-18.8187296274891,38.2872491040185,9.35368037244278));
#62526=CARTESIAN_POINT('Ctrl Pts',(-18.8725828404318,38.2826646375801,9.32323696558139));
#62527=CARTESIAN_POINT('Ctrl Pts',(-18.9248375251718,38.2780801711417,9.2898231632124));
#62528=CARTESIAN_POINT('Ctrl Pts',(-18.9751509413837,38.2734957047033,9.25363631040213));
#62529=CARTESIAN_POINT('Ctrl Pts',(-19.0254335912709,38.2689140416361,9.21747158561546));
#62530=CARTESIAN_POINT('Ctrl Pts',(-19.0737769139927,38.2643323785689,9.17853746933835));
#62531=CARTESIAN_POINT('Ctrl Pts',(-19.1198666738557,38.2597507155017,9.13707489969342));
#62532=CARTESIAN_POINT('Ctrl Pts',(-19.1659451810197,38.255170171036,9.09562245303071));
#62533=CARTESIAN_POINT('Ctrl Pts',(-19.209770839256,38.2505896265704,9.05164311877771));
#62534=CARTESIAN_POINT('Ctrl Pts',(-19.2510636625165,38.2460090821047,9.00541710460519));
#62535=CARTESIAN_POINT('Ctrl Pts',(-19.2938653571655,38.241261161036,8.95750195646996));
#62536=CARTESIAN_POINT('Ctrl Pts',(-19.3339450943942,38.2365132399673,8.90717315076404));
#62537=CARTESIAN_POINT('Ctrl Pts',(-19.3710358126974,38.2317653188985,8.85478129723972));
#62538=CARTESIAN_POINT('Ctrl Pts',(-19.4068643252429,38.2271789706864,8.80417235065824));
#62539=CARTESIAN_POINT('Ctrl Pts',(-19.4399037766589,38.2225926224744,8.75163900632939));
#62540=CARTESIAN_POINT('Ctrl Pts',(-19.4699584385784,38.2180062742623,8.69752564123957));
#62541=CARTESIAN_POINT('Ctrl Pts',(-19.5016012979122,38.2131775667652,8.64055272954281));
#62542=CARTESIAN_POINT('Ctrl Pts',(-19.5299348738889,38.2083488592682,8.58182875448926));
#62543=CARTESIAN_POINT('Ctrl Pts',(-19.5547878867937,38.2035201517712,8.52178059744654));
#62544=CARTESIAN_POINT('Ctrl Pts',(-19.5796408996986,38.1986914442742,8.46173244040382));
#62545=CARTESIAN_POINT('Ctrl Pts',(-19.6010132090966,38.1938627367771,8.40036074067821));
#62546=CARTESIAN_POINT('Ctrl Pts',(-19.6187949975821,38.1890340292801,8.33810873896993));
#62547=CARTESIAN_POINT('Ctrl Pts',(-19.6403677510782,38.1831758718387,8.2625850036274));
#62548=CARTESIAN_POINT('Ctrl Pts',(-19.6567316249322,38.1773177143972,8.18551169491221));
#62549=CARTESIAN_POINT('Ctrl Pts',(-19.6677069478144,38.1714595569558,8.10752914326218));
#62550=CARTESIAN_POINT('Ctrl Pts',(-19.6786822706967,38.1656013995144,8.02954659161215));
#62551=CARTESIAN_POINT('Ctrl Pts',(-19.6842688386404,38.1597432420729,7.95065458203133));
#62552=CARTESIAN_POINT('Ctrl Pts',(-19.6843393239652,38.1538850846314,7.87151802034673));
#62553=CARTESIAN_POINT('',(-19.6843398591675,37.3601350845258,7.86930714147356));
#62554=CARTESIAN_POINT('Ctrl Pts',(-19.684339323966,38.1538850845701,7.87151801951866));
#62555=CARTESIAN_POINT('Ctrl Pts',(-19.6843939994145,38.1493409108528,7.81013177524482));
#62556=CARTESIAN_POINT('Ctrl Pts',(-19.6811279138394,38.1447967371355,7.74867522821752));
#62557=CARTESIAN_POINT('Ctrl Pts',(-19.6745449565224,38.1402525634182,7.6875384261698));
#62558=CARTESIAN_POINT('Ctrl Pts',(-19.6679653226271,38.1357106838378,7.62643248918267));
#62559=CARTESIAN_POINT('Ctrl Pts',(-19.6580721916101,38.1311688042574,7.56564649212944));
#62560=CARTESIAN_POINT('Ctrl Pts',(-19.6449214208484,38.1266269246771,7.5055668813074));
#62561=CARTESIAN_POINT('Ctrl Pts',(-19.6317722530837,38.1220855987235,7.44549459381499));
#62562=CARTESIAN_POINT('Ctrl Pts',(-19.6153663460452,38.1175442727699,7.38612902791419));
#62563=CARTESIAN_POINT('Ctrl Pts',(-19.5958105189662,38.1130029468163,7.32784577618699));
#62564=CARTESIAN_POINT('Ctrl Pts',(-19.5762357963367,38.1084572328687,7.2695062090652));
#62565=CARTESIAN_POINT('Ctrl Pts',(-19.5535052420422,38.103911518921,7.21225153699297));
#62566=CARTESIAN_POINT('Ctrl Pts',(-19.5277749423548,38.0993658049733,7.15644021734786));
#62567=CARTESIAN_POINT('Ctrl Pts',(-19.5020316447147,38.0948177947067,7.10060070398162));
#62568=CARTESIAN_POINT('Ctrl Pts',(-19.473285828702,38.0902697844401,7.04620645300395));
#62569=CARTESIAN_POINT('Ctrl Pts',(-19.4417395089391,38.0857217741735,6.99359116640328));
#62570=CARTESIAN_POINT('Ctrl Pts',(-19.4101351427099,38.0811653953895,6.9408790656105));
#62571=CARTESIAN_POINT('Ctrl Pts',(-19.3757202766866,38.0766090166055,6.88995289366633));
#62572=CARTESIAN_POINT('Ctrl Pts',(-19.3387395567511,38.0720526378215,6.84111630758394));
#62573=CARTESIAN_POINT('Ctrl Pts',(-19.3142399422629,38.0690340507344,6.8087622178305));
#62574=CARTESIAN_POINT('Ctrl Pts',(-19.2886150194716,38.0660154636472,6.77732458050104));
#62575=CARTESIAN_POINT('Ctrl Pts',(-19.2619447992417,38.0629968765601,6.74688274552598));
#62576=CARTESIAN_POINT('Ctrl Pts',(-19.2213277366001,38.0583997588854,6.70052175159917));
#62577=CARTESIAN_POINT('Ctrl Pts',(-19.178109068014,38.0538026412107,6.65627172587807));
#62578=CARTESIAN_POINT('Ctrl Pts',(-19.1325367588251,38.049205523536,6.61443882858826));
#62579=CARTESIAN_POINT('Ctrl Pts',(-19.0861734661884,38.0445286152154,6.57187985158207));
#62580=CARTESIAN_POINT('Ctrl Pts',(-19.037374329153,38.0398517068947,6.53182317146351));
#62581=CARTESIAN_POINT('Ctrl Pts',(-18.9864430772941,38.035174798574,6.49455564715733));
#62582=CARTESIAN_POINT('Ctrl Pts',(-18.9365185119837,38.0305903321338,6.45802473768087));
#62583=CARTESIAN_POINT('Ctrl Pts',(-18.8845457805321,38.0260058656936,6.4241740441216));
#62584=CARTESIAN_POINT('Ctrl Pts',(-18.8308458937871,38.0214213992534,6.39323458172068));
#62585=CARTESIAN_POINT('Ctrl Pts',(-18.7771788441709,38.0168397361843,6.36231403859829));
#62586=CARTESIAN_POINT('Ctrl Pts',(-18.721787173621,38.0122580731153,6.33430145038162));
#62587=CARTESIAN_POINT('Ctrl Pts',(-18.6650198733706,38.0076764100463,6.30938390092651));
#62588=CARTESIAN_POINT('Ctrl Pts',(-18.6082664327135,38.0030958655787,6.28447243502831));
#62589=CARTESIAN_POINT('Ctrl Pts',(-18.5501384950162,37.9985153211112,6.26265471234632));
#62590=CARTESIAN_POINT('Ctrl Pts',(-18.4910067256778,37.9939347766437,6.24407043144173));
#62591=CARTESIAN_POINT('Ctrl Pts',(-18.4297142362459,37.9891868555767,6.22480706669403));
#62592=CARTESIAN_POINT('Ctrl Pts',(-18.3673436697886,37.9844389345097,6.20901825874842));
#62593=CARTESIAN_POINT('Ctrl Pts',(-18.3043245188214,37.9796910134428,6.19680292789783));
#62594=CARTESIAN_POINT('Ctrl Pts',(-18.2434499241491,37.9751046652287,6.18500328758365));
#62595=CARTESIAN_POINT('Ctrl Pts',(-18.1819707144308,37.9705183170147,6.17653780523465));
#62596=CARTESIAN_POINT('Ctrl Pts',(-18.1202813180055,37.9659319688007,6.17144296904147));
#62597=CARTESIAN_POINT('Ctrl Pts',(-18.0553320300569,37.9611032613073,6.1660789032192));
#62598=CARTESIAN_POINT('Ctrl Pts',(-17.9901503705743,37.9562745538138,6.16445162514072));
#62599=CARTESIAN_POINT('Ctrl Pts',(-17.925195875559,37.9514458463204,6.16654135842861));
#62600=CARTESIAN_POINT('Ctrl Pts',(-17.8602413805436,37.946617138827,6.16863109171649));
#62601=CARTESIAN_POINT('Ctrl Pts',(-17.7955146903895,37.9417884313335,6.17443770098243));
#62602=CARTESIAN_POINT('Ctrl Pts',(-17.7314649292784,37.9369597238401,6.18387866562889));
#62603=CARTESIAN_POINT('Ctrl Pts',(-17.6704870611287,37.9323626061653,6.19286683182079));
#62604=CARTESIAN_POINT('Ctrl Pts',(-17.6098721581796,37.9277654884906,6.20518558302436));
#62605=CARTESIAN_POINT('Ctrl Pts',(-17.5500119205432,37.9231683708158,6.22079258820333));
#62606=CARTESIAN_POINT('Ctrl Pts',(-17.4891127086272,37.9184914624952,6.23667047899189));
#62607=CARTESIAN_POINT('Ctrl Pts',(-17.4289951475099,37.9138145541745,6.25595187527877));
#62608=CARTESIAN_POINT('Ctrl Pts',(-17.3700649579288,37.9091376458538,6.27853712576962));
#62609=CARTESIAN_POINT('Ctrl Pts',(-17.312299558667,37.9045531794136,6.3006759653238));
#62610=CARTESIAN_POINT('Ctrl Pts',(-17.2556755183872,37.8999687129733,6.32598905149395));
#62611=CARTESIAN_POINT('Ctrl Pts',(-17.2005610075826,37.895384246533,6.35433193188636));
#62612=CARTESIAN_POINT('Ctrl Pts',(-17.1454801989402,37.8908025834639,6.3826574807931));
#62613=CARTESIAN_POINT('Ctrl Pts',(-17.091907541249,37.8862209203948,6.41400891796747));
#62614=CARTESIAN_POINT('Ctrl Pts',(-17.0401894652584,37.8816392573258,6.44819445971376));
#62615=CARTESIAN_POINT('Ctrl Pts',(-16.9884840161057,37.8770587128582,6.48237165514613));
#62616=CARTESIAN_POINT('Ctrl Pts',(-16.9386326742921,37.8724781683906,6.51938130096242));
#62617=CARTESIAN_POINT('Ctrl Pts',(-16.8909538092563,37.867897623923,6.55898770790408));
#62618=CARTESIAN_POINT('Ctrl Pts',(-16.841532722014,37.8631497028561,6.60004136325739));
#62619=CARTESIAN_POINT('Ctrl Pts',(-16.7944464418052,37.8584017817892,6.64388490591297));
#62620=CARTESIAN_POINT('Ctrl Pts',(-16.7500109741647,37.8536538607223,6.69021110705151));
#62621=CARTESIAN_POINT('Ctrl Pts',(-16.7070876557729,37.8490675125082,6.73496081684271));
#62622=CARTESIAN_POINT('Ctrl Pts',(-16.6666379116302,37.8444811642942,6.78202647117671));
#62623=CARTESIAN_POINT('Ctrl Pts',(-16.6289062771767,37.8398948160801,6.83109644925646));
#62624=CARTESIAN_POINT('Ctrl Pts',(-16.5891807662652,37.8350661085868,6.88275946300789));
#62625=CARTESIAN_POINT('Ctrl Pts',(-16.5524689747073,37.8302374010934,6.93664397959055));
#62626=CARTESIAN_POINT('Ctrl Pts',(-16.5190034677509,37.8254086936001,6.99235316421911));
#62627=CARTESIAN_POINT('Ctrl Pts',(-16.4855379607946,37.8205799861068,7.04806234884768));
#62628=CARTESIAN_POINT('Ctrl Pts',(-16.4553189719353,37.8157512786134,7.10559559003678));
#62629=CARTESIAN_POINT('Ctrl Pts',(-16.4285207017313,37.8109225711201,7.16453077838679));
#62630=CARTESIAN_POINT('Ctrl Pts',(-16.4030077043532,37.806325453445,7.22063937399411));
#62631=CARTESIAN_POINT('Ctrl Pts',(-16.3804899460733,37.8017283357699,7.27824899691806));
#62632=CARTESIAN_POINT('Ctrl Pts',(-16.3611442575079,37.7971312180948,7.33700757922819));
#62633=CARTESIAN_POINT('Ctrl Pts',(-16.3414627922477,37.7924543097742,7.39678601474696));
#62634=CARTESIAN_POINT('Ctrl Pts',(-16.3250648660629,37.7877774014536,7.45775323064423));
#62635=CARTESIAN_POINT('Ctrl Pts',(-16.3120867506042,37.7831004931329,7.51951429688232));
#62636=CARTESIAN_POINT('Ctrl Pts',(-16.2993651553313,37.7785160266923,7.58005461884215));
#62637=CARTESIAN_POINT('Ctrl Pts',(-16.2899295218182,37.7739315602517,7.64135717253982));
#62638=CARTESIAN_POINT('Ctrl Pts',(-16.2838581174722,37.769347093811,7.70303428515065));
#62639=CARTESIAN_POINT('Ctrl Pts',(-16.2777904257503,37.7647654307416,7.76467368261133));
#62640=CARTESIAN_POINT('Ctrl Pts',(-16.2750829338365,37.7601837676721,7.82668667925809));
#62641=CARTESIAN_POINT('Ctrl Pts',(-16.275762352157,37.7556021046027,7.88867820319456));
#62642=CARTESIAN_POINT('Ctrl Pts',(-16.2764416045992,37.7510215601347,7.95065459205662));
#62643=CARTESIAN_POINT('Ctrl Pts',(-16.2805061201738,37.7464410156668,8.01260900979874));
#62644=CARTESIAN_POINT('Ctrl Pts',(-16.2879305028511,37.7418604711988,8.07414615455166));
#62645=CARTESIAN_POINT('Ctrl Pts',(-16.2956261781505,37.7371125501323,8.13793191364476));
#62646=CARTESIAN_POINT('Ctrl Pts',(-16.3069320119322,37.7323646290657,8.20126872867588));
#62647=CARTESIAN_POINT('Ctrl Pts',(-16.3217612174133,37.7276167079991,8.26372449190449));
#62648=CARTESIAN_POINT('Ctrl Pts',(-16.3360857816018,37.7230303597847,8.32405487106394));
#62649=CARTESIAN_POINT('Ctrl Pts',(-16.3536975343428,37.7184440115703,8.38356271747965));
#62650=CARTESIAN_POINT('Ctrl Pts',(-16.3744672442257,37.7138576633558,8.44187359244485));
#62651=CARTESIAN_POINT('Ctrl Pts',(-16.396334500928,37.7090289558632,8.50326582558571));
#62652=CARTESIAN_POINT('Ctrl Pts',(-16.4217024861552,37.7042002483706,8.56333047484713));
#62653=CARTESIAN_POINT('Ctrl Pts',(-16.4503638792474,37.699371540878,8.62165695213241));
#62654=CARTESIAN_POINT('Ctrl Pts',(-16.4790252723396,37.6945428333853,8.67998342941768));
#62655=CARTESIAN_POINT('Ctrl Pts',(-16.5109796861268,37.6897141258927,8.73657120696363));
#62656=CARTESIAN_POINT('Ctrl Pts',(-16.5459669156816,37.6848854184001,8.79104503075598));
#62657=CARTESIAN_POINT('Ctrl Pts',(-16.5792761214321,37.6802883007252,8.84290623348067));
#62658=CARTESIAN_POINT('Ctrl Pts',(-16.6154706772694,37.6756911830504,8.89306470453681));
#62659=CARTESIAN_POINT('Ctrl Pts',(-16.6543506546144,37.6710940653755,8.94118095981901));
#62660=CARTESIAN_POINT('Ctrl Pts',(-16.6939054588227,37.6664171570549,8.99013235297523));
#62661=CARTESIAN_POINT('Ctrl Pts',(-16.7362395867746,37.6617402487342,9.03696946441502));
#62662=CARTESIAN_POINT('Ctrl Pts',(-16.7810951033588,37.6570633404136,9.08136364664361));
#62663=CARTESIAN_POINT('Ctrl Pts',(-16.8250640239252,37.6524788739732,9.12488035140286));
#62664=CARTESIAN_POINT('Ctrl Pts',(-16.871455187435,37.6478944075328,9.1660494443908));
#62665=CARTESIAN_POINT('Ctrl Pts',(-16.9199853038366,37.6433099410924,9.2045949496074));
#62666=CARTESIAN_POINT('Ctrl Pts',(-16.9684857443899,37.6387282780232,9.24311688450012));
#62667=CARTESIAN_POINT('Ctrl Pts',(-17.019122146548,37.634146614954,9.279018096759));
#62668=CARTESIAN_POINT('Ctrl Pts',(-17.0715770468266,37.6295649518848,9.31206191744591));
#62669=CARTESIAN_POINT('Ctrl Pts',(-17.1240191403734,37.6249844074171,9.34509767056718));
#62670=CARTESIAN_POINT('Ctrl Pts',(-17.178278420132,37.6204038629494,9.37527714578282));
#62671=CARTESIAN_POINT('Ctrl Pts',(-17.2340089748521,37.6158233184818,9.40240733031358));
#62672=CARTESIAN_POINT('Ctrl Pts',(-17.2917759666773,37.611075397415,9.43052887254254));
#62673=CARTESIAN_POINT('Ctrl Pts',(-17.3511233424126,37.6063274763481,9.45537365085896));
#62674=CARTESIAN_POINT('Ctrl Pts',(-17.4116409768806,37.6015795552813,9.4767802763411));
#62675=CARTESIAN_POINT('Ctrl Pts',(-17.4700991822432,37.5969932070672,9.49745842940434));
#62676=CARTESIAN_POINT('Ctrl Pts',(-17.5296487457302,37.592406858853,9.51492860707238));
#62677=CARTESIAN_POINT('Ctrl Pts',(-17.5899049813651,37.5878205106388,9.52909635405429));
#62678=CARTESIAN_POINT('Ctrl Pts',(-17.653345375101,37.5829918031457,9.54401277618743));
#62679=CARTESIAN_POINT('Ctrl Pts',(-17.7175685644248,37.5781630956526,9.55526794030782));
#62680=CARTESIAN_POINT('Ctrl Pts',(-17.7821171463219,37.5733343881595,9.56281340135887));
#62681=CARTESIAN_POINT('Ctrl Pts',(-17.8466657282189,37.5685056806663,9.57035886240993));
#62682=CARTESIAN_POINT('Ctrl Pts',(-17.9115390493107,37.5636769731732,9.57419465952163));
#62683=CARTESIAN_POINT('Ctrl Pts',(-17.976280718664,37.5588482656801,9.57433594181028));
#62684=CARTESIAN_POINT('Ctrl Pts',(-18.037917310428,37.554251148005,9.57447044805388));
#62685=CARTESIAN_POINT('Ctrl Pts',(-18.0996878045383,37.5496540303299,9.57125732671632));
#62686=CARTESIAN_POINT('Ctrl Pts',(-18.1611985492709,37.5450569126547,9.56468047765416));
#62687=CARTESIAN_POINT('Ctrl Pts',(-18.2237769155815,37.5403800043341,9.55798947640599));
#62688=CARTESIAN_POINT('Ctrl Pts',(-18.2860858994534,37.5357030960135,9.54781677144421));
#62689=CARTESIAN_POINT('Ctrl Pts',(-18.3477095004604,37.5310261876929,9.53420087695902));
#62690=CARTESIAN_POINT('Ctrl Pts',(-18.4081150742713,37.5264417212523,9.52085410874218));
#62691=CARTESIAN_POINT('Ctrl Pts',(-18.4678615913966,37.5218572548116,9.50419914068351));
#62692=CARTESIAN_POINT('Ctrl Pts',(-18.5265635584022,37.517272788371,9.48432435161796));
#62693=CARTESIAN_POINT('Ctrl Pts',(-18.5852296295396,37.5126911253015,9.46446171585568));
#62694=CARTESIAN_POINT('Ctrl Pts',(-18.6428519358873,37.5081094622321,9.44138332603462));
#62695=CARTESIAN_POINT('Ctrl Pts',(-18.6990594801508,37.5035277991626,9.41522758828767));
#62696=CARTESIAN_POINT('Ctrl Pts',(-18.7552533014838,37.4989472546947,9.3890782363982));
#62697=CARTESIAN_POINT('Ctrl Pts',(-18.8100325850791,37.4943667102267,9.3598532427556));
#62698=CARTESIAN_POINT('Ctrl Pts',(-18.8630475886996,37.4897861657588,9.32773858825642));
#62699=CARTESIAN_POINT('Ctrl Pts',(-18.9179998011045,37.4850382446922,9.29445043971674));
#62700=CARTESIAN_POINT('Ctrl Pts',(-18.9710557700258,37.4802903236257,9.25805760831249));
#62701=CARTESIAN_POINT('Ctrl Pts',(-19.0218575044375,37.4755424025591,9.21881717665783));
#62702=CARTESIAN_POINT('Ctrl Pts',(-19.0709304440763,37.4709560543447,9.18091210596905));
#62703=CARTESIAN_POINT('Ctrl Pts',(-19.1178997652097,37.4663697061303,9.14035054174966));
#62704=CARTESIAN_POINT('Ctrl Pts',(-19.1624775100696,37.4617833579158,9.09740448662189));
#62705=CARTESIAN_POINT('Ctrl Pts',(-19.209410904689,37.4569546504232,9.05218900613965));
#62706=CARTESIAN_POINT('Ctrl Pts',(-19.2536925069757,37.4521259429306,9.00433050152082));
#62707=CARTESIAN_POINT('Ctrl Pts',(-19.2950335873058,37.447297235438,8.9541870225462));
#62708=CARTESIAN_POINT('Ctrl Pts',(-19.3363746676359,37.4424685279453,8.90404354357157));
#62709=CARTESIAN_POINT('Ctrl Pts',(-19.3747749045952,37.4376398204527,8.85161566044052));
#62710=CARTESIAN_POINT('Ctrl Pts',(-19.4099995504222,37.4328111129601,8.79729505627508));
#62711=CARTESIAN_POINT('Ctrl Pts',(-19.4442592518619,37.4281146831408,8.74446251141809));
#62712=CARTESIAN_POINT('Ctrl Pts',(-19.4756515793317,37.4234182533215,8.68963005408069));
#62713=CARTESIAN_POINT('Ctrl Pts',(-19.5039428546648,37.4187218235022,8.63313367853616));
#62714=CARTESIAN_POINT('Ctrl Pts',(-19.5333533790022,37.4138395952578,8.57440221421144));
#62715=CARTESIAN_POINT('Ctrl Pts',(-19.5594119799198,37.4089573670135,8.51387279618993));
#62716=CARTESIAN_POINT('Ctrl Pts',(-19.5819054569772,37.4040751387692,8.45195682185774));
#62717=CARTESIAN_POINT('Ctrl Pts',(-19.6034658205024,37.3993954436072,8.3926093536465));
#62718=CARTESIAN_POINT('Ctrl Pts',(-19.6217508084192,37.3947157484452,8.33198859873641));
#62719=CARTESIAN_POINT('Ctrl Pts',(-19.6366201226328,37.3900360532833,8.27048046754878));
#62720=CARTESIAN_POINT('Ctrl Pts',(-19.6514743036184,37.3853611208759,8.20903493619342));
#62721=CARTESIAN_POINT('Ctrl Pts',(-19.6629196009608,37.3806861884685,8.14670428650603));
#62722=CARTESIAN_POINT('Ctrl Pts',(-19.6708654690599,37.3760112560611,8.08388969386272));
#62723=CARTESIAN_POINT('Ctrl Pts',(-19.678804960735,37.3713400752075,8.02112550886222));
#62724=CARTESIAN_POINT('Ctrl Pts',(-19.683250545557,37.3666688943539,7.95787862815727));
#62725=CARTESIAN_POINT('Ctrl Pts',(-19.6841630505933,37.3619977135002,7.89455875796057));
#62726=CARTESIAN_POINT('Ctrl Pts',(-19.6842843374322,37.3613768371902,7.88614251192121));
#62727=CARTESIAN_POINT('Ctrl Pts',(-19.6843432812367,37.3607559608802,7.87772498405695));
#62728=CARTESIAN_POINT('Ctrl Pts',(-19.6843398591677,37.3601350845702,7.86930714207592));
#62729=CARTESIAN_POINT('',(-19.6843396079794,36.5663850846257,7.86884402740817));
#62730=CARTESIAN_POINT('Ctrl Pts',(-19.6843398591675,37.3601350845258,7.86930714147356));
#62731=CARTESIAN_POINT('Ctrl Pts',(-19.684312342679,37.3551426892111,7.80162023799952));
#62732=CARTESIAN_POINT('Ctrl Pts',(-19.6802484007567,37.3501502938964,7.73406057782156));
#62733=CARTESIAN_POINT('Ctrl Pts',(-19.6722183804769,37.3451578985817,7.6670916749466));
#62734=CARTESIAN_POINT('Ctrl Pts',(-19.6641639652474,37.3401503365266,7.59991932264465));
#62735=CARTESIAN_POINT('Ctrl Pts',(-19.6521194773108,37.3351427744715,7.53334165648438));
#62736=CARTESIAN_POINT('Ctrl Pts',(-19.6362060715679,37.3301352124164,7.4678106365136));
#62737=CARTESIAN_POINT('Ctrl Pts',(-19.6202226848285,37.3251056290424,7.40199143649161));
#62738=CARTESIAN_POINT('Ctrl Pts',(-19.6003364347516,37.3200760456684,7.33722843146035));
#62739=CARTESIAN_POINT('Ctrl Pts',(-19.5767183878877,37.3150464622943,7.27395870496986));
#62740=CARTESIAN_POINT('Ctrl Pts',(-19.5637696453067,37.3122889616096,7.23927067990921));
#62741=CARTESIAN_POINT('Ctrl Pts',(-19.5497000125454,37.3095314609248,7.20503111778527));
#62742=CARTESIAN_POINT('Ctrl Pts',(-19.5345435224027,37.30677396024,7.1713088861623));
#62743=CARTESIAN_POINT('Ctrl Pts',(-19.5092756524411,37.3021768425653,7.1150894741849));
#62744=CARTESIAN_POINT('Ctrl Pts',(-19.4809022245421,37.2975797248906,7.06012706266653));
#62745=CARTESIAN_POINT('Ctrl Pts',(-19.4495707280332,37.2929826072159,7.00678698404857));
#62746=CARTESIAN_POINT('Ctrl Pts',(-19.4176954211366,37.2883056988952,6.95252109938666));
#62747=CARTESIAN_POINT('Ctrl Pts',(-19.38275851271,37.2836287905746,6.89993492413997));
#62748=CARTESIAN_POINT('Ctrl Pts',(-19.3449664635909,37.2789518822539,6.84939165745511));
#62749=CARTESIAN_POINT('Ctrl Pts',(-19.3079213968469,37.2743674158137,6.79984740856048));
#62750=CARTESIAN_POINT('Ctrl Pts',(-19.2681333488877,37.2697829493735,6.75226647216188));
#62751=CARTESIAN_POINT('Ctrl Pts',(-19.2258416508355,37.2651984829332,6.70696370794222));
#62752=CARTESIAN_POINT('Ctrl Pts',(-19.1835758138795,37.2606168198642,6.66168864606606));
#62753=CARTESIAN_POINT('Ctrl Pts',(-19.1388097091757,37.2560351567952,6.61868936543772));
#62754=CARTESIAN_POINT('Ctrl Pts',(-19.0918222818161,37.2514534937261,6.5782469085552));
#62755=CARTESIAN_POINT('Ctrl Pts',(-19.0448463263186,37.2468729492586,6.53781432559668));
#62756=CARTESIAN_POINT('Ctrl Pts',(-18.9956505104337,37.2422924047911,6.49993765911998));
#62757=CARTESIAN_POINT('Ctrl Pts',(-18.9445483741916,37.2377118603236,6.46485898592195));
#62758=CARTESIAN_POINT('Ctrl Pts',(-18.891578926793,37.2329639392566,6.42849851116655));
#62759=CARTESIAN_POINT('Ctrl Pts',(-18.8365615891362,37.2282160181896,6.39514485209127));
#62760=CARTESIAN_POINT('Ctrl Pts',(-18.7798780879788,37.2234680971227,6.3650183124133));
#62761=CARTESIAN_POINT('Ctrl Pts',(-18.7251235394868,37.2188817489087,6.33591698585419));
#62762=CARTESIAN_POINT('Ctrl Pts',(-18.6688149218315,37.2142954006947,6.30982681152079));
#62763=CARTESIAN_POINT('Ctrl Pts',(-18.6113187077245,37.2097090524807,6.28689813186988));
#62764=CARTESIAN_POINT('Ctrl Pts',(-18.5507841850613,37.2048803449873,6.26275781759838));
#62765=CARTESIAN_POINT('Ctrl Pts',(-18.4889336801542,37.2000516374938,6.24212260958859));
#62766=CARTESIAN_POINT('Ctrl Pts',(-18.4262123908774,37.1952229300004,6.22510810755617));
#62767=CARTESIAN_POINT('Ctrl Pts',(-18.3634911016007,37.190394222507,6.20809360552376));
#62768=CARTESIAN_POINT('Ctrl Pts',(-18.2998996799295,37.1855655150136,6.19469986745871));
#62769=CARTESIAN_POINT('Ctrl Pts',(-18.2358917336808,37.1807368075201,6.1849794493141));
#62770=CARTESIAN_POINT('Ctrl Pts',(-18.1749536748877,37.1761396898437,6.17572523250032));
#62771=CARTESIAN_POINT('Ctrl Pts',(-18.1133877947718,37.1715425721674,6.16976197005564));
#62772=CARTESIAN_POINT('Ctrl Pts',(-18.051581028338,37.166945454491,6.16716383877307));
#62773=CARTESIAN_POINT('Ctrl Pts',(-17.9887015023952,37.1622685461705,6.16452061258908));
#62774=CARTESIAN_POINT('Ctrl Pts',(-17.925573158648,37.1575916378501,6.16536062015343));
#62775=CARTESIAN_POINT('Ctrl Pts',(-17.8626131167544,37.1529147295296,6.16970733247424));
#62776=CARTESIAN_POINT('Ctrl Pts',(-17.800897517588,37.1483302630877,6.17396812943711));
#62777=CARTESIAN_POINT('Ctrl Pts',(-17.7393441601812,37.1437457966458,6.18159823189687));
#62778=CARTESIAN_POINT('Ctrl Pts',(-17.6783473722258,37.1391613302039,6.19256728070635));
#62779=CARTESIAN_POINT('Ctrl Pts',(-17.6173878834064,37.1345796671331,6.20352962201436));
#62780=CARTESIAN_POINT('Ctrl Pts',(-17.5569847891959,37.1299980040624,6.21782677128591));
#62781=CARTESIAN_POINT('Ctrl Pts',(-17.49752548396,37.1254163409917,6.23537674769628));
#62782=CARTESIAN_POINT('Ctrl Pts',(-17.4380806955638,37.1208357965224,6.25292243932408));
#62783=CARTESIAN_POINT('Ctrl Pts',(-17.3795797267511,37.1162552520532,6.27371923750358));
#62784=CARTESIAN_POINT('Ctrl Pts',(-17.3223959911261,37.111674707584,6.29763496505645));
#62785=CARTESIAN_POINT('Ctrl Pts',(-17.2631227180923,37.1069267865187,6.32242459157439));
#62786=CARTESIAN_POINT('Ctrl Pts',(-17.2052653691306,37.1021788654533,6.35056533045179));
#62787=CARTESIAN_POINT('Ctrl Pts',(-17.1492160376861,37.097430944388,6.38185590631751));
#62788=CARTESIAN_POINT('Ctrl Pts',(-17.0950740779267,37.0928445961723,6.41208165666479));
#62789=CARTESIAN_POINT('Ctrl Pts',(-17.0426194586066,37.0882582479567,6.44524595273187));
#62790=CARTESIAN_POINT('Ctrl Pts',(-16.992177218904,37.083671899741,6.48112239965223));
#62791=CARTESIAN_POINT('Ctrl Pts',(-16.9390694283006,37.0788431922509,6.51889468815235));
#62792=CARTESIAN_POINT('Ctrl Pts',(-16.8881931097297,37.0740144847607,6.55967332189239));
#62793=CARTESIAN_POINT('Ctrl Pts',(-16.8398867992758,37.0691857772705,6.60314692046219));
#62794=CARTESIAN_POINT('Ctrl Pts',(-16.7915804888219,37.0643570697804,6.64662051903199));
#62795=CARTESIAN_POINT('Ctrl Pts',(-16.7458445887407,37.0595283622902,6.69278856607415));
#62796=CARTESIAN_POINT('Ctrl Pts',(-16.7029692247785,37.0546996548001,6.74129842972684));
#62797=CARTESIAN_POINT('Ctrl Pts',(-16.6621502077228,37.0501025371273,6.78748171002631));
#62798=CARTESIAN_POINT('Ctrl Pts',(-16.6237558808871,37.0455054194545,6.83597700623768));
#62799=CARTESIAN_POINT('Ctrl Pts',(-16.5880583831769,37.0409083017818,6.88649943011922));
#62800=CARTESIAN_POINT('Ctrl Pts',(-16.5517412958278,37.0362313934609,6.9378987549708));
#62801=CARTESIAN_POINT('Ctrl Pts',(-16.5182159688866,37.03155448514,6.99139591238914));
#62802=CARTESIAN_POINT('Ctrl Pts',(-16.4877283047894,37.0268775768191,7.04665315736733));
#62803=CARTESIAN_POINT('Ctrl Pts',(-16.4578432475579,37.0222931103807,7.10081820993945));
#62804=CARTESIAN_POINT('Ctrl Pts',(-16.4308771215619,37.0177086439424,7.15667393762248));
#62805=CARTESIAN_POINT('Ctrl Pts',(-16.407018241228,37.0131241775041,7.21387255645679));
#62806=CARTESIAN_POINT('Ctrl Pts',(-16.383173950443,37.0085425144369,7.2710361987107));
#62807=CARTESIAN_POINT('Ctrl Pts',(-16.3624333333595,37.0039608513698,7.32954063499695));
#62808=CARTESIAN_POINT('Ctrl Pts',(-16.3449375712924,36.9993791883026,7.3890159152023));
#62809=CARTESIAN_POINT('Ctrl Pts',(-16.3274460807714,36.994798643837,7.448476674668));
#62810=CARTESIAN_POINT('Ctrl Pts',(-16.3131980161933,36.9902180993713,7.50890731935247));
#62811=CARTESIAN_POINT('Ctrl Pts',(-16.3022848018994,36.9856375549056,7.56992242725872));
#62812=CARTESIAN_POINT('Ctrl Pts',(-16.2909728103965,36.9808896338368,7.63316707394078));
#62813=CARTESIAN_POINT('Ctrl Pts',(-16.2832442686416,36.976141712768,7.69703916222988));
#62814=CARTESIAN_POINT('Ctrl Pts',(-16.2791426724025,36.9713937916992,7.76110010671339));
#62815=CARTESIAN_POINT('Ctrl Pts',(-16.2751806544359,36.966807443487,7.82298104237933));
#62816=CARTESIAN_POINT('Ctrl Pts',(-16.2746026142157,36.9622210952748,7.88503765754329));
#62817=CARTESIAN_POINT('Ctrl Pts',(-16.2773945816838,36.9576347470626,7.94687408614226));
#62818=CARTESIAN_POINT('Ctrl Pts',(-16.2803340868458,36.9528060395655,8.01197817605266));
#62819=CARTESIAN_POINT('Ctrl Pts',(-16.2870095896517,36.9479773320684,8.07683751952399));
#62820=CARTESIAN_POINT('Ctrl Pts',(-16.2973430321799,36.9431486245714,8.14099882702023));
#62821=CARTESIAN_POINT('Ctrl Pts',(-16.307676474708,36.9383199170743,8.20516013451646));
#62822=CARTESIAN_POINT('Ctrl Pts',(-16.3216676412264,36.9334912095772,8.26862278806169));
#62823=CARTESIAN_POINT('Ctrl Pts',(-16.3391775632061,36.9286625020801,8.33095180497942));
#62824=CARTESIAN_POINT('Ctrl Pts',(-16.3558476911547,36.9240653844061,8.39029145755644));
#62825=CARTESIAN_POINT('Ctrl Pts',(-16.3757751995548,36.9194682667322,8.44884752041912));
#62826=CARTESIAN_POINT('Ctrl Pts',(-16.3988682860906,36.9148711490582,8.50623685752226));
#62827=CARTESIAN_POINT('Ctrl Pts',(-16.4223621916703,36.9101942407375,8.56462228231588));
#62828=CARTESIAN_POINT('Ctrl Pts',(-16.4491325591648,36.9055173324167,8.62179955771093));
#62829=CARTESIAN_POINT('Ctrl Pts',(-16.4790289483411,36.900840424096,8.67737893066517));
#62830=CARTESIAN_POINT('Ctrl Pts',(-16.5083344175611,36.8962559576565,8.73185974417645));
#62831=CARTESIAN_POINT('Ctrl Pts',(-16.5406432049823,36.8916714912171,8.78480477720931));
#62832=CARTESIAN_POINT('Ctrl Pts',(-16.5757652085565,36.8870870247777,8.83586721970446));
#62833=CARTESIAN_POINT('Ctrl Pts',(-16.6108657352555,36.8825053617095,8.88689843785039));
#62834=CARTESIAN_POINT('Ctrl Pts',(-16.6487757791845,36.8779236986413,8.93604892953435));
#62835=CARTESIAN_POINT('Ctrl Pts',(-16.6892610560999,36.8733420355731,8.98299946734022));
#62836=CARTESIAN_POINT('Ctrl Pts',(-16.7297364486367,36.8687614911064,9.02993854229032));
#62837=CARTESIAN_POINT('Ctrl Pts',(-16.7727854937313,36.8641809466397,9.07467834424582));
#62838=CARTESIAN_POINT('Ctrl Pts',(-16.8181339268211,36.859600402173,9.11693306299734));
#62839=CARTESIAN_POINT('Ctrl Pts',(-16.8651394263687,36.8548524811053,9.16073180151654));
#62840=CARTESIAN_POINT('Ctrl Pts',(-16.9146152273539,36.8501045600376,9.20185988358829));
#62841=CARTESIAN_POINT('Ctrl Pts',(-16.9662164071788,36.8453566389698,9.24004294185492));
#62842=CARTESIAN_POINT('Ctrl Pts',(-17.0160615868918,36.8407702907567,9.276926621797));
#62843=CARTESIAN_POINT('Ctrl Pts',(-17.0678893257283,36.8361839425435,9.31106227917652));
#62844=CARTESIAN_POINT('Ctrl Pts',(-17.1213594340831,36.8315975943304,9.34224699495769));
#62845=CARTESIAN_POINT('Ctrl Pts',(-17.1776550969888,36.8267688868354,9.37507962427978));
#62846=CARTESIAN_POINT('Ctrl Pts',(-17.2357709504644,36.8219401793403,9.40464048260112));
#62847=CARTESIAN_POINT('Ctrl Pts',(-17.2952838051689,36.8171114718453,9.43074936108783));
#62848=CARTESIAN_POINT('Ctrl Pts',(-17.3547966598735,36.8122827643502,9.45685823957453));
#62849=CARTESIAN_POINT('Ctrl Pts',(-17.4157058795918,36.8074540568551,9.47951498439359));
#62850=CARTESIAN_POINT('Ctrl Pts',(-17.4775706282056,36.8026253493601,9.49860049182058));
#62851=CARTESIAN_POINT('Ctrl Pts',(-17.5364682794436,36.7980282316744,9.51677063855719));
#62852=CARTESIAN_POINT('Ctrl Pts',(-17.596473846165,36.7934311139887,9.5317789719462));
#62853=CARTESIAN_POINT('Ctrl Pts',(-17.6572156305096,36.788833996303,9.54349487194097));
#62854=CARTESIAN_POINT('Ctrl Pts',(-17.7190116896824,36.7841570879837,9.55541412089208));
#62855=CARTESIAN_POINT('Ctrl Pts',(-17.7815692878552,36.7794801796644,9.56392530793355));
#62856=CARTESIAN_POINT('Ctrl Pts',(-17.8444793712416,36.7748032713451,9.56894349369864));
#62857=CARTESIAN_POINT('Ctrl Pts',(-17.9061459995017,36.7702188048939,9.5738624920445));
#62858=CARTESIAN_POINT('Ctrl Pts',(-17.9681507735409,36.7656343384426,9.57542527236441));
#62859=CARTESIAN_POINT('Ctrl Pts',(-18.0300992146251,36.7610498719913,9.57360350560039));
#62860=CARTESIAN_POINT('Ctrl Pts',(-18.0920097746435,36.7564682089113,9.57178285283481));
#62861=CARTESIAN_POINT('Ctrl Pts',(-18.1538635622118,36.7518865458312,9.56658177168102));
#62862=CARTESIAN_POINT('Ctrl Pts',(-18.2152653164343,36.7473048827511,9.55802401241305));
#62863=CARTESIAN_POINT('Ctrl Pts',(-18.2766520795728,36.7427243382726,9.54946834250051));
#62864=CARTESIAN_POINT('Ctrl Pts',(-18.3375865244753,36.738143793794,9.5375576915874));
#62865=CARTESIAN_POINT('Ctrl Pts',(-18.3976797888509,36.7335632493155,9.52236752255226));
#62866=CARTESIAN_POINT('Ctrl Pts',(-18.4599689067945,36.7288153282592,9.50662229319178));
#62867=CARTESIAN_POINT('Ctrl Pts',(-18.5213535991595,36.7240674072029,9.48735331450911));
#62868=CARTESIAN_POINT('Ctrl Pts',(-18.5814163041024,36.7193194861466,9.4647016224861));
#62869=CARTESIAN_POINT('Ctrl Pts',(-18.63943506156,36.7147331379218,9.44282077268526));
#62870=CARTESIAN_POINT('Ctrl Pts',(-18.696219912393,36.710146789697,9.41778403264034));
#62871=CARTESIAN_POINT('Ctrl Pts',(-18.7514158934743,36.7055604414722,9.38976720417808));
#62872=CARTESIAN_POINT('Ctrl Pts',(-18.8095286300586,36.7007317340002,9.36026986505195));
#62873=CARTESIAN_POINT('Ctrl Pts',(-18.8658793526181,36.6959030265282,9.32746906024655));
#62874=CARTESIAN_POINT('Ctrl Pts',(-18.9200871732797,36.6910743190561,9.29162264410602));
#62875=CARTESIAN_POINT('Ctrl Pts',(-18.9742949939413,36.6862456115841,9.25577622796548));
#62876=CARTESIAN_POINT('Ctrl Pts',(-19.0263594384661,36.6814169041121,9.21688465163489));
#62877=CARTESIAN_POINT('Ctrl Pts',(-19.0759413917834,36.6765881966401,9.17525373065001));
#62878=CARTESIAN_POINT('Ctrl Pts',(-19.1230907030207,36.6719964003061,9.13566534981216));
#62879=CARTESIAN_POINT('Ctrl Pts',(-19.1682034839025,36.6674046039722,9.09342518089385));
#62880=CARTESIAN_POINT('Ctrl Pts',(-19.2109609351148,36.6628128076383,9.04877479266453));
#62881=CARTESIAN_POINT('Ctrl Pts',(-19.2530959184682,36.6582878591999,9.00477442988744));
#62882=CARTESIAN_POINT('Ctrl Pts',(-19.2929432957966,36.6537629107615,8.95843392556737));
#62883=CARTESIAN_POINT('Ctrl Pts',(-19.3302301661075,36.6492379623231,8.91002564109415));
#62884=CARTESIAN_POINT('Ctrl Pts',(-19.3674809633399,36.6447173915334,8.86166418908046));
#62885=CARTESIAN_POINT('Ctrl Pts',(-19.4021758408854,36.6401968207438,8.81123933213499));
#62886=CARTESIAN_POINT('Ctrl Pts',(-19.4340805176135,36.6356762499541,8.75905831299012));
#62887=CARTESIAN_POINT('Ctrl Pts',(-19.4659668223746,36.6311582822868,8.70690734172728));
#62888=CARTESIAN_POINT('Ctrl Pts',(-19.4950658374982,36.6266403146195,8.65300265920719));
#62889=CARTESIAN_POINT('Ctrl Pts',(-19.5211864923278,36.6221223469522,8.59768058340608));
#62890=CARTESIAN_POINT('Ctrl Pts',(-19.5480402662957,36.6174775750916,8.54080580255989));
#62891=CARTESIAN_POINT('Ctrl Pts',(-19.5717456588421,36.6128328032311,8.48243335371606));
#62892=CARTESIAN_POINT('Ctrl Pts',(-19.5921466851392,36.6081880313705,8.42295379661841));
#62893=CARTESIAN_POINT('Ctrl Pts',(-19.6120017637458,36.6036675572994,8.36506595977829));
#62894=CARTESIAN_POINT('Ctrl Pts',(-19.628727039104,36.5991470832283,8.30613007263316));
#62895=CARTESIAN_POINT('Ctrl Pts',(-19.6422292726584,36.5946266091571,8.24652181970979));
#62896=CARTESIAN_POINT('Ctrl Pts',(-19.6562884050324,36.5899196884019,8.18445502794113));
#62897=CARTESIAN_POINT('Ctrl Pts',(-19.6668526780841,36.5852127676466,8.12165980555281));
#62898=CARTESIAN_POINT('Ctrl Pts',(-19.6738761962583,36.5805058468914,8.0585689989087));
#62899=CARTESIAN_POINT('Ctrl Pts',(-19.6808997144325,36.5757989261361,7.9954781922646));
#62900=CARTESIAN_POINT('Ctrl Pts',(-19.6843825063727,36.5710920053809,7.93209243945));
#62901=CARTESIAN_POINT('Ctrl Pts',(-19.6843396079794,36.5663850846257,7.86884402740818));
#62902=CARTESIAN_POINT('',(-19.6843394141537,35.7726350845326,7.87141313913839));
#62903=CARTESIAN_POINT('Ctrl Pts',(-19.6843396079789,36.5663850845702,7.86884402666309));
#62904=CARTESIAN_POINT('Ctrl Pts',(-19.6842915046734,36.5611070710201,7.79792165657743));
#62905=CARTESIAN_POINT('Ctrl Pts',(-19.6798165048226,36.5558290574701,7.72714864521007));
#62906=CARTESIAN_POINT('Ctrl Pts',(-19.6709699394029,36.5505510439201,7.65693780336342));
#62907=CARTESIAN_POINT('Ctrl Pts',(-19.6632646347729,36.5459539262461,7.59578458749917));
#62908=CARTESIAN_POINT('Ctrl Pts',(-19.6522218556924,36.5413568085721,7.53492429571754));
#62909=CARTESIAN_POINT('Ctrl Pts',(-19.63787569595,36.5367596908982,7.47474943089457));
#62910=CARTESIAN_POINT('Ctrl Pts',(-19.6232805346711,36.5320827825774,7.41353013090068));
#62911=CARTESIAN_POINT('Ctrl Pts',(-19.6052661997884,36.5274058742567,7.35302081646679));
#62912=CARTESIAN_POINT('Ctrl Pts',(-19.5839237981891,36.5227289659359,7.29362921204945));
#62913=CARTESIAN_POINT('Ctrl Pts',(-19.5630032418838,36.5181444994969,7.23541151810847));
#62914=CARTESIAN_POINT('Ctrl Pts',(-19.5388851643774,36.513560033058,7.17826825427033));
#62915=CARTESIAN_POINT('Ctrl Pts',(-19.511706252538,36.508975566619,7.12257054410726));
#62916=CARTESIAN_POINT('Ctrl Pts',(-19.4845439604262,36.5043939035514,7.06690689273134));
#62917=CARTESIAN_POINT('Ctrl Pts',(-19.4543247680311,36.4998122404838,7.01268749885754));
#62918=CARTESIAN_POINT('Ctrl Pts',(-19.4212331397365,36.4952305774163,6.960262745335));
#62919=CARTESIAN_POINT('Ctrl Pts',(-19.3881495906809,36.4906500329504,6.90785079118619));
#62920=CARTESIAN_POINT('Ctrl Pts',(-19.3521952695133,36.4860694884845,6.85723303787884));
#62921=CARTESIAN_POINT('Ctrl Pts',(-19.3135991259382,36.4814889440186,6.80873273540695));
#62922=CARTESIAN_POINT('Ctrl Pts',(-19.2735926497222,36.4767410229504,6.75846019474391));
#62923=CARTESIAN_POINT('Ctrl Pts',(-19.2307478576811,36.4719931018822,6.71046334262124));
#62924=CARTESIAN_POINT('Ctrl Pts',(-19.1853652729516,36.467245180814,6.66506456838455));
#62925=CARTESIAN_POINT('Ctrl Pts',(-19.1415270681169,36.462658832602,6.62121072497537));
#62926=CARTESIAN_POINT('Ctrl Pts',(-19.0953214707558,36.4580724843901,6.57978126216683));
#62927=CARTESIAN_POINT('Ctrl Pts',(-19.0470548962871,36.4534861361782,6.54102720723496));
#62928=CARTESIAN_POINT('Ctrl Pts',(-18.9962377408532,36.4486574286818,6.50022524739323));
#62929=CARTESIAN_POINT('Ctrl Pts',(-18.9431362676737,36.4438287211855,6.46238967789154));
#62930=CARTESIAN_POINT('Ctrl Pts',(-18.8881423387969,36.4390000136891,6.42776134842927));
#62931=CARTESIAN_POINT('Ctrl Pts',(-18.8331484099201,36.4341713061928,6.393133018967));
#62932=CARTESIAN_POINT('Ctrl Pts',(-18.7762626317917,36.4293425986964,6.36171217583273));
#62933=CARTESIAN_POINT('Ctrl Pts',(-18.7179033614849,36.4245138912001,6.33368184782277));
#62934=CARTESIAN_POINT('Ctrl Pts',(-18.6623430613862,36.419916773447,6.30699588297241));
#62935=CARTESIAN_POINT('Ctrl Pts',(-18.6052191482576,36.4153196556939,6.28327296643721));
#62936=CARTESIAN_POINT('Ctrl Pts',(-18.5468798979243,36.4107225379407,6.26269728522304));
#62937=CARTESIAN_POINT('Ctrl Pts',(-18.4875280737191,36.4060456296299,6.24176447913884));
#62938=CARTESIAN_POINT('Ctrl Pts',(-18.4269187586668,36.401368721319,6.2240895165564));
#62939=CARTESIAN_POINT('Ctrl Pts',(-18.365443933186,36.3966918130082,6.20981693480204));
#62940=CARTESIAN_POINT('Ctrl Pts',(-18.3051841931071,36.392107346489,6.19582645886256));
#62941=CARTESIAN_POINT('Ctrl Pts',(-18.2440933657748,36.3875228799699,6.18510520861257));
#62942=CARTESIAN_POINT('Ctrl Pts',(-18.1825573944324,36.3829384134508,6.17773957749974));
#62943=CARTESIAN_POINT('Ctrl Pts',(-18.1210590519331,36.3783567503029,6.17037845042205));
#62944=CARTESIAN_POINT('Ctrl Pts',(-18.0591166095782,36.373775087155,6.16636893417111));
#62945=CARTESIAN_POINT('Ctrl Pts',(-17.9971244910363,36.3691934240071,6.16574603201085));
#62946=CARTESIAN_POINT('Ctrl Pts',(-17.9351475077161,36.3646128794609,6.16512328193061));
#62947=CARTESIAN_POINT('Ctrl Pts',(-17.873121381107,36.3600323349146,6.16788550967169));
#62948=CARTESIAN_POINT('Ctrl Pts',(-17.8114418593283,36.3554517903684,6.17401562836997));
#62949=CARTESIAN_POINT('Ctrl Pts',(-17.7475085227582,36.3507038693777,6.18036974608442));
#62950=CARTESIAN_POINT('Ctrl Pts',(-17.683948197553,36.345955948387,6.19034265594962));
#62951=CARTESIAN_POINT('Ctrl Pts',(-17.6211947190923,36.3412080273963,6.2038566670323));
#62952=CARTESIAN_POINT('Ctrl Pts',(-17.560576754033,36.3366216791049,6.21691079361959));
#62953=CARTESIAN_POINT('Ctrl Pts',(-17.5007120907975,36.3320353308135,6.23326866138507));
#62954=CARTESIAN_POINT('Ctrl Pts',(-17.4419778000741,36.3274489825221,6.25280893275195));
#62955=CARTESIAN_POINT('Ctrl Pts',(-17.3801397793381,36.3226202751818,6.27338178195278));
#62956=CARTESIAN_POINT('Ctrl Pts',(-17.3195555144789,36.3177915678415,6.29748247377392));
#62957=CARTESIAN_POINT('Ctrl Pts',(-17.2606398578557,36.3129628605011,6.32491235798932));
#62958=CARTESIAN_POINT('Ctrl Pts',(-17.2017242012325,36.3081341531608,6.35234224220473));
#62959=CARTESIAN_POINT('Ctrl Pts',(-17.1444776886246,36.3033054458204,6.38310094281609));
#62960=CARTESIAN_POINT('Ctrl Pts',(-17.0892809569805,36.2984767384801,6.41693619479307));
#62961=CARTESIAN_POINT('Ctrl Pts',(-17.0367315180382,36.2938796209698,6.44914867286746));
#62962=CARTESIAN_POINT('Ctrl Pts',(-16.985823826324,36.2892825034595,6.48428163117312));
#62963=CARTESIAN_POINT('Ctrl Pts',(-16.9369014906503,36.2846853859493,6.52214231634328));
#62964=CARTESIAN_POINT('Ctrl Pts',(-16.8871300242321,36.280008477608,6.56066013840899));
#62965=CARTESIAN_POINT('Ctrl Pts',(-16.8394139915803,36.2753315692668,6.60200108286855));
#62966=CARTESIAN_POINT('Ctrl Pts',(-16.7940873857918,36.2706546609256,6.64591417496078));
#62967=CARTESIAN_POINT('Ctrl Pts',(-16.7496566891601,36.2660701946487,6.68895929689248));
#62968=CARTESIAN_POINT('Ctrl Pts',(-16.7075222054155,36.2614857283718,6.73447544024023));
#62969=CARTESIAN_POINT('Ctrl Pts',(-16.6679658003392,36.2569012620949,6.7821851745263));
#62970=CARTESIAN_POINT('Ctrl Pts',(-16.6284335837389,36.2523195991884,6.82986573463028));
#62971=CARTESIAN_POINT('Ctrl Pts',(-16.5914766441364,36.2477379362818,6.87973683486253));
#62972=CARTESIAN_POINT('Ctrl Pts',(-16.5573382667583,36.2431562733753,6.93148605318312));
#62973=CARTESIAN_POINT('Ctrl Pts',(-16.5232082241712,36.2385757290691,6.98322263707437));
#62974=CARTESIAN_POINT('Ctrl Pts',(-16.4918956579468,36.233995184763,7.03683600404243));
#62975=CARTESIAN_POINT('Ctrl Pts',(-16.4636008043483,36.2294146404568,7.09198437353299));
#62976=CARTESIAN_POINT('Ctrl Pts',(-16.434272033143,36.2246667192321,7.14914791055222));
#62977=CARTESIAN_POINT('Ctrl Pts',(-16.4081861061293,36.2199187980073,7.20796031340688));
#62978=CARTESIAN_POINT('Ctrl Pts',(-16.3855129915753,36.2151708767826,7.26801493742372));
#62979=CARTESIAN_POINT('Ctrl Pts',(-16.3636114498346,36.2105845287254,7.32602588477298));
#62980=CARTESIAN_POINT('Ctrl Pts',(-16.3448942508113,36.2059981806682,7.38519533490138));
#62981=CARTESIAN_POINT('Ctrl Pts',(-16.3294639095098,36.201411832611,7.44514067082224));
#62982=CARTESIAN_POINT('Ctrl Pts',(-16.3132181713755,36.1965831248025,7.5082537420573));
#62983=CARTESIAN_POINT('Ctrl Pts',(-16.3006164407995,36.191754416994,7.5722263432863));
#62984=CARTESIAN_POINT('Ctrl Pts',(-16.2917167601815,36.1869257091856,7.63660218992504));
#62985=CARTESIAN_POINT('Ctrl Pts',(-16.2828170795634,36.1820970013771,7.70097803656378));
#62986=CARTESIAN_POINT('Ctrl Pts',(-16.2776194235065,36.1772682935686,7.7657564745557));
#62987=CARTESIAN_POINT('Ctrl Pts',(-16.2761182329847,36.1724395857601,7.83048089534406));
#62988=CARTESIAN_POINT('Ctrl Pts',(-16.2746890411959,36.167842468039,7.89210106239372));
#62989=CARTESIAN_POINT('Ctrl Pts',(-16.2766039256916,36.1632453503179,7.95392542127461));
#62990=CARTESIAN_POINT('Ctrl Pts',(-16.2818872519691,36.1586482325969,8.01556074530885));
#62991=CARTESIAN_POINT('Ctrl Pts',(-16.2872622791266,36.153971324282,8.07826585249882));
#62992=CARTESIAN_POINT('Ctrl Pts',(-16.2961239002959,36.1492944159671,8.14077477207092));
#62993=CARTESIAN_POINT('Ctrl Pts',(-16.3084423481408,36.1446175076523,8.20267078638046));
#62994=CARTESIAN_POINT('Ctrl Pts',(-16.3205173146481,36.1400330411699,8.26334338970927));
#62995=CARTESIAN_POINT('Ctrl Pts',(-16.3359135950058,36.1354485746876,8.32342657259014));
#62996=CARTESIAN_POINT('Ctrl Pts',(-16.3545509274159,36.1308641082052,8.38253307018724));
#62997=CARTESIAN_POINT('Ctrl Pts',(-16.3731768632127,36.1262824450957,8.44160342452705));
#62998=CARTESIAN_POINT('Ctrl Pts',(-16.3950397685123,36.1217007819863,8.49969779331158));
#62999=CARTESIAN_POINT('Ctrl Pts',(-16.4200090607561,36.1171191188768,8.55644235379012));
#63000=CARTESIAN_POINT('Ctrl Pts',(-16.4449722568007,36.1125385743705,8.61317306020581));
#63001=CARTESIAN_POINT('Ctrl Pts',(-16.4730401292783,36.1079580298643,8.66855414677424));
#63002=CARTESIAN_POINT('Ctrl Pts',(-16.5040340848873,36.103377485358,8.72223204177362));
#63003=CARTESIAN_POINT('Ctrl Pts',(-16.5361605828025,36.0986295643315,8.77787136718084));
#63004=CARTESIAN_POINT('Ctrl Pts',(-16.5714309102883,36.093881643305,8.83168008336001));
#63005=CARTESIAN_POINT('Ctrl Pts',(-16.609595561297,36.0891337222785,8.88329487809966));
#63006=CARTESIAN_POINT('Ctrl Pts',(-16.6464614609853,36.0845473740305,8.93315321022147));
#63007=CARTESIAN_POINT('Ctrl Pts',(-16.686027455947,36.0799610257825,8.98096418929041));
#63008=CARTESIAN_POINT('Ctrl Pts',(-16.7280276523126,36.0753746775344,9.02643420747833));
#63009=CARTESIAN_POINT('Ctrl Pts',(-16.7722472903959,36.0705459701187,9.07430702527207));
#63010=CARTESIAN_POINT('Ctrl Pts',(-16.8191650719499,36.065717262703,9.11958415431174));
#63011=CARTESIAN_POINT('Ctrl Pts',(-16.8684290911691,36.0608885552873,9.16196940762575));
#63012=CARTESIAN_POINT('Ctrl Pts',(-16.9176931103883,36.0560598478715,9.20435466093977));
#63013=CARTESIAN_POINT('Ctrl Pts',(-16.9693028039508,36.0512311404558,9.24384770520734));
#63014=CARTESIAN_POINT('Ctrl Pts',(-17.0228715062085,36.0464024330401,9.28020561691283));
#63015=CARTESIAN_POINT('Ctrl Pts',(-17.0738710048934,36.041805314814,9.31481977017882));
#63016=CARTESIAN_POINT('Ctrl Pts',(-17.1268553831708,36.0372081965879,9.34673488681428));
#63017=CARTESIAN_POINT('Ctrl Pts',(-17.1815074563142,36.0326110783618,9.37571726870559));
#63018=CARTESIAN_POINT('Ctrl Pts',(-17.2371080998668,36.0279341701101,9.40520268421062));
#63019=CARTESIAN_POINT('Ctrl Pts',(-17.2944344955896,36.0232572618583,9.43165221332123));
#63020=CARTESIAN_POINT('Ctrl Pts',(-17.3531203679941,36.0185803536066,9.45486490357257));
#63021=CARTESIAN_POINT('Ctrl Pts',(-17.4106462869812,36.0139958866101,9.47761878426245));
#63022=CARTESIAN_POINT('Ctrl Pts',(-17.4694779340439,36.0094114196135,9.49726242038527));
#63023=CARTESIAN_POINT('Ctrl Pts',(-17.529246399954,36.004826952617,9.51365325651294));
#63024=CARTESIAN_POINT('Ctrl Pts',(-17.588978317847,36.0002452889914,9.53003406975394));
#63025=CARTESIAN_POINT('Ctrl Pts',(-17.6496454287661,35.9956636253658,9.54316589266056));
#63026=CARTESIAN_POINT('Ctrl Pts',(-17.7108628315388,35.9910819617402,9.55295573921381));
#63027=CARTESIAN_POINT('Ctrl Pts',(-17.7720652882304,35.9865014167167,9.56274319559964));
#63028=CARTESIAN_POINT('Ctrl Pts',(-17.8338172676042,35.9819208716933,9.56919021502666));
#63029=CARTESIAN_POINT('Ctrl Pts',(-17.8957248501482,35.9773403266698,9.57225513208727));
#63030=CARTESIAN_POINT('Ctrl Pts',(-17.9598945680667,35.9725924061406,9.57543204281681));
#63031=CARTESIAN_POINT('Ctrl Pts',(-18.0242309024963,35.9678444856115,9.57497480613621));
#63032=CARTESIAN_POINT('Ctrl Pts',(-18.0882932978743,35.9630965650824,9.57089605715209));
#63033=CARTESIAN_POINT('Ctrl Pts',(-18.150175649512,35.9585102163204,9.56695610802298));
#63034=CARTESIAN_POINT('Ctrl Pts',(-18.2118018920341,35.9539238675584,9.55963731561465));
#63035=CARTESIAN_POINT('Ctrl Pts',(-18.2727811503428,35.9493375187964,9.54900388135465));
#63036=CARTESIAN_POINT('Ctrl Pts',(-18.3369827518602,35.9445088123837,9.53780854169233));
#63037=CARTESIAN_POINT('Ctrl Pts',(-18.4004664639146,35.9396801059709,9.5229386679061));
#63038=CARTESIAN_POINT('Ctrl Pts',(-18.4627926050996,35.9348513995582,9.50452933166129));
#63039=CARTESIAN_POINT('Ctrl Pts',(-18.5251187462847,35.9300226931455,9.48611999541648));
#63040=CARTESIAN_POINT('Ctrl Pts',(-18.5862867310796,35.9251939867328,9.46417148928455));
#63041=CARTESIAN_POINT('Ctrl Pts',(-18.6458827826311,35.9203652803201,9.43887697267678));
#63042=CARTESIAN_POINT('Ctrl Pts',(-18.7026205415385,35.9157681640155,9.41479560910305));
#63043=CARTESIAN_POINT('Ctrl Pts',(-18.7581668126214,35.9111710477108,9.38758297034592));
#63044=CARTESIAN_POINT('Ctrl Pts',(-18.8121532460799,35.9065739314062,9.35737883897773));
#63045=CARTESIAN_POINT('Ctrl Pts',(-18.8670767225288,35.9018970229143,9.32665045424125));
#63046=CARTESIAN_POINT('Ctrl Pts',(-18.9203851712327,35.8972201144224,9.29282585956303));
#63047=CARTESIAN_POINT('Ctrl Pts',(-18.971711136109,35.8925432059305,9.25610384102974));
#63048=CARTESIAN_POINT('Ctrl Pts',(-19.0220225958897,35.887958740854,9.22010766710573));
#63049=CARTESIAN_POINT('Ctrl Pts',(-19.0704287956415,35.8833742757776,9.18132787790683));
#63050=CARTESIAN_POINT('Ctrl Pts',(-19.1166099179761,35.8787898107012,9.1399971377757));
#63051=CARTESIAN_POINT('Ctrl Pts',(-19.1627628009093,35.8742081489899,9.0986916710744));
#63052=CARTESIAN_POINT('Ctrl Pts',(-19.2066929257736,35.8696264872786,9.05483868525564));
#63053=CARTESIAN_POINT('Ctrl Pts',(-19.2481134527839,35.8650448255673,9.00871116024585));
#63054=CARTESIAN_POINT('Ctrl Pts',(-19.2895238671477,35.8604642824494,8.9625948970762));
#63055=CARTESIAN_POINT('Ctrl Pts',(-19.328425559996,35.8558837393314,8.91420557571092));
#63056=CARTESIAN_POINT('Ctrl Pts',(-19.3645699219587,35.8513031962135,8.86385158188092));
#63057=CARTESIAN_POINT('Ctrl Pts',(-19.4020350479962,35.846555273829,8.81165758472919));
#63058=CARTESIAN_POINT('Ctrl Pts',(-19.4365370373085,35.8418073514446,8.7573529876506));
#63059=CARTESIAN_POINT('Ctrl Pts',(-19.4678476161369,35.8370594290601,8.7013148060487));
#63060=CARTESIAN_POINT('Ctrl Pts',(-19.4980926716629,35.83247308216,8.64718364726638));
#63061=CARTESIAN_POINT('Ctrl Pts',(-19.5253598851062,35.8278867352599,8.59143551198449));
#63062=CARTESIAN_POINT('Ctrl Pts',(-19.549491249346,35.8233003883598,8.53443363387662));
#63063=CARTESIAN_POINT('Ctrl Pts',(-19.5748978235564,35.8184716782332,8.47441951980089));
#63064=CARTESIAN_POINT('Ctrl Pts',(-19.5968277040167,35.8136429681065,8.41301608542877));
#63065=CARTESIAN_POINT('Ctrl Pts',(-19.6151559647572,35.8088142579799,8.35066600308205));
#63066=CARTESIAN_POINT('Ctrl Pts',(-19.6334842254977,35.8039855478533,8.28831592073533));
#63067=CARTESIAN_POINT('Ctrl Pts',(-19.6482107948462,35.7991568377267,8.22501984103038));
#63068=CARTESIAN_POINT('Ctrl Pts',(-19.6592736002429,35.7943281276001,8.16123016864215));
#63069=CARTESIAN_POINT('Ctrl Pts',(-19.6758401992731,35.7870971132568,8.06570485776181));
#63070=CARTESIAN_POINT('Ctrl Pts',(-19.6842587270469,35.7798660989135,7.96872710022575));
#63071=CARTESIAN_POINT('Ctrl Pts',(-19.6843394141533,35.7726350845702,7.87141313964419));
#63072=CARTESIAN_POINT('',(-19.6843399766484,34.9788850846098,7.87028213160167));
#63073=CARTESIAN_POINT('Ctrl Pts',(-19.6843394141537,35.7726350845326,7.8714131391384));
#63074=CARTESIAN_POINT('Ctrl Pts',(-19.6843898638469,35.7681138840299,7.81056746706279));
#63075=CARTESIAN_POINT('Ctrl Pts',(-19.6811777589129,35.7635926835272,7.74960646610825));
#63076=CARTESIAN_POINT('Ctrl Pts',(-19.6746925941157,35.7590714830244,7.68891480720527));
#63077=CARTESIAN_POINT('Ctrl Pts',(-19.6682138803083,35.7545547798968,7.62828352013334));
#63078=CARTESIAN_POINT('Ctrl Pts',(-19.658468608052,35.7500380767691,7.56792156436955));
#63079=CARTESIAN_POINT('Ctrl Pts',(-19.6454982932953,35.7455213736414,7.50821239569258));
#63080=CARTESIAN_POINT('Ctrl Pts',(-19.6325357833295,35.7410073884065,7.44853915656618));
#63081=CARTESIAN_POINT('Ctrl Pts',(-19.6163521865777,35.7364934031715,7.38951843896976));
#63082=CARTESIAN_POINT('Ctrl Pts',(-19.5970403871103,35.7319794179365,7.33152509617046));
#63083=CARTESIAN_POINT('Ctrl Pts',(-19.5777326210722,35.7274663754848,7.27354386576143));
#63084=CARTESIAN_POINT('Ctrl Pts',(-19.5552981152331,35.722953333033,7.21659008277439));
#63085=CARTESIAN_POINT('Ctrl Pts',(-19.5298793954744,35.7184402905813,7.16102278239427));
#63086=CARTESIAN_POINT('Ctrl Pts',(-19.504438441355,35.7139233004636,7.10540687597058));
#63087=CARTESIAN_POINT('Ctrl Pts',(-19.4760082787103,35.7094063103459,7.05118035357585));
#63088=CARTESIAN_POINT('Ctrl Pts',(-19.4447787212475,35.7048893202283,6.99868023471251));
#63089=CARTESIAN_POINT('Ctrl Pts',(-19.4135352439157,35.7003703167644,6.94615671510854));
#63090=CARTESIAN_POINT('Ctrl Pts',(-19.3794901817844,35.6958513133006,6.89536156744597));
#63091=CARTESIAN_POINT('Ctrl Pts',(-19.3428765130795,35.6913323098367,6.84660249868574));
#63092=CARTESIAN_POINT('Ctrl Pts',(-19.3061967613092,35.6868051501402,6.79775542594119));
#63093=CARTESIAN_POINT('Ctrl Pts',(-19.2669394870019,35.6822779904436,6.75095217067773));
#63094=CARTESIAN_POINT('Ctrl Pts',(-19.2253769567209,35.6777508307471,6.70646612800977));
#63095=CARTESIAN_POINT('Ctrl Pts',(-19.1964275659122,35.6745975454581,6.67548043426059));
#63096=CARTESIAN_POINT('Ctrl Pts',(-19.1663605874905,35.6714442601691,6.64561817842495));
#63097=CARTESIAN_POINT('Ctrl Pts',(-19.1352773691066,35.6682909748801,6.61696008202848));
#63098=CARTESIAN_POINT('Ctrl Pts',(-19.0899616695121,35.6636938534647,6.5751799268587));
#63099=CARTESIAN_POINT('Ctrl Pts',(-19.042283529149,35.6590967320493,6.53577536668713));
#63100=CARTESIAN_POINT('Ctrl Pts',(-18.9925220576629,35.6544996106339,6.49902446471642));
#63101=CARTESIAN_POINT('Ctrl Pts',(-18.9418969390844,35.6498227027808,6.46163572369713));
#63102=CARTESIAN_POINT('Ctrl Pts',(-18.8891158098682,35.6451457949278,6.42699406116622));
#63103=CARTESIAN_POINT('Ctrl Pts',(-18.834511174932,35.6404688870747,6.39535241921456));
#63104=CARTESIAN_POINT('Ctrl Pts',(-18.7809857835882,35.6358844168478,6.36433616445523));
#63105=CARTESIAN_POINT('Ctrl Pts',(-18.7257087743786,35.6312999466209,6.33620268827328));
#63106=CARTESIAN_POINT('Ctrl Pts',(-18.6690238994596,35.626715476394,6.31114756901959));
#63107=CARTESIAN_POINT('Ctrl Pts',(-18.61237368686,35.6221338095318,6.28610777075849));
#63108=CARTESIAN_POINT('Ctrl Pts',(-18.5543177802338,35.6175521426695,6.26414280230948));
#63109=CARTESIAN_POINT('Ctrl Pts',(-18.495223083031,35.6129704758072,6.24540158491029));
#63110=CARTESIAN_POINT('Ctrl Pts',(-18.4361428136328,35.6083899275461,6.22666494312673));
#63111=CARTESIAN_POINT('Ctrl Pts',(-18.3760247421643,35.6038093792849,6.21115064377193));
#63112=CARTESIAN_POINT('Ctrl Pts',(-18.3152522857029,35.5992288310237,6.1989581870788));
#63113=CARTESIAN_POINT('Ctrl Pts',(-18.2522592579376,35.5944809136184,6.18632022890303));
#63114=CARTESIAN_POINT('Ctrl Pts',(-18.1885636565305,35.5897329962131,6.1772517441605));
#63115=CARTESIAN_POINT('Ctrl Pts',(-18.1246030549647,35.5849850788078,6.17180543161424));
#63116=CARTESIAN_POINT('Ctrl Pts',(-18.062818949301,35.5803987268432,6.16654444998496));
#63117=CARTESIAN_POINT('Ctrl Pts',(-18.000788120127,35.5758123748785,6.16466301434031));
#63118=CARTESIAN_POINT('Ctrl Pts',(-17.9389066401533,35.5712260229139,6.16615547323809));
#63119=CARTESIAN_POINT('Ctrl Pts',(-17.8737552709548,35.5663973227882,6.16772679539626));
#63120=CARTESIAN_POINT('Ctrl Pts',(-17.8087701168144,35.5615686226626,6.17303842020226));
#63121=CARTESIAN_POINT('Ctrl Pts',(-17.7444060044007,35.556739922537,6.18202182927694));
#63122=CARTESIAN_POINT('Ctrl Pts',(-17.6800418919871,35.5519112224114,6.19100523835162));
#63123=CARTESIAN_POINT('Ctrl Pts',(-17.6162994436632,35.5470825222857,6.20366022899527));
#63124=CARTESIAN_POINT('Ctrl Pts',(-17.553616462983,35.5422538221601,6.21985700166293));
#63125=CARTESIAN_POINT('Ctrl Pts',(-17.4939398764833,35.5376567156154,6.23527694651285));
#63126=CARTESIAN_POINT('Ctrl Pts',(-17.4349782765018,35.5330596090706,6.25396999845588));
#63127=CARTESIAN_POINT('Ctrl Pts',(-17.377116641579,35.5284625025259,6.27585242473006));
#63128=CARTESIAN_POINT('Ctrl Pts',(-17.3182505614296,35.523785592814,6.29811471753664));
#63129=CARTESIAN_POINT('Ctrl Pts',(-17.2605235375668,35.5191086831021,6.32367813162913));
#63130=CARTESIAN_POINT('Ctrl Pts',(-17.2043283990451,35.5144317733902,6.3524004470638));
#63131=CARTESIAN_POINT('Ctrl Pts',(-17.149244140679,35.5098473180493,6.38055497227541));
#63132=CARTESIAN_POINT('Ctrl Pts',(-17.0956322288748,35.5052628627085,6.41174440081137));
#63133=CARTESIAN_POINT('Ctrl Pts',(-17.0438433892217,35.5006784073676,6.44578595860873));
#63134=CARTESIAN_POINT('Ctrl Pts',(-16.9920862177114,35.4960967553563,6.47980670047505));
#63135=CARTESIAN_POINT('Ctrl Pts',(-16.9421503324278,35.4915151033451,6.51667583439566));
#63136=CARTESIAN_POINT('Ctrl Pts',(-16.8943598105172,35.4869334513338,6.55616583444497));
#63137=CARTESIAN_POINT('Ctrl Pts',(-16.846580955954,35.482352917865,6.59564619359614));
#63138=CARTESIAN_POINT('Ctrl Pts',(-16.8009468172885,35.4777723843961,6.63774582456135));
#63139=CARTESIAN_POINT('Ctrl Pts',(-16.7577489016525,35.4731918509273,6.68219652796081));
#63140=CARTESIAN_POINT('Ctrl Pts',(-16.7129722924801,35.4684439191367,6.72827170877109));
#63141=CARTESIAN_POINT('Ctrl Pts',(-16.670813872052,35.4636959873461,6.77687275872741));
#63142=CARTESIAN_POINT('Ctrl Pts',(-16.6315551950533,35.4589480555555,6.82766059097233));
#63143=CARTESIAN_POINT('Ctrl Pts',(-16.593632674264,35.4543617180678,6.87671987598634));
#63144=CARTESIAN_POINT('Ctrl Pts',(-16.5584159132772,35.4497753805801,6.92781899746907));
#63145=CARTESIAN_POINT('Ctrl Pts',(-16.526114930877,35.4451890430925,6.98062210428792));
#63146=CARTESIAN_POINT('Ctrl Pts',(-16.4921068167789,35.4403603141504,7.03621589580741));
#63147=CARTESIAN_POINT('Ctrl Pts',(-16.4613315471435,35.4355315852084,7.09369821844355));
#63148=CARTESIAN_POINT('Ctrl Pts',(-16.4339781823525,35.4307028562663,7.1526497543335));
#63149=CARTESIAN_POINT('Ctrl Pts',(-16.4066248175614,35.4258741273242,7.21160129022345));
#63150=CARTESIAN_POINT('Ctrl Pts',(-16.3826935247805,35.4210453983822,7.27202140649802));
#63151=CARTESIAN_POINT('Ctrl Pts',(-16.3623126417182,35.4162166694401,7.33347185865497));
#63152=CARTESIAN_POINT('Ctrl Pts',(-16.3429092942354,35.4116195425503,7.39197494080935));
#63153=CARTESIAN_POINT('Ctrl Pts',(-16.3266438012761,35.4070224156606,7.4516521121725));
#63154=CARTESIAN_POINT('Ctrl Pts',(-16.3136545618917,35.4024252887708,7.51213449943365));
#63155=CARTESIAN_POINT('Ctrl Pts',(-16.3004399023335,35.397748381602,7.57366652092223));
#63156=CARTESIAN_POINT('Ctrl Pts',(-16.2906165525897,35.3930714744333,7.63603149923745));
#63157=CARTESIAN_POINT('Ctrl Pts',(-16.2842780252214,35.3883945672645,7.69882225654889));
#63158=CARTESIAN_POINT('Ctrl Pts',(-16.2780647689407,35.3838100918568,7.76037205267192));
#63159=CARTESIAN_POINT('Ctrl Pts',(-16.2751998980814,35.3792256164491,7.82233042015416));
#63160=CARTESIAN_POINT('Ctrl Pts',(-16.2757200219049,35.3746411410414,7.88430356123687));
#63161=CARTESIAN_POINT('Ctrl Pts',(-16.2762398276636,35.3700594691206,7.94623880466037));
#63162=CARTESIAN_POINT('Ctrl Pts',(-16.2801405193744,35.3654777971997,8.00818829577254));
#63163=CARTESIAN_POINT('Ctrl Pts',(-16.2874066548916,35.3608961252789,8.06975636083683));
#63164=CARTESIAN_POINT('Ctrl Pts',(-16.2946710161991,35.3563155720885,8.13130939250985));
#63165=CARTESIAN_POINT('Ctrl Pts',(-16.3052991303677,35.3517350188981,8.19248067768262));
#63166=CARTESIAN_POINT('Ctrl Pts',(-16.3192237196464,35.3471544657076,8.25287985349837));
#63167=CARTESIAN_POINT('Ctrl Pts',(-16.3336570702856,35.342406553292,8.31548582811055));
#63168=CARTESIAN_POINT('Ctrl Pts',(-16.351632376275,35.3376586408764,8.37726159848694));
#63169=CARTESIAN_POINT('Ctrl Pts',(-16.3730174056464,35.3329107284608,8.43778673553079));
#63170=CARTESIAN_POINT('Ctrl Pts',(-16.3936747725681,35.3283243719411,8.49625240056126));
#63171=CARTESIAN_POINT('Ctrl Pts',(-16.417513263608,35.3237380154214,8.55355072015488));
#63172=CARTESIAN_POINT('Ctrl Pts',(-16.4443645722589,35.3191516589017,8.60932311519822));
#63173=CARTESIAN_POINT('Ctrl Pts',(-16.472634649994,35.3143229685381,8.66804241129839));
#63174=CARTESIAN_POINT('Ctrl Pts',(-16.5042444537181,35.3094942781745,8.72506948723511));
#63175=CARTESIAN_POINT('Ctrl Pts',(-16.5389441911409,35.3046655878109,8.78001812693671));
#63176=CARTESIAN_POINT('Ctrl Pts',(-16.5736439285637,35.2998368974473,8.83496676663832));
#63177=CARTESIAN_POINT('Ctrl Pts',(-16.611433158618,35.2950082070837,8.88783648650567));
#63178=CARTESIAN_POINT('Ctrl Pts',(-16.6520132617444,35.2901795167201,8.9382818254643));
#63179=CARTESIAN_POINT('Ctrl Pts',(-16.6906474407284,35.2855823749341,8.98630817591898));
#63180=CARTESIAN_POINT('Ctrl Pts',(-16.7319696179128,35.280985233148,9.0323346627571));
#63181=CARTESIAN_POINT('Ctrl Pts',(-16.775744901437,35.2763880913619,9.07604497975203));
#63182=CARTESIAN_POINT('Ctrl Pts',(-16.8202797157512,35.2717111860552,9.12051370032366));
#63183=CARTESIAN_POINT('Ctrl Pts',(-16.8673533156068,35.2670342807485,9.16258463764284));
#63184=CARTESIAN_POINT('Ctrl Pts',(-16.9166742887765,35.2623573754417,9.20195843307931));
#63185=CARTESIAN_POINT('Ctrl Pts',(-16.9650206932943,35.2577728844773,9.24055421331711));
#63186=CARTESIAN_POINT('Ctrl Pts',(-17.0155260471576,35.253188393513,9.27655813834427));
#63187=CARTESIAN_POINT('Ctrl Pts',(-17.0678793219735,35.2486039025486,9.30972591291417));
#63188=CARTESIAN_POINT('Ctrl Pts',(-17.120200584247,35.2440222148704,9.34287340633082));
#63189=CARTESIAN_POINT('Ctrl Pts',(-17.1743670978097,35.2394405271922,9.37318791612522));
#63190=CARTESIAN_POINT('Ctrl Pts',(-17.2300380335726,35.234858839514,9.40046786458009));
#63191=CARTESIAN_POINT('Ctrl Pts',(-17.2856953780302,35.2302782703928,9.42774115300485));
#63192=CARTESIAN_POINT('Ctrl Pts',(-17.3428559586453,35.2256977012716,9.4519811268719));
#63193=CARTESIAN_POINT('Ctrl Pts',(-17.401155301161,35.2211171321504,9.47303264165956));
#63194=CARTESIAN_POINT('Ctrl Pts',(-17.4615843191,35.2163692348045,9.49485316844173));
#63195=CARTESIAN_POINT('Ctrl Pts',(-17.5232363810911,35.2116213374587,9.51324752106772));
#63196=CARTESIAN_POINT('Ctrl Pts',(-17.5856865378925,35.2068734401128,9.52809882974473));
#63197=CARTESIAN_POINT('Ctrl Pts',(-17.6460121247443,35.2022870674219,9.54244489318707));
#63198=CARTESIAN_POINT('Ctrl Pts',(-17.7070818399886,35.1977006947309,9.55348510286701));
#63199=CARTESIAN_POINT('Ctrl Pts',(-17.7685031325249,35.19311432204,9.56116643493426));
#63200=CARTESIAN_POINT('Ctrl Pts',(-17.8331691634683,35.1882856623667,9.56925355320603));
#63201=CARTESIAN_POINT('Ctrl Pts',(-17.8982243040283,35.1834570026934,9.57361701714175));
#63202=CARTESIAN_POINT('Ctrl Pts',(-17.9632086098792,35.1786283430201,9.57425728245996));
#63203=CARTESIAN_POINT('Ctrl Pts',(-18.0281929157302,35.1737996833468,9.57489754777817));
#63204=CARTESIAN_POINT('Ctrl Pts',(-18.0931057414124,35.1689710236735,9.57181472283474));
#63205=CARTESIAN_POINT('Ctrl Pts',(-18.1574949088875,35.1641423640002,9.56507238574612));
#63206=CARTESIAN_POINT('Ctrl Pts',(-18.2187953337298,35.1595453347016,9.55865347796752));
#63207=CARTESIAN_POINT('Ctrl Pts',(-18.279873043712,35.1549483054031,9.5488918016507));
#63208=CARTESIAN_POINT('Ctrl Pts',(-18.3403349184589,35.1503512761045,9.53581318944809));
#63209=CARTESIAN_POINT('Ctrl Pts',(-18.4018475377279,35.1456743567369,9.5225072888892));
#63210=CARTESIAN_POINT('Ctrl Pts',(-18.4627221750685,35.1409974373692,9.50576802473026));
#63211=CARTESIAN_POINT('Ctrl Pts',(-18.522549267284,35.1363205180015,9.48567791597507));
#63212=CARTESIAN_POINT('Ctrl Pts',(-18.5811925734696,35.1317361398489,9.46598532595604));
#63213=CARTESIAN_POINT('Ctrl Pts',(-18.6388289058307,35.1271517616964,9.44307345791211));
#63214=CARTESIAN_POINT('Ctrl Pts',(-18.6950843618617,35.1225673835438,9.41707116546747));
#63215=CARTESIAN_POINT('Ctrl Pts',(-18.7513054207461,35.1179858084887,9.39108477200804));
#63216=CARTESIAN_POINT('Ctrl Pts',(-18.8061468163189,35.1134042334336,9.36201191414382));
#63217=CARTESIAN_POINT('Ctrl Pts',(-18.8592543782398,35.1088226583785,9.33002964831067));
#63218=CARTESIAN_POINT('Ctrl Pts',(-18.9123489786251,35.1042422015116,9.2980551881319));
#63219=CARTESIAN_POINT('Ctrl Pts',(-18.9637101494715,35.0996617446447,9.26317299210534));
#63220=CARTESIAN_POINT('Ctrl Pts',(-19.0130099127576,35.0950812877778,9.22560516218571));
#63221=CARTESIAN_POINT('Ctrl Pts',(-19.0641130225915,35.090333281403,9.18666313060915));
#63222=CARTESIAN_POINT('Ctrl Pts',(-19.1130004910849,35.0855852750282,9.14483548314177));
#63223=CARTESIAN_POINT('Ctrl Pts',(-19.159343662819,35.0808372686534,9.10041592990687));
#63224=CARTESIAN_POINT('Ctrl Pts',(-19.2041081261462,35.0762510060112,9.05750955584162));
#63225=CARTESIAN_POINT('Ctrl Pts',(-19.2464985531242,35.0716647433691,9.012185471226));
#63226=CARTESIAN_POINT('Ctrl Pts',(-19.2862575471968,35.067078480727,8.96474474467405));
#63227=CARTESIAN_POINT('Ctrl Pts',(-19.3281198120402,35.0622496024858,8.91479437984195));
#63228=CARTESIAN_POINT('Ctrl Pts',(-19.3670641114359,35.0574207242447,8.86249772431315));
#63229=CARTESIAN_POINT('Ctrl Pts',(-19.4028413932655,35.0525918460035,8.8082415495011));
#63230=CARTESIAN_POINT('Ctrl Pts',(-19.4386186750951,35.0477629677624,8.75398537468905));
#63231=CARTESIAN_POINT('Ctrl Pts',(-19.4712286803328,35.0429340895213,8.6977702819307));
#63232=CARTESIAN_POINT('Ctrl Pts',(-19.5004796218082,35.0381052112801,8.64001075009758));
#63233=CARTESIAN_POINT('Ctrl Pts',(-19.5303734600336,35.0331702007242,8.58098174065393));
#63234=CARTESIAN_POINT('Ctrl Pts',(-19.5568705363577,35.0282351901684,8.52012166857817));
#63235=CARTESIAN_POINT('Ctrl Pts',(-19.5797592626129,35.0233001796125,8.45783087472852));
#63236=CARTESIAN_POINT('Ctrl Pts',(-19.6024236126755,35.0184135465359,8.39615071211298));
#63237=CARTESIAN_POINT('Ctrl Pts',(-19.621549852988,35.0135269134592,8.33306812440386));
#63238=CARTESIAN_POINT('Ctrl Pts',(-19.6369781019475,35.0086402803826,8.26899674844114));
#63239=CARTESIAN_POINT('Ctrl Pts',(-19.6526354595126,35.0036810810871,8.2039739162472));
#63240=CARTESIAN_POINT('Ctrl Pts',(-19.6644838559723,34.9987218817917,8.13793304788255));
#63241=CARTESIAN_POINT('Ctrl Pts',(-19.6724072407195,34.9937626824962,8.07132701547553));
#63242=CARTESIAN_POINT('Ctrl Pts',(-19.6803306254667,34.9888034832007,8.00472098306851));
#63243=CARTESIAN_POINT('Ctrl Pts',(-19.6843288412817,34.9838442839052,7.93755020982685));
#63244=CARTESIAN_POINT('Ctrl Pts',(-19.6843399766484,34.9788850846098,7.87028213160166));
#63245=CARTESIAN_POINT('',(-19.6843394318536,34.1851350845228,7.86860837179767));
#63246=CARTESIAN_POINT('Ctrl Pts',(-19.6843399766485,34.9788850845702,7.87028213106522));
#63247=CARTESIAN_POINT('Ctrl Pts',(-19.6843506246404,34.9741429314013,7.80595813210616));
#63248=CARTESIAN_POINT('Ctrl Pts',(-19.6807154430222,34.9694007782325,7.74168452333965));
#63249=CARTESIAN_POINT('Ctrl Pts',(-19.6734774373292,34.9646586250636,7.67788283560038));
#63250=CARTESIAN_POINT('Ctrl Pts',(-19.6662229716926,34.9599056877676,7.61393605648821));
#63251=CARTESIAN_POINT('Ctrl Pts',(-19.6553493709468,34.9551527504716,7.55046379591763));
#63252=CARTESIAN_POINT('Ctrl Pts',(-19.6409512267573,34.9503998131755,7.48787978601849));
#63253=CARTESIAN_POINT('Ctrl Pts',(-19.6265360234759,34.945641244543,7.42522162584197));
#63254=CARTESIAN_POINT('Ctrl Pts',(-19.6085880846665,34.9408826759105,7.36345425064649));
#63255=CARTESIAN_POINT('Ctrl Pts',(-19.5872517340696,34.936124107278,7.30297557466159));
#63256=CARTESIAN_POINT('Ctrl Pts',(-19.565860394136,34.9313532745739,7.24234102936538));
#63257=CARTESIAN_POINT('Ctrl Pts',(-19.5410633669874,34.9265824418697,7.18300224204036));
#63258=CARTESIAN_POINT('Ctrl Pts',(-19.513052892334,34.9218116091656,7.12533654251973));
#63259=CARTESIAN_POINT('Ctrl Pts',(-19.4939841403159,34.9185637589638,7.08607933828757));
#63260=CARTESIAN_POINT('Ctrl Pts',(-19.473427089533,34.915315908762,7.04759702947158));
#63261=CARTESIAN_POINT('Ctrl Pts',(-19.4514538962117,34.9120680585602,7.01000100760332));
#63262=CARTESIAN_POINT('Ctrl Pts',(-19.4203513175739,34.9074707970321,6.95678465395239));
#63263=CARTESIAN_POINT('Ctrl Pts',(-19.3862942488289,34.902873535504,6.90514851011583));
#63264=CARTESIAN_POINT('Ctrl Pts',(-19.3494682120233,34.8982762739759,6.85544016841895));
#63265=CARTESIAN_POINT('Ctrl Pts',(-19.312004314286,34.893599383637,6.80487083238505));
#63266=CARTESIAN_POINT('Ctrl Pts',(-19.2716747990087,34.888922493298,6.75629722263615));
#63267=CARTESIAN_POINT('Ctrl Pts',(-19.2287235719348,34.884245602959,6.71005850298634));
#63268=CARTESIAN_POINT('Ctrl Pts',(-19.1866197856181,34.879660989087,6.66473208732072));
#63269=CARTESIAN_POINT('Ctrl Pts',(-19.1419971652128,34.8750763752151,6.62164965363058));
#63270=CARTESIAN_POINT('Ctrl Pts',(-19.0951271836689,34.8704917613432,6.58109884015776));
#63271=CARTESIAN_POINT('Ctrl Pts',(-19.0482858525379,34.8659099499276,6.54057281435312));
#63272=CARTESIAN_POINT('Ctrl Pts',(-18.9992002683831,34.8613281385121,6.50257567263456));
#63273=CARTESIAN_POINT('Ctrl Pts',(-18.9481776970915,34.8567463270966,6.46735721494934));
#63274=CARTESIAN_POINT('Ctrl Pts',(-18.8971675750048,34.8521656336159,6.43214735035905));
#63275=CARTESIAN_POINT('Ctrl Pts',(-18.8442218227312,34.8475849401352,6.39971511294401));
#63276=CARTESIAN_POINT('Ctrl Pts',(-18.7896779613946,34.8430042466545,6.37026787910912));
#63277=CARTESIAN_POINT('Ctrl Pts',(-18.7331445635888,34.8382564682533,6.3397465308973));
#63278=CARTESIAN_POINT('Ctrl Pts',(-18.6748947006025,34.8335086898521,6.31243248880869));
#63279=CARTESIAN_POINT('Ctrl Pts',(-18.6153313043008,34.8287609114509,6.28850419874872));
#63280=CARTESIAN_POINT('Ctrl Pts',(-18.5577912669704,34.8241744143167,6.26538874884508));
#63281=CARTESIAN_POINT('Ctrl Pts',(-18.4990260348583,34.8195879171825,6.24543280049305));
#63282=CARTESIAN_POINT('Ctrl Pts',(-18.4394160071978,34.8150014200483,6.22874689096094));
#63283=CARTESIAN_POINT('Ctrl Pts',(-18.3766617562319,34.8101730010136,6.21118085726711));
#63284=CARTESIAN_POINT('Ctrl Pts',(-18.3129717504518,34.8053445819789,6.19723952836195));
#63285=CARTESIAN_POINT('Ctrl Pts',(-18.248800852578,34.8005161629442,6.18699051183503));
#63286=CARTESIAN_POINT('Ctrl Pts',(-18.1846299547043,34.7956877439096,6.17674149530811));
#63287=CARTESIAN_POINT('Ctrl Pts',(-18.1199788188343,34.7908593248749,6.17018477954102));
#63288=CARTESIAN_POINT('Ctrl Pts',(-18.0553039694653,34.7860309058402,6.16732441499187));
#63289=CARTESIAN_POINT('Ctrl Pts',(-17.9937365055766,34.7814344743454,6.16460148029923));
#63290=CARTESIAN_POINT('Ctrl Pts',(-17.9318944866733,34.7768380428507,6.16521660012749));
#63291=CARTESIAN_POINT('Ctrl Pts',(-17.870170437177,34.7722416113559,6.16920245098657));
#63292=CARTESIAN_POINT('Ctrl Pts',(-17.8073645375938,34.7675646172628,6.1732581626719));
#63293=CARTESIAN_POINT('Ctrl Pts',(-17.7446813086675,34.7628876231696,6.18080402050468));
#63294=CARTESIAN_POINT('Ctrl Pts',(-17.6825381119754,34.7582106290764,6.19181906196834));
#63295=CARTESIAN_POINT('Ctrl Pts',(-17.6216334537591,34.7536268493244,6.20261456930127));
#63296=CARTESIAN_POINT('Ctrl Pts',(-17.561248025304,34.7490430695724,6.21674215214675));
#63297=CARTESIAN_POINT('Ctrl Pts',(-17.5017706035719,34.7444592898204,6.2341297484238));
#63298=CARTESIAN_POINT('Ctrl Pts',(-17.442329535482,34.7398783117549,6.25150671709735));
#63299=CARTESIAN_POINT('Ctrl Pts',(-17.3837958614369,34.7352973336894,6.2721396056733));
#63300=CARTESIAN_POINT('Ctrl Pts',(-17.3265459798054,34.7307163556238,6.29590575914542));
#63301=CARTESIAN_POINT('Ctrl Pts',(-17.2693100430223,34.7261364933867,6.31966612369019));
#63302=CARTESIAN_POINT('Ctrl Pts',(-17.2133577480129,34.7215566311496,6.34655804293153));
#63303=CARTESIAN_POINT('Ctrl Pts',(-17.1590462563224,34.7169767689125,6.37641043578171));
#63304=CARTESIAN_POINT('Ctrl Pts',(-17.1027339258694,34.7122281842631,6.4073625926581));
#63305=CARTESIAN_POINT('Ctrl Pts',(-17.04818619406,34.7074795996138,6.44149738242054));
#63306=CARTESIAN_POINT('Ctrl Pts',(-16.9957717532147,34.7027310149644,6.47857282122635));
#63307=CARTESIAN_POINT('Ctrl Pts',(-16.9451554313795,34.6981453342818,6.51437635766619));
#63308=CARTESIAN_POINT('Ctrl Pts',(-16.8965287638021,34.6935596535992,6.55292165238522));
#63309=CARTESIAN_POINT('Ctrl Pts',(-16.8501907821988,34.6889739729166,6.59394907351958));
#63310=CARTESIAN_POINT('Ctrl Pts',(-16.8013836008616,34.6841439362838,6.63716271196092));
#63311=CARTESIAN_POINT('Ctrl Pts',(-16.7551163052492,34.6793138996511,6.68312995311512));
#63312=CARTESIAN_POINT('Ctrl Pts',(-16.711692661252,34.6744838630183,6.73150479575973));
#63313=CARTESIAN_POINT('Ctrl Pts',(-16.6682690172549,34.6696538263856,6.77987963840435));
#63314=CARTESIAN_POINT('Ctrl Pts',(-16.6276893705955,34.6648237897529,6.83066152487718));
#63315=CARTESIAN_POINT('Ctrl Pts',(-16.5902048672717,34.6599937531201,6.88346853844153));
#63316=CARTESIAN_POINT('Ctrl Pts',(-16.554520903842,34.6553957236604,6.93373900686912));
#63317=CARTESIAN_POINT('Ctrl Pts',(-16.521494791712,34.6507976942006,6.98605115161277));
#63318=CARTESIAN_POINT('Ctrl Pts',(-16.4913668687188,34.6461996647409,7.04009263405372));
#63319=CARTESIAN_POINT('Ctrl Pts',(-16.4607228501906,34.6415228703933,7.09505985464775));
#63320=CARTESIAN_POINT('Ctrl Pts',(-16.4330776327838,34.6368460760458,7.15181584110059));
#63321=CARTESIAN_POINT('Ctrl Pts',(-16.4086397103088,34.6321692816983,7.2099987306213));
#63322=CARTESIAN_POINT('Ctrl Pts',(-16.3846795378917,34.6275839165127,7.26704417161848));
#63323=CARTESIAN_POINT('Ctrl Pts',(-16.3638025931529,34.622998551327,7.32546073552173));
#63324=CARTESIAN_POINT('Ctrl Pts',(-16.3461591813918,34.6184131861414,7.38488247295153));
#63325=CARTESIAN_POINT('Ctrl Pts',(-16.3285265842987,34.6138306315914,7.44426778735998));
#63326=CARTESIAN_POINT('Ctrl Pts',(-16.3141237346164,34.6092480770414,7.50465656678885));
#63327=CARTESIAN_POINT('Ctrl Pts',(-16.3030517150819,34.6046655224915,7.56566583282496));
#63328=CARTESIAN_POINT('Ctrl Pts',(-16.2919824191085,34.6000840951855,7.62666009143899));
#63329=CARTESIAN_POINT('Ctrl Pts',(-16.2842424175926,34.5955026678796,7.6882740332079));
#63330=CARTESIAN_POINT('Ctrl Pts',(-16.2798816739943,34.5909212405736,7.75011458312333));
#63331=CARTESIAN_POINT('Ctrl Pts',(-16.2753632824288,34.5861741872258,7.81419076940771));
#63332=CARTESIAN_POINT('Ctrl Pts',(-16.2744732661424,34.581427133878,7.87850968701966));
#63333=CARTESIAN_POINT('Ctrl Pts',(-16.2772082986786,34.5766800805303,7.94263096798809));
#63334=CARTESIAN_POINT('Ctrl Pts',(-16.2798512308894,34.5720928809143,8.00459300925585));
#63335=CARTESIAN_POINT('Ctrl Pts',(-16.2858788120345,34.5675056812983,8.06636999537276));
#63336=CARTESIAN_POINT('Ctrl Pts',(-16.2952351180072,34.5629184816823,8.1275696566054));
#63337=CARTESIAN_POINT('Ctrl Pts',(-16.305080493745,34.5580915014686,8.19196832650925));
#63338=CARTESIAN_POINT('Ctrl Pts',(-16.3186120185535,34.5532645212549,8.25572702750474));
#63339=CARTESIAN_POINT('Ctrl Pts',(-16.3357041636109,34.5484375410413,8.31840387825416));
#63340=CARTESIAN_POINT('Ctrl Pts',(-16.3527963086682,34.5436105608276,8.38108072900357));
#63341=CARTESIAN_POINT('Ctrl Pts',(-16.3734487949792,34.5387835806139,8.44267513964444));
#63342=CARTESIAN_POINT('Ctrl Pts',(-16.3974775887123,34.5339566004002,8.50276982653415));
#63343=CARTESIAN_POINT('Ctrl Pts',(-16.4203658458407,34.5293587347932,8.56001209432588));
#63344=CARTESIAN_POINT('Ctrl Pts',(-16.4464107655711,34.5247608691861,8.61612806925893));
#63345=CARTESIAN_POINT('Ctrl Pts',(-16.4754801685045,34.5201630035791,8.67074647188537));
#63346=CARTESIAN_POINT('Ctrl Pts',(-16.5050487175514,34.51548618875,8.72630271845209));
#63347=CARTESIAN_POINT('Ctrl Pts',(-16.5377464870054,34.5108093739208,8.78030895071487));
#63348=CARTESIAN_POINT('Ctrl Pts',(-16.5733823977776,34.5061325590917,8.83239376386073));
#63349=CARTESIAN_POINT('Ctrl Pts',(-16.6083205706582,34.5015473145592,8.88345877571848));
#63350=CARTESIAN_POINT('Ctrl Pts',(-16.6460825651465,34.4969620700266,8.93267649162326));
#63351=CARTESIAN_POINT('Ctrl Pts',(-16.6864423443792,34.4923768254941,8.9797222297426));
#63352=CARTESIAN_POINT('Ctrl Pts',(-16.7267775270666,34.4877943753568,9.02673929667849));
#63353=CARTESIAN_POINT('Ctrl Pts',(-16.7697070246047,34.4832119252195,9.07158662508624));
#63354=CARTESIAN_POINT('Ctrl Pts',(-16.814963808604,34.4786294750822,9.11397166701559));
#63355=CARTESIAN_POINT('Ctrl Pts',(-16.8602096204161,34.4740481359276,9.15634643299131));
#63356=CARTESIAN_POINT('Ctrl Pts',(-16.9077812273287,34.4694667967729,9.19625974987497));
#63357=CARTESIAN_POINT('Ctrl Pts',(-16.9573754072449,34.4648854576182,9.23345655519069));
#63358=CARTESIAN_POINT('Ctrl Pts',(-17.0087647217844,34.4601382901234,9.27199975383744));
#63359=CARTESIAN_POINT('Ctrl Pts',(-17.0623254112357,34.4553911226285,9.30762561239995));
#63360=CARTESIAN_POINT('Ctrl Pts',(-17.1176855824613,34.4506439551337,9.34009818750481));
#63361=CARTESIAN_POINT('Ctrl Pts',(-17.1711797008059,34.4460568027794,9.37147619333745));
#63362=CARTESIAN_POINT('Ctrl Pts',(-17.2263534091185,34.4414696504252,9.39990994792744));
#63363=CARTESIAN_POINT('Ctrl Pts',(-17.2828467641579,34.4368824980709,9.42523380922449));
#63364=CARTESIAN_POINT('Ctrl Pts',(-17.3422961335553,34.4320553230058,9.45188274136469));
#63365=CARTESIAN_POINT('Ctrl Pts',(-17.4032064466867,34.4272281479407,9.47508714952236));
#63366=CARTESIAN_POINT('Ctrl Pts',(-17.4651382813054,34.4224009728756,9.49471297348881));
#63367=CARTESIAN_POINT('Ctrl Pts',(-17.5270701159241,34.4175737978104,9.51433879745526));
#63368=CARTESIAN_POINT('Ctrl Pts',(-17.5900228249264,34.4127466227453,9.53038595207365));
#63369=CARTESIAN_POINT('Ctrl Pts',(-17.6535459491956,34.4079194476802,9.5427828873806));
#63370=CARTESIAN_POINT('Ctrl Pts',(-17.713973200144,34.4033275306045,9.55457564363122));
#63371=CARTESIAN_POINT('Ctrl Pts',(-17.7751660974045,34.3987356135289,9.56311443212996));
#63372=CARTESIAN_POINT('Ctrl Pts',(-17.8367420124595,34.3941436964532,9.56830856578122));
#63373=CARTESIAN_POINT('Ctrl Pts',(-17.8994663460402,34.3894661380576,9.57359957236249));
#63374=CARTESIAN_POINT('Ctrl Pts',(-17.9625876258848,34.3847885796621,9.57541969358361));
#63375=CARTESIAN_POINT('Ctrl Pts',(-18.0256893124278,34.3801110212666,9.57372747889147));
#63376=CARTESIAN_POINT('Ctrl Pts',(-18.0874648290596,34.3755317682816,9.57207082845016));
#63377=CARTESIAN_POINT('Ctrl Pts',(-18.1492210311112,34.3709525152966,9.56704805752778));
#63378=CARTESIAN_POINT('Ctrl Pts',(-18.2105633826536,34.3663732623116,9.55867266282704));
#63379=CARTESIAN_POINT('Ctrl Pts',(-18.2718683053278,34.36179680342,9.550302378487));
#63380=CARTESIAN_POINT('Ctrl Pts',(-18.3327593735459,34.3572203445283,9.53858359511074));
#63381=CARTESIAN_POINT('Ctrl Pts',(-18.3928467801605,34.3526438856367,9.52358167978213));
#63382=CARTESIAN_POINT('Ctrl Pts',(-18.4529197289901,34.3480685278985,9.50858337410284));
#63383=CARTESIAN_POINT('Ctrl Pts',(-18.5121889051227,34.3434931701604,9.49030362811654));
#63384=CARTESIAN_POINT('Ctrl Pts',(-18.5702763487881,34.3389178124222,9.46885855148645));
#63385=CARTESIAN_POINT('Ctrl Pts',(-18.6306185776935,34.3341648526337,9.44658103949334));
#63386=CARTESIAN_POINT('Ctrl Pts',(-18.6896848739899,34.3294118928452,9.42088755978668));
#63387=CARTESIAN_POINT('Ctrl Pts',(-18.7470731927272,34.3246589330567,9.39196371592734));
#63388=CARTESIAN_POINT('Ctrl Pts',(-18.8023884161351,34.3200776691631,9.36408471685403));
#63389=CARTESIAN_POINT('Ctrl Pts',(-18.8561444038319,34.3154964052694,9.33320509228768));
#63390=CARTESIAN_POINT('Ctrl Pts',(-18.9080076521529,34.3109151413757,9.29953720943028));
#63391=CARTESIAN_POINT('Ctrl Pts',(-18.9599081636949,34.3063305858901,9.2658451365385));
#63392=CARTESIAN_POINT('Ctrl Pts',(-19.0099128202455,34.3017460304045,9.22936112250298));
#63393=CARTESIAN_POINT('Ctrl Pts',(-19.0577198226825,34.2971614749189,9.19033890323557));
#63394=CARTESIAN_POINT('Ctrl Pts',(-19.1056072871779,34.2925692033509,9.15125100722773));
#63395=CARTESIAN_POINT('Ctrl Pts',(-19.1512893491688,34.2879769317829,9.10961673335924));
#63396=CARTESIAN_POINT('Ctrl Pts',(-19.1945007774973,34.2833846602149,9.06572684884901));
#63397=CARTESIAN_POINT('Ctrl Pts',(-19.1992129950831,34.2828838717966,9.06094064543879));
#63398=CARTESIAN_POINT('Ctrl Pts',(-19.2038958721242,34.2823830833784,9.05612764994006));
#63399=CARTESIAN_POINT('Ctrl Pts',(-19.2085490945638,34.2818822949602,9.05128826196086));
#63400=CARTESIAN_POINT('Ctrl Pts',(-19.2507977189333,34.2773354197475,9.00734935992727));
#63401=CARTESIAN_POINT('Ctrl Pts',(-19.2907820667709,34.2727885445347,8.9610410817571));
#63402=CARTESIAN_POINT('Ctrl Pts',(-19.3282210877398,34.268241669322,8.91262876143603));
#63403=CARTESIAN_POINT('Ctrl Pts',(-19.3656073664394,34.2637011995256,8.86428464203401));
#63404=CARTESIAN_POINT('Ctrl Pts',(-19.4004551043781,34.2591607297292,8.81384275911745));
#63405=CARTESIAN_POINT('Ctrl Pts',(-19.4325205974813,34.2546202599328,8.76160459257042));
#63406=CARTESIAN_POINT('Ctrl Pts',(-19.4645533250525,34.2500844297316,8.70941980462916));
#63407=CARTESIAN_POINT('Ctrl Pts',(-19.4938091701776,34.2455485995304,8.65544281204892));
#63408=CARTESIAN_POINT('Ctrl Pts',(-19.5200865495544,34.2410127693292,8.60000565441758));
#63409=CARTESIAN_POINT('Ctrl Pts',(-19.5470628518699,34.2363562955993,8.54309398517029));
#63410=CARTESIAN_POINT('Ctrl Pts',(-19.5708996400718,34.2316998218694,8.48464382257598));
#63411=CARTESIAN_POINT('Ctrl Pts',(-19.5914290092486,34.2270433481395,8.42504178559117));
#63412=CARTESIAN_POINT('Ctrl Pts',(-19.6114150615545,34.2225101096007,8.36701713717319));
#63413=CARTESIAN_POINT('Ctrl Pts',(-19.6282664798948,34.217976871062,8.30790136813938));
#63414=CARTESIAN_POINT('Ctrl Pts',(-19.6418780073849,34.2134436325233,8.24806920553037));
#63415=CARTESIAN_POINT('Ctrl Pts',(-19.6560445748906,34.2087255411978,8.18579725469854));
#63416=CARTESIAN_POINT('Ctrl Pts',(-19.6667011420569,34.2040074498723,8.1227498077348));
#63417=CARTESIAN_POINT('Ctrl Pts',(-19.673787848891,34.1992893585467,8.05936092138871));
#63418=CARTESIAN_POINT('Ctrl Pts',(-19.6808745557251,34.1945712672212,7.99597203504263));
#63419=CARTESIAN_POINT('Ctrl Pts',(-19.6843913902768,34.1898531758957,7.93224234397999));
#63420=CARTESIAN_POINT('Ctrl Pts',(-19.6843394318541,34.1851350845702,7.86860837243737));
#63421=CARTESIAN_POINT('',(-18.5338892852531,34.0285,6.25817448361128));
#63422=CARTESIAN_POINT('Ctrl Pts',(-19.6843394318536,34.1851350845228,7.86860837179767));
#63423=CARTESIAN_POINT('Ctrl Pts',(-19.6842719233823,34.1790049718436,7.78593014688382));
#63424=CARTESIAN_POINT('Ctrl Pts',(-19.6781845294511,34.1728748591644,7.70351110997361));
#63425=CARTESIAN_POINT('Ctrl Pts',(-19.6662118452382,34.1667447464852,7.62207975359352));
#63426=CARTESIAN_POINT('Ctrl Pts',(-19.6591158625868,34.1631115450702,7.57381693450569));
#63427=CARTESIAN_POINT('Ctrl Pts',(-19.649953449709,34.1594783436552,7.5259004991251));
#63428=CARTESIAN_POINT('Ctrl Pts',(-19.6387602520471,34.1558451422402,7.47847827412956));
#63429=CARTESIAN_POINT('Ctrl Pts',(-19.6245873402614,34.1512447550488,7.41843189311805));
#63430=CARTESIAN_POINT('Ctrl Pts',(-19.607121248674,34.1466443678575,7.35903532165387));
#63431=CARTESIAN_POINT('Ctrl Pts',(-19.5864384974648,34.1420439806661,7.30067567286909));
#63432=CARTESIAN_POINT('Ctrl Pts',(-19.5654135544815,34.137367481035,7.24135047595436));
#63433=CARTESIAN_POINT('Ctrl Pts',(-19.5410645761215,34.1326909814039,7.18309736177195));
#63434=CARTESIAN_POINT('Ctrl Pts',(-19.5135260599372,34.1280144817729,7.12631145020672));
#63435=CARTESIAN_POINT('Ctrl Pts',(-19.4865088438649,34.1234265076006,7.07060048770063));
#63436=CARTESIAN_POINT('Ctrl Pts',(-19.4564220270362,34.1188385334284,7.01630214098928));
#63437=CARTESIAN_POINT('Ctrl Pts',(-19.4234417677024,34.1142505592562,6.96377116639769));
#63438=CARTESIAN_POINT('Ctrl Pts',(-19.3904811002752,34.1096653105678,6.91127139780543));
#63439=CARTESIAN_POINT('Ctrl Pts',(-19.354630668445,34.1050800618793,6.86053734884721));
#63440=CARTESIAN_POINT('Ctrl Pts',(-19.3161118896715,34.1004948131909,6.8118979945778));
#63441=CARTESIAN_POINT('Ctrl Pts',(-19.2776019099619,34.0959106119369,6.76326975127296));
#63442=CARTESIAN_POINT('Ctrl Pts',(-19.2364251088108,34.091326410683,6.71673565079938));
#63443=CARTESIAN_POINT('Ctrl Pts',(-19.192844206647,34.086742209429,6.67259289880058));
#63444=CARTESIAN_POINT('Ctrl Pts',(-19.1477392085214,34.0819976911032,6.62690640202541));
#63445=CARTESIAN_POINT('Ctrl Pts',(-19.1000592002055,34.0772531727775,6.58378207147794));
#63446=CARTESIAN_POINT('Ctrl Pts',(-19.0501364505395,34.0725086544518,6.54350732650842));
#63447=CARTESIAN_POINT('Ctrl Pts',(-19.0018381420728,34.0679185184686,6.50454308537656));
#63448=CARTESIAN_POINT('Ctrl Pts',(-18.9514412861617,34.0633283824854,6.46824606480622));
#63449=CARTESIAN_POINT('Ctrl Pts',(-18.8992778243817,34.0587382465022,6.43483341830988));
#63450=CARTESIAN_POINT('Ctrl Pts',(-18.8444827028466,34.0539165370052,6.39973509540149));
#63451=CARTESIAN_POINT('Ctrl Pts',(-18.7877385472706,34.0490948275082,6.36782022212208));
#63452=CARTESIAN_POINT('Ctrl Pts',(-18.7294583783504,34.0442731180112,6.33928546922675));
#63453=CARTESIAN_POINT('Ctrl Pts',(-18.6711782094302,34.0394514085142,6.31075071633142));
#63454=CARTESIAN_POINT('Ctrl Pts',(-18.6113626481108,34.0346296990172,6.28559626162566));
#63455=CARTESIAN_POINT('Ctrl Pts',(-18.5504447240674,34.0298079895202,6.26395901285688));
#63456=CARTESIAN_POINT('Ctrl Pts',(-18.5449363038492,34.0293719930134,6.26200249414));
#63457=CARTESIAN_POINT('Ctrl Pts',(-18.5394177624311,34.0289359965067,6.26007429487589));
#63458=CARTESIAN_POINT('Ctrl Pts',(-18.5338892852531,34.0285,6.25817448361128));
#63459=CARTESIAN_POINT('',(-19.6230207093981,34.0285,7.41694615762715));
#63460=CARTESIAN_POINT('Origin',(-17.98,34.0285,7.87));
#63461=CARTESIAN_POINT('',(-19.6817804353622,34.0624899145464,7.87021334420357));
#63462=CARTESIAN_POINT('Ctrl Pts',(-19.6230207093982,34.0285,7.41694615762719));
#63463=CARTESIAN_POINT('Ctrl Pts',(-19.6439594234565,34.0343385372865,7.49288137240387));
#63464=CARTESIAN_POINT('Ctrl Pts',(-19.6596181661918,34.040177074573,7.57022718668484));
#63465=CARTESIAN_POINT('Ctrl Pts',(-19.6698639770707,34.0460156118594,7.64833679917736));
#63466=CARTESIAN_POINT('Ctrl Pts',(-19.6795006474282,34.0515070326815,7.72180258887821));
#63467=CARTESIAN_POINT('Ctrl Pts',(-19.6843492737208,34.0569984535036,7.79594416842021));
#63468=CARTESIAN_POINT('Ctrl Pts',(-19.684339986675,34.0624898743257,7.87021312113508));
#63469=CARTESIAN_POINT('',(-19.6836712649746,34.8562399466723,7.87062608132905));
#63470=CARTESIAN_POINT('Ctrl Pts',(-19.6817242086285,34.0624899154299,7.87021334910381));
#63471=CARTESIAN_POINT('Ctrl Pts',(-19.6788237970149,34.0931723278599,8.28454169889619));
#63472=CARTESIAN_POINT('Ctrl Pts',(-19.32074390439,34.1658671245298,9.26764861307284));
#63473=CARTESIAN_POINT('Ctrl Pts',(-17.6674941309001,34.2805743054401,9.86139173961966));
#63474=CARTESIAN_POINT('Ctrl Pts',(-16.1387855091513,34.40661145816,8.68643802656981));
#63475=CARTESIAN_POINT('Ctrl Pts',(-16.2948985422798,34.53264861088,6.76609642493242));
#63476=CARTESIAN_POINT('Ctrl Pts',(-17.9941440978388,34.6586857636,5.85535067860367));
#63477=CARTESIAN_POINT('Ctrl Pts',(-19.4371160993711,34.7665495317833,6.65484857269287));
#63478=CARTESIAN_POINT('Ctrl Pts',(-19.6807260588958,34.8324009157266,7.5478711651106));
#63479=CARTESIAN_POINT('Ctrl Pts',(-19.6817736577327,34.8562399154299,7.87062496082499));
#63480=CARTESIAN_POINT('',(-19.6843395660614,35.6499899153767,7.87121620626328));
#63481=CARTESIAN_POINT('Ctrl Pts',(-19.6843398848609,34.8562399576805,7.87062647613745));
#63482=CARTESIAN_POINT('Ctrl Pts',(-19.6843151234373,34.8612080553341,7.93799038569272));
#63483=CARTESIAN_POINT('Ctrl Pts',(-19.6802923106048,34.8661761529877,8.0052332769274));
#63484=CARTESIAN_POINT('Ctrl Pts',(-19.672339476806,34.8711442506413,8.07189584157179));
#63485=CARTESIAN_POINT('Ctrl Pts',(-19.6643644321827,34.8761262232918,8.13874458268597));
#63486=CARTESIAN_POINT('Ctrl Pts',(-19.6524375222774,34.8811081959424,8.20500940461969));
#63487=CARTESIAN_POINT('Ctrl Pts',(-19.6366776310176,34.886090168593,8.27024250459691));
#63488=CARTESIAN_POINT('Ctrl Pts',(-19.620850813758,34.891093297703,8.33575262364476));
#63489=CARTESIAN_POINT('Ctrl Pts',(-19.6011585501973,34.8960964268129,8.40022190399817));
#63490=CARTESIAN_POINT('Ctrl Pts',(-19.5777696675149,34.9010995559229,8.46321743498425));
#63491=CARTESIAN_POINT('Ctrl Pts',(-19.5627158479965,34.904319726962,8.50376333736041));
#63492=CARTESIAN_POINT('Ctrl Pts',(-19.5461316374502,34.907539898001,8.54369915558196));
#63493=CARTESIAN_POINT('Ctrl Pts',(-19.5280720831781,34.91076006904,8.58291490437828));
#63494=CARTESIAN_POINT('Ctrl Pts',(-19.5022938886773,34.9153565388155,8.63889143540082));
#63495=CARTESIAN_POINT('Ctrl Pts',(-19.4734226123672,34.9199530085909,8.69358328884918));
#63496=CARTESIAN_POINT('Ctrl Pts',(-19.4416089489638,34.9245494783663,8.74662655441696));
#63497=CARTESIAN_POINT('Ctrl Pts',(-19.4092379836671,34.9292264676744,8.80059901546763));
#63498=CARTESIAN_POINT('Ctrl Pts',(-19.3738206871155,34.9339034569825,8.85286405197072));
#63499=CARTESIAN_POINT('Ctrl Pts',(-19.3355668076366,34.9385804462905,8.90306024298394));
#63500=CARTESIAN_POINT('Ctrl Pts',(-19.2980751762118,34.9431642417566,8.95225622305252));
#63501=CARTESIAN_POINT('Ctrl Pts',(-19.2578592916959,34.9477480372227,8.99946462368427));
#63502=CARTESIAN_POINT('Ctrl Pts',(-19.2151612444391,34.9523318326888,9.04437282659111));
#63503=CARTESIAN_POINT('Ctrl Pts',(-19.1724893732809,34.9569128180525,9.08925349846036));
#63504=CARTESIAN_POINT('Ctrl Pts',(-19.1273387067944,34.9614938034163,9.13183640037992));
#63505=CARTESIAN_POINT('Ctrl Pts',(-19.0799906443404,34.96607478878,9.17184308500047));
#63506=CARTESIAN_POINT('Ctrl Pts',(-19.0326542016859,34.9706546499134,9.21183995148637));
#63507=CARTESIAN_POINT('Ctrl Pts',(-18.9831218223752,34.9752345110467,9.24926152721103));
#63508=CARTESIAN_POINT('Ctrl Pts',(-18.931709148148,34.9798143721801,9.283868640621));
#63509=CARTESIAN_POINT('Ctrl Pts',(-18.8784025704177,34.9845629429784,9.31975058624508));
#63510=CARTESIAN_POINT('Ctrl Pts',(-18.8230749130192,34.9893115137768,9.35260629089814));
#63511=CARTESIAN_POINT('Ctrl Pts',(-18.7661101301898,34.9940600845751,9.38221879991389));
#63512=CARTESIAN_POINT('Ctrl Pts',(-18.7110996723638,34.9986457433042,9.41081537480491));
#63513=CARTESIAN_POINT('Ctrl Pts',(-18.6545631187334,35.0032314020333,9.43638754236675));
#63514=CARTESIAN_POINT('Ctrl Pts',(-18.5968682145621,35.0078170607625,9.45878835640968));
#63515=CARTESIAN_POINT('Ctrl Pts',(-18.5360987697057,35.0126470875954,9.48238290177329));
#63516=CARTESIAN_POINT('Ctrl Pts',(-18.4740446787157,35.0174771144283,9.50245843256857));
#63517=CARTESIAN_POINT('Ctrl Pts',(-18.4111526444799,35.0223071412612,9.51890334245462));
#63518=CARTESIAN_POINT('Ctrl Pts',(-18.3482606102441,35.0271371680942,9.53534825234067));
#63519=CARTESIAN_POINT('Ctrl Pts',(-18.2845312868417,35.0319671949271,9.54816248925614));
#63520=CARTESIAN_POINT('Ctrl Pts',(-18.2204192144078,35.03679722176,9.55729767289105));
#63521=CARTESIAN_POINT('Ctrl Pts',(-18.1593967423115,35.041394486619,9.56599262638878));
#63522=CARTESIAN_POINT('Ctrl Pts',(-18.0977766951745,35.0459917514779,9.57139077173162));
#63523=CARTESIAN_POINT('Ctrl Pts',(-18.0359466975418,35.0505890163369,9.57342149881765));
#63524=CARTESIAN_POINT('Ctrl Pts',(-17.9730457984822,35.0552659062595,9.57548739828953));
#63525=CARTESIAN_POINT('Ctrl Pts',(-17.909928118726,35.0599427961822,9.57406795243933));
#63526=CARTESIAN_POINT('Ctrl Pts',(-17.8470109542982,35.0646196861048,9.5691435340557));
#63527=CARTESIAN_POINT('Ctrl Pts',(-17.7853351396093,35.069204301429,9.56431627398382));
#63528=CARTESIAN_POINT('Ctrl Pts',(-17.7238525319013,35.0737889167531,9.55612113212566));
#63529=CARTESIAN_POINT('Ctrl Pts',(-17.6629571844191,35.0783735320773,9.54459209620986));
#63530=CARTESIAN_POINT('Ctrl Pts',(-17.6020990699957,35.0829553442439,9.53307010945774));
#63531=CARTESIAN_POINT('Ctrl Pts',(-17.5418280029354,35.0875371564105,9.51821836506025));
#63532=CARTESIAN_POINT('Ctrl Pts',(-17.4825306284952,35.0921189685771,9.50012240645132));
#63533=CARTESIAN_POINT('Ctrl Pts',(-17.4232477313223,35.0966996621088,9.48203086591371));
#63534=CARTESIAN_POINT('Ctrl Pts',(-17.3649385415053,35.1012803556404,9.46069683204308));
#63535=CARTESIAN_POINT('Ctrl Pts',(-17.3079752627805,35.105861049172,9.43625591400802));
#63536=CARTESIAN_POINT('Ctrl Pts',(-17.2489342138832,35.110608826281,9.41092349865015));
#63537=CARTESIAN_POINT('Ctrl Pts',(-17.1913397195808,35.11535660339,9.38225333882373));
#63538=CARTESIAN_POINT('Ctrl Pts',(-17.1355819578834,35.120104380499,9.35045027128507));
#63539=CARTESIAN_POINT('Ctrl Pts',(-17.0817182835261,35.1246908759453,9.31972755176912));
#63540=CARTESIAN_POINT('Ctrl Pts',(-17.0295689526653,35.1292773713916,9.28608172025399));
#63541=CARTESIAN_POINT('Ctrl Pts',(-16.9794569339345,35.1338638668379,9.24974215292145));
#63542=CARTESIAN_POINT('Ctrl Pts',(-16.9267016716432,35.1386922847782,9.2114857933746));
#63543=CARTESIAN_POINT('Ctrl Pts',(-16.8762051016778,35.1435207027186,9.17024405891093));
#63544=CARTESIAN_POINT('Ctrl Pts',(-16.828302823352,35.1483491206589,9.12633134518765));
#63545=CARTESIAN_POINT('Ctrl Pts',(-16.7804005450262,35.1531775385993,9.08241863146438));
#63546=CARTESIAN_POINT('Ctrl Pts',(-16.7350929556611,35.1580059565396,9.03583545820782));
#63547=CARTESIAN_POINT('Ctrl Pts',(-16.6926668877745,35.16283437448,8.98693701423482));
#63548=CARTESIAN_POINT('Ctrl Pts',(-16.6522724599837,35.1674315759071,8.94038015043522));
#63549=CARTESIAN_POINT('Ctrl Pts',(-16.6143239782576,35.1720287773342,8.89153356176056));
#63550=CARTESIAN_POINT('Ctrl Pts',(-16.5790909528396,35.1766259787614,8.84068464352961));
#63551=CARTESIAN_POINT('Ctrl Pts',(-16.5432471327471,35.181302876613,8.78895421574631));
#63552=CARTESIAN_POINT('Ctrl Pts',(-16.5102142347303,35.1859797744646,8.73515171132269));
#63553=CARTESIAN_POINT('Ctrl Pts',(-16.4802350318256,35.1906566723162,8.67961711681319));
#63554=CARTESIAN_POINT('Ctrl Pts',(-16.4508477515244,35.195241227434,8.62517902182931));
#63555=CARTESIAN_POINT('Ctrl Pts',(-16.4243949291801,35.1998257825519,8.56907708288993));
#63556=CARTESIAN_POINT('Ctrl Pts',(-16.4010616749758,35.2044103376697,8.51166081489345));
#63557=CARTESIAN_POINT('Ctrl Pts',(-16.3777426805329,35.2089920910068,8.454279635971));
#63558=CARTESIAN_POINT('Ctrl Pts',(-16.3575396652213,35.2135738443439,8.39558619130295));
#63559=CARTESIAN_POINT('Ctrl Pts',(-16.3405904038642,35.218155597681,8.33595172678911));
#63560=CARTESIAN_POINT('Ctrl Pts',(-16.323645275198,35.222736233862,8.27633180278007));
#63561=CARTESIAN_POINT('Ctrl Pts',(-16.3099524646705,35.227316870043,8.215771803851));
#63562=CARTESIAN_POINT('Ctrl Pts',(-16.2995998497716,35.231897506224,8.15465798901892));
#63563=CARTESIAN_POINT('Ctrl Pts',(-16.2888693515922,35.2366453413053,8.0913134441677));
#63564=CARTESIAN_POINT('Ctrl Pts',(-16.2817277674087,35.2413931763867,8.02737443498475));
#63565=CARTESIAN_POINT('Ctrl Pts',(-16.2782145559828,35.246141011468,7.96327989135553));
#63566=CARTESIAN_POINT('Ctrl Pts',(-16.2748207687374,35.2507274539531,7.90136410596504));
#63567=CARTESIAN_POINT('Ctrl Pts',(-16.2748125482068,35.2553138964382,7.83930371930836));
#63568=CARTESIAN_POINT('Ctrl Pts',(-16.2781722879367,35.2599003389234,7.77749446474163));
#63569=CARTESIAN_POINT('Ctrl Pts',(-16.2817093667871,35.2647288703028,7.712422695896));
#63570=CARTESIAN_POINT('Ctrl Pts',(-16.2889797411147,35.2695574016822,7.64762994774134));
#63571=CARTESIAN_POINT('Ctrl Pts',(-16.2999012076079,35.2743859330617,7.58356871085268));
#63572=CARTESIAN_POINT('Ctrl Pts',(-16.3108226741011,35.2792144644411,7.51950747396401));
#63573=CARTESIAN_POINT('Ctrl Pts',(-16.3253950114371,35.2840429958206,7.45617836410896));
#63574=CARTESIAN_POINT('Ctrl Pts',(-16.3434752900945,35.2888715272,7.3940150112991));
#63575=CARTESIAN_POINT('Ctrl Pts',(-16.360688737066,35.2934685619264,7.33483198666555));
#63576=CARTESIAN_POINT('Ctrl Pts',(-16.3811521205907,35.2980655966527,7.27646232160108));
#63577=CARTESIAN_POINT('Ctrl Pts',(-16.4047701441574,35.3026626313791,7.21928828436697));
#63578=CARTESIAN_POINT('Ctrl Pts',(-16.4287985847493,35.3073395500683,7.16112071783878));
#63579=CARTESIAN_POINT('Ctrl Pts',(-16.4560922934411,35.3120164687575,7.10419126539392));
#63580=CARTESIAN_POINT('Ctrl Pts',(-16.4864972678719,35.3166933874467,7.04888829948308));
#63581=CARTESIAN_POINT('Ctrl Pts',(-16.5163006442759,35.3212777678224,6.99467956751886));
#63582=CARTESIAN_POINT('Ctrl Pts',(-16.5490930309837,35.3258621481981,6.942034012477));
#63583=CARTESIAN_POINT('Ctrl Pts',(-16.5846811669062,35.3304465285739,6.89129667947134));
#63584=CARTESIAN_POINT('Ctrl Pts',(-16.6202475333548,35.3350281046569,6.84059038279334));
#63585=CARTESIAN_POINT('Ctrl Pts',(-16.6586059662633,35.33960968074,6.79179040955657));
#63586=CARTESIAN_POINT('Ctrl Pts',(-16.6995192765142,35.3441912568231,6.74521381926106));
#63587=CARTESIAN_POINT('Ctrl Pts',(-16.7404225907294,35.3487717135247,6.69864860866713));
#63588=CARTESIAN_POINT('Ctrl Pts',(-16.7838792073069,35.3533521702264,6.65430608495941));
#63589=CARTESIAN_POINT('Ctrl Pts',(-16.8296122643484,35.357932626928,6.61246952591105));
#63590=CARTESIAN_POINT('Ctrl Pts',(-16.8770181827825,35.362680631344,6.56910263477996));
#63591=CARTESIAN_POINT('Ctrl Pts',(-16.9268699213697,35.36742863576,6.52842903170431));
#63592=CARTESIAN_POINT('Ctrl Pts',(-16.9788200298526,35.372176640176,6.49071993308988));
#63593=CARTESIAN_POINT('Ctrl Pts',(-17.0290004127111,35.3767628996925,6.45429542771381));
#63594=CARTESIAN_POINT('Ctrl Pts',(-17.0811380077813,35.3813491592089,6.42063691214574));
#63595=CARTESIAN_POINT('Ctrl Pts',(-17.1348907892762,35.3859354187253,6.38994417079969));
#63596=CARTESIAN_POINT('Ctrl Pts',(-17.1914871423834,35.3907642955911,6.35762775518849));
#63597=CARTESIAN_POINT('Ctrl Pts',(-17.2498737426217,35.3955931724569,6.32859990749813));
#63598=CARTESIAN_POINT('Ctrl Pts',(-17.3096257081861,35.4004220493226,6.30303696773824));
#63599=CARTESIAN_POINT('Ctrl Pts',(-17.3693776737504,35.4052509261884,6.27747402797836));
#63600=CARTESIAN_POINT('Ctrl Pts',(-17.4304943668391,35.4100798030542,6.25537614417692));
#63601=CARTESIAN_POINT('Ctrl Pts',(-17.4925338173321,35.41490867992,6.23685837835318));
#63602=CARTESIAN_POINT('Ctrl Pts',(-17.5515960289201,35.4195058216566,6.21922926986613));
#63603=CARTESIAN_POINT('Ctrl Pts',(-17.6117371016633,35.4241029633933,6.20477204542772));
#63604=CARTESIAN_POINT('Ctrl Pts',(-17.6725841503931,35.4287001051299,6.19361390753489));
#63605=CARTESIAN_POINT('Ctrl Pts',(-17.7344869373383,35.4333770104428,6.18226216826233));
#63606=CARTESIAN_POINT('Ctrl Pts',(-17.7971199510101,35.4380539157558,6.17432533261754));
#63607=CARTESIAN_POINT('Ctrl Pts',(-17.8600733785421,35.4427308210687,6.16988458007531));
#63608=CARTESIAN_POINT('Ctrl Pts',(-17.9217828637429,35.447315312025,6.16553157557615));
#63609=CARTESIAN_POINT('Ctrl Pts',(-17.9837996829887,35.4518998029814,6.16453778560315));
#63610=CARTESIAN_POINT('Ctrl Pts',(-18.0457291105473,35.4564842939378,6.16692791707848));
#63611=CARTESIAN_POINT('Ctrl Pts',(-18.1076206702255,35.4610659816234,6.16931658706422));
#63612=CARTESIAN_POINT('Ctrl Pts',(-18.1694244365405,35.4656476693089,6.17508505606959));
#63613=CARTESIAN_POINT('Ctrl Pts',(-18.2307453797122,35.4702293569945,6.18420594669663));
#63614=CARTESIAN_POINT('Ctrl Pts',(-18.292051352411,35.4748099261384,6.19332461061223));
#63615=CARTESIAN_POINT('Ctrl Pts',(-18.3528742326574,35.4793904952823,6.20579399657293));
#63616=CARTESIAN_POINT('Ctrl Pts',(-18.4128258636383,35.4839710644262,6.2215350754821));
#63617=CARTESIAN_POINT('Ctrl Pts',(-18.474967527914,35.4887189617773,6.2378511760603));
#63618=CARTESIAN_POINT('Ctrl Pts',(-18.5361724781148,35.4934668591285,6.2576825394613));
#63619=CARTESIAN_POINT('Ctrl Pts',(-18.5960244732915,35.4982147564796,6.28088430757671));
#63620=CARTESIAN_POINT('Ctrl Pts',(-18.6538402893248,35.5028011292311,6.30329674601002));
#63621=CARTESIAN_POINT('Ctrl Pts',(-18.710393281511,35.5073875019826,6.32885365136161));
#63622=CARTESIAN_POINT('Ctrl Pts',(-18.7653301112277,35.511973874734,6.35737597136661));
#63623=CARTESIAN_POINT('Ctrl Pts',(-18.8231691198259,35.516802534385,6.38740505605384));
#63624=CARTESIAN_POINT('Ctrl Pts',(-18.8792159148823,35.521631194036,6.42072123326522));
#63625=CARTESIAN_POINT('Ctrl Pts',(-18.9330920032162,35.526459853687,6.45706317586196));
#63626=CARTESIAN_POINT('Ctrl Pts',(-18.9869680915501,35.531288513338,6.49340511845869));
#63627=CARTESIAN_POINT('Ctrl Pts',(-19.0386730031194,35.536117172989,6.53277237100758));
#63628=CARTESIAN_POINT('Ctrl Pts',(-19.0878704529053,35.54094583264,6.57485603302973));
#63629=CARTESIAN_POINT('Ctrl Pts',(-19.1341625502696,35.5454893360873,6.61445444693653));
#63630=CARTESIAN_POINT('Ctrl Pts',(-19.1784373949638,35.5500328395347,6.65663099304316));
#63631=CARTESIAN_POINT('Ctrl Pts',(-19.2203879253897,35.5545763429821,6.70114901285603));
#63632=CARTESIAN_POINT('Ctrl Pts',(-19.2621522608043,35.5590996803513,6.74546944200395));
#63633=CARTESIAN_POINT('Ctrl Pts',(-19.3016124668893,35.5636230177204,6.79211026620416));
#63634=CARTESIAN_POINT('Ctrl Pts',(-19.3384978864176,35.5681463550896,6.84079723659574));
#63635=CARTESIAN_POINT('Ctrl Pts',(-19.3753474306025,35.5726652929892,6.88943685326857));
#63636=CARTESIAN_POINT('Ctrl Pts',(-19.4096268323428,35.5771842308888,6.94011825861442));
#63637=CARTESIAN_POINT('Ctrl Pts',(-19.4411043180265,35.5817031687884,6.99253261744701));
#63638=CARTESIAN_POINT('Ctrl Pts',(-19.4725635320018,35.5862194835842,7.04491655136303));
#63639=CARTESIAN_POINT('Ctrl Pts',(-19.501223783586,35.5907357983799,7.09903099590914));
#63640=CARTESIAN_POINT('Ctrl Pts',(-19.5268967318177,35.5952521131756,7.15453837510904));
#63641=CARTESIAN_POINT('Ctrl Pts',(-19.5528264412119,35.5998135966923,7.21060089659642));
#63642=CARTESIAN_POINT('Ctrl Pts',(-19.5757084782704,35.6043750802091,7.26808390292818));
#63643=CARTESIAN_POINT('Ctrl Pts',(-19.5953974763933,35.6089365637258,7.32661631524103));
#63644=CARTESIAN_POINT('Ctrl Pts',(-19.6149016598431,35.6134552299759,7.38459930149502));
#63645=CARTESIAN_POINT('Ctrl Pts',(-19.6312723962809,35.6179738962259,7.44361154905003));
#63646=CARTESIAN_POINT('Ctrl Pts',(-19.6444185667383,35.6224925624759,7.50327712057099));
#63647=CARTESIAN_POINT('Ctrl Pts',(-19.6577515898165,35.627075454626,7.56379074654537));
#63648=CARTESIAN_POINT('Ctrl Pts',(-19.6677675384883,35.6316583467761,7.62497587102851));
#63649=CARTESIAN_POINT('Ctrl Pts',(-19.674425515394,35.6362412389263,7.68643255086586));
#63650=CARTESIAN_POINT('Ctrl Pts',(-19.6810834922998,35.6408241310764,7.74788923070321));
#63651=CARTESIAN_POINT('Ctrl Pts',(-19.6843835229444,35.6454070232265,7.80961690595762));
#63652=CARTESIAN_POINT('Ctrl Pts',(-19.6843395660614,35.6499899153767,7.87121620626327));
#63653=CARTESIAN_POINT('',(-19.6843394477967,36.443739915472,7.86862803641127));
#63654=CARTESIAN_POINT('Ctrl Pts',(-19.6843395660609,35.6499899154299,7.87121620697879));
#63655=CARTESIAN_POINT('Ctrl Pts',(-19.6842852362621,35.6556542720732,7.94735162419525));
#63656=CARTESIAN_POINT('Ctrl Pts',(-19.6791290596449,35.6613186287166,8.02330707152566));
#63657=CARTESIAN_POINT('Ctrl Pts',(-19.6689440442991,35.66698298536,8.09856695042523));
#63658=CARTESIAN_POINT('Ctrl Pts',(-19.6606780378931,35.6715800926505,8.15964674461064));
#63659=CARTESIAN_POINT('Ctrl Pts',(-19.6490774011019,35.676177199941,8.2204030153502));
#63660=CARTESIAN_POINT('Ctrl Pts',(-19.6341798253407,35.6807743072315,8.28044359056506));
#63661=CARTESIAN_POINT('Ctrl Pts',(-19.6190236388585,35.6854512168502,8.34152642505003));
#63662=CARTESIAN_POINT('Ctrl Pts',(-19.6004549338115,35.6901281264689,8.40186794066396));
#63663=CARTESIAN_POINT('Ctrl Pts',(-19.5785685526927,35.6948050360876,8.46106126411898));
#63664=CARTESIAN_POINT('Ctrl Pts',(-19.55711482541,35.6993894917333,8.51908444353228));
#63665=CARTESIAN_POINT('Ctrl Pts',(-19.5324735819567,35.7039739473791,8.57600391221258));
#63666=CARTESIAN_POINT('Ctrl Pts',(-19.5047849065872,35.7085584030249,8.63144981728524));
#63667=CARTESIAN_POINT('Ctrl Pts',(-19.477113163443,35.7131400551766,8.686861815985));
#63668=CARTESIAN_POINT('Ctrl Pts',(-19.4463979105317,35.7177217073284,8.74080158335486));
#63669=CARTESIAN_POINT('Ctrl Pts',(-19.4128268173985,35.7223033594801,8.79292044453666));
#63670=CARTESIAN_POINT('Ctrl Pts',(-19.3792639213525,35.7268838929253,8.84502657980423));
#63671=CARTESIAN_POINT('Ctrl Pts',(-19.3428468448988,35.7314644263705,8.89531226371593));
#63672=CARTESIAN_POINT('Ctrl Pts',(-19.3038074921772,35.7360449598156,8.94345636113232));
#63673=CARTESIAN_POINT('Ctrl Pts',(-19.2633414251559,35.7407928913377,8.99335991067695));
#63674=CARTESIAN_POINT('Ctrl Pts',(-19.2200580231003,35.7455408228597,9.04096181964529));
#63675=CARTESIAN_POINT('Ctrl Pts',(-19.1742607568843,35.7502887543817,9.08594246581251));
#63676=CARTESIAN_POINT('Ctrl Pts',(-19.1300221872733,35.7548750914384,9.12939220879997));
#63677=CARTESIAN_POINT('Ctrl Pts',(-19.0834385756392,35.7594614284952,9.170395965748));
#63678=CARTESIAN_POINT('Ctrl Pts',(-19.0348186262504,35.764047765552,9.20870553196557));
#63679=CARTESIAN_POINT('Ctrl Pts',(-18.9836290724174,35.7688764943066,9.24903979036904));
#63680=CARTESIAN_POINT('Ctrl Pts',(-18.9301824890949,35.7737052230613,9.28638679929457));
#63681=CARTESIAN_POINT('Ctrl Pts',(-18.8748729381879,35.7785339518159,9.3205093105868));
#63682=CARTESIAN_POINT('Ctrl Pts',(-18.8195633872809,35.7833626805706,9.35463182187903));
#63683=CARTESIAN_POINT('Ctrl Pts',(-18.7623914774936,35.7881914093252,9.38552959481498));
#63684=CARTESIAN_POINT('Ctrl Pts',(-18.7037772347804,35.7930201380799,9.41302344441478));
#63685=CARTESIAN_POINT('Ctrl Pts',(-18.6479743930322,35.797617259429,9.43919856614713));
#63686=CARTESIAN_POINT('Ctrl Pts',(-18.5906351878047,35.8022143807782,9.46239641294078));
#63687=CARTESIAN_POINT('Ctrl Pts',(-18.5321095708365,35.8068115021273,9.48243600102166));
#63688=CARTESIAN_POINT('Ctrl Pts',(-18.4725681975944,35.8114884099887,9.50282339128514));
#63689=CARTESIAN_POINT('Ctrl Pts',(-18.4117992776774,35.81616531785,9.51994153812279));
#63690=CARTESIAN_POINT('Ctrl Pts',(-18.3501961007209,35.8208422257114,9.53364950714117));
#63691=CARTESIAN_POINT('Ctrl Pts',(-18.2898104917995,35.8254266959129,9.5470865423258));
#63692=CARTESIAN_POINT('Ctrl Pts',(-18.228623824416,35.8300111661145,9.55724685912381));
#63693=CARTESIAN_POINT('Ctrl Pts',(-18.1670228187882,35.834595636316,9.56404760879159));
#63694=CARTESIAN_POINT('Ctrl Pts',(-18.1054594814475,35.8391773031682,9.57084419988131));
#63695=CARTESIAN_POINT('Ctrl Pts',(-18.0434828131926,35.8437589700204,9.5742852415339));
#63696=CARTESIAN_POINT('Ctrl Pts',(-17.9814875427819,35.8483406368726,9.57433935083846));
#63697=CARTESIAN_POINT('Ctrl Pts',(-17.9195074081365,35.8529211851389,9.57439344693257));
#63698=CARTESIAN_POINT('Ctrl Pts',(-17.8575091891972,35.8575017334052,9.57106225174645));
#63699=CARTESIAN_POINT('Ctrl Pts',(-17.7958884611795,35.8620822816714,9.56436648245684));
#63700=CARTESIAN_POINT('Ctrl Pts',(-17.732016166547,35.8668301990988,9.55742605571059));
#63701=CARTESIAN_POINT('Ctrl Pts',(-17.6685500690245,35.8715781165262,9.54687041744939));
#63702=CARTESIAN_POINT('Ctrl Pts',(-17.605923271481,35.8763260339536,9.53278123539465));
#63703=CARTESIAN_POINT('Ctrl Pts',(-17.5454275819437,35.8809123859611,9.51917148977694));
#63704=CARTESIAN_POINT('Ctrl Pts',(-17.4857154745479,35.8854987379686,9.50226504846101));
#63705=CARTESIAN_POINT('Ctrl Pts',(-17.4271628914053,35.890085089976,9.48218670350573));
#63706=CARTESIAN_POINT('Ctrl Pts',(-17.3655163222364,35.8949137901134,9.46104739564517));
#63707=CARTESIAN_POINT('Ctrl Pts',(-17.3051558190442,35.8997424902507,9.4363919073577));
#63708=CARTESIAN_POINT('Ctrl Pts',(-17.2464943920001,35.904571190388,9.40842268529577));
#63709=CARTESIAN_POINT('Ctrl Pts',(-17.1878329649559,35.9093998905254,9.38045346323384));
#63710=CARTESIAN_POINT('Ctrl Pts',(-17.1308711463604,35.9142285906627,9.34917088828989));
#63711=CARTESIAN_POINT('Ctrl Pts',(-17.0759872408914,35.9190572908,9.31483070529693));
#63712=CARTESIAN_POINT('Ctrl Pts',(-17.0237355377478,35.9236544090989,9.2821374588468));
#63713=CARTESIAN_POINT('Ctrl Pts',(-16.9731523080326,35.9282515273978,9.24653891649767));
#63714=CARTESIAN_POINT('Ctrl Pts',(-16.924579377696,35.9328486456967,9.20823097618292));
#63715=CARTESIAN_POINT('Ctrl Pts',(-16.8751633906599,35.9375255539393,9.16925814360195));
#63716=CARTESIAN_POINT('Ctrl Pts',(-16.8278286522298,35.9422024621819,9.12748116553173));
#63717=CARTESIAN_POINT('Ctrl Pts',(-16.7829068386722,35.9468793704246,9.0831540704718));
#63718=CARTESIAN_POINT('Ctrl Pts',(-16.7388729242615,35.9514638375454,9.03970311968939));
#63719=CARTESIAN_POINT('Ctrl Pts',(-16.697157797824,35.9560483046663,8.99380231765614));
#63720=CARTESIAN_POINT('Ctrl Pts',(-16.6580407679681,35.9606327717871,8.94573166935142));
#63721=CARTESIAN_POINT('Ctrl Pts',(-16.6189476577524,35.965214435556,8.89769041572762));
#63722=CARTESIAN_POINT('Ctrl Pts',(-16.5824498145957,35.9697960993248,8.84748234079259));
#63723=CARTESIAN_POINT('Ctrl Pts',(-16.5487876471297,35.9743777630936,8.79542208564061));
#63724=CARTESIAN_POINT('Ctrl Pts',(-16.515133698063,35.9789583082791,8.74337454066144));
#63725=CARTESIAN_POINT('Ctrl Pts',(-16.4843143266433,35.9835388534645,8.68947614044453));
#63726=CARTESIAN_POINT('Ctrl Pts',(-16.4565266249892,35.9881193986499,8.63407048839299));
#63727=CARTESIAN_POINT('Ctrl Pts',(-16.427723547981,35.9928673190557,8.57664028842207));
#63728=CARTESIAN_POINT('Ctrl Pts',(-16.4021783051839,35.9976152394616,8.5175910447526));
#63729=CARTESIAN_POINT('Ctrl Pts',(-16.3800571267117,36.0023631598674,8.45733094402891));
#63730=CARTESIAN_POINT('Ctrl Pts',(-16.3586887305708,36.0069495088363,8.39912149079511));
#63731=CARTESIAN_POINT('Ctrl Pts',(-16.3405151730133,36.0115358578053,8.33978279836506));
#63732=CARTESIAN_POINT('Ctrl Pts',(-16.3256354543646,36.0161222067742,8.27969840827669));
#63733=CARTESIAN_POINT('Ctrl Pts',(-16.3099694444177,36.0209509128985,8.21643896937226));
#63734=CARTESIAN_POINT('Ctrl Pts',(-16.2979551716987,36.0257796190228,8.15235346972648));
#63735=CARTESIAN_POINT('Ctrl Pts',(-16.2896464898562,36.0306083251471,8.08789870661546));
#63736=CARTESIAN_POINT('Ctrl Pts',(-16.2813378080138,36.0354370312714,8.02344394350444));
#63737=CARTESIAN_POINT('Ctrl Pts',(-16.2767346856514,36.0402657373957,7.95862057072215));
#63738=CARTESIAN_POINT('Ctrl Pts',(-16.2758273748365,36.04509444352,7.89388512598626));
#63739=CARTESIAN_POINT('Ctrl Pts',(-16.2749635795829,36.0496915599244,7.83225445986492));
#63740=CARTESIAN_POINT('Ctrl Pts',(-16.27744559109,36.0542886763289,7.77045029018436));
#63741=CARTESIAN_POINT('Ctrl Pts',(-16.2832941663669,36.0588857927333,7.70886605039501));
#63742=CARTESIAN_POINT('Ctrl Pts',(-16.2892442552701,36.0635627012128,7.64621289395288));
#63743=CARTESIAN_POINT('Ctrl Pts',(-16.298678991754,36.0682396096922,7.58378790397998));
#63744=CARTESIAN_POINT('Ctrl Pts',(-16.3115647867247,36.0729165181717,7.52200750769174));
#63745=CARTESIAN_POINT('Ctrl Pts',(-16.3241958822037,36.0775009832888,7.46144825729071));
#63746=CARTESIAN_POINT('Ctrl Pts',(-16.3401427422826,36.082085448406,7.40150887309082));
#63747=CARTESIAN_POINT('Ctrl Pts',(-16.3593215557563,36.0866699135232,7.34257586710154));
#63748=CARTESIAN_POINT('Ctrl Pts',(-16.3784886414409,36.0912515752532,7.2836788984752));
#63749=CARTESIAN_POINT('Ctrl Pts',(-16.4008836045432,36.0958332369832,7.22578757090005));
#63750=CARTESIAN_POINT('Ctrl Pts',(-16.4263724385346,36.1004148987132,7.16927449321788));
#63751=CARTESIAN_POINT('Ctrl Pts',(-16.4518550494127,36.1049954418279,7.11277521323577));
#63752=CARTESIAN_POINT('Ctrl Pts',(-16.4804298224537,36.1095759849426,7.05765397899624));
#63753=CARTESIAN_POINT('Ctrl Pts',(-16.5119149281939,36.1141565280573,7.00426270870425));
#63754=CARTESIAN_POINT('Ctrl Pts',(-16.5445505422352,36.1189044504059,6.94892044926253));
#63755=CARTESIAN_POINT('Ctrl Pts',(-16.5803130608027,36.1236523727544,6.89543756585259));
#63756=CARTESIAN_POINT('Ctrl Pts',(-16.6189496548617,36.128400295103,6.84417506678822));
#63757=CARTESIAN_POINT('Ctrl Pts',(-16.6562714154448,36.1329866419453,6.79465707060959));
#63758=CARTESIAN_POINT('Ctrl Pts',(-16.6962743728658,36.1375729887876,6.74721111209977));
#63759=CARTESIAN_POINT('Ctrl Pts',(-16.7386899508729,36.1421593356299,6.70212834714767));
#63760=CARTESIAN_POINT('Ctrl Pts',(-16.7833469593884,36.1469880457316,6.65466320549543));
#63761=CARTESIAN_POINT('Ctrl Pts',(-16.8306781869341,36.1518167558333,6.60981840046909));
#63762=CARTESIAN_POINT('Ctrl Pts',(-16.880329024369,36.156645465935,6.56788687858741));
#63763=CARTESIAN_POINT('Ctrl Pts',(-16.9299798618039,36.1614741760366,6.52595535670574));
#63764=CARTESIAN_POINT('Ctrl Pts',(-16.9819497427688,36.1663028861383,6.48693744610878));
#63765=CARTESIAN_POINT('Ctrl Pts',(-17.0358497883043,36.17113159624,6.45107251300325));
#63766=CARTESIAN_POINT('Ctrl Pts',(-17.0871647100218,36.1757287144503,6.41692771374697));
#63767=CARTESIAN_POINT('Ctrl Pts',(-17.1404396653232,36.1803258326605,6.38550004795636));
#63768=CARTESIAN_POINT('Ctrl Pts',(-17.1953553387445,36.1849229508708,6.35702029386931));
#63769=CARTESIAN_POINT('Ctrl Pts',(-17.2512241579779,36.1895998591245,6.32804622993145));
#63770=CARTESIAN_POINT('Ctrl Pts',(-17.3087908038339,36.1942767673782,6.30212375768071));
#63771=CARTESIAN_POINT('Ctrl Pts',(-17.3676871725774,36.1989536756319,6.27945046069801));
#63772=CARTESIAN_POINT('Ctrl Pts',(-17.4254194272433,36.2035381426222,6.25722531195888));
#63773=CARTESIAN_POINT('Ctrl Pts',(-17.4844288198954,36.2081226096125,6.23812225639109));
#63774=CARTESIAN_POINT('Ctrl Pts',(-17.5443451489424,36.2127070766028,6.22228045883105));
#63775=CARTESIAN_POINT('Ctrl Pts',(-17.6042248396019,36.2172887402257,6.20644834841187));
#63776=CARTESIAN_POINT('Ctrl Pts',(-17.665009875857,36.2218704038487,6.19387367158885));
#63777=CARTESIAN_POINT('Ctrl Pts',(-17.7263145196248,36.2264520674717,6.18464587915572));
#63778=CARTESIAN_POINT('Ctrl Pts',(-17.7876041960597,36.2310326124961,6.17542033965863));
#63779=CARTESIAN_POINT('Ctrl Pts',(-17.8494127249925,36.2356131575205,6.16954013817003));
#63780=CARTESIAN_POINT('Ctrl Pts',(-17.9113458212266,36.240193702545,6.16704332429244));
#63781=CARTESIAN_POINT('Ctrl Pts',(-17.9755419851792,36.2449416230795,6.16445527553028));
#63782=CARTESIAN_POINT('Ctrl Pts',(-18.0398714169071,36.2496895436141,6.16550274986414));
#63783=CARTESIAN_POINT('Ctrl Pts',(-18.1038936953115,36.2544374641487,6.17016907080085));
#63784=CARTESIAN_POINT('Ctrl Pts',(-18.1657372952182,36.2590238129205,6.17467659680957));
#63785=CARTESIAN_POINT('Ctrl Pts',(-18.2272937973692,36.2636101616924,6.18256047419938));
#63786=CARTESIAN_POINT('Ctrl Pts',(-18.2881729321403,36.2681965104642,6.19375291812453));
#63787=CARTESIAN_POINT('Ctrl Pts',(-18.3522691191712,36.2730252168802,6.2055368073315));
#63788=CARTESIAN_POINT('Ctrl Pts',(-18.4156137347041,36.2778539232961,6.22098848966207));
#63789=CARTESIAN_POINT('Ctrl Pts',(-18.4777683550696,36.2826826297121,6.23996886523866));
#63790=CARTESIAN_POINT('Ctrl Pts',(-18.5399229754351,36.287511336128,6.25894924081525));
#63791=CARTESIAN_POINT('Ctrl Pts',(-18.6008870178212,36.292340042544,6.28145801170677));
#63792=CARTESIAN_POINT('Ctrl Pts',(-18.6602484949544,36.29716874896,6.30729823039958));
#63793=CARTESIAN_POINT('Ctrl Pts',(-18.7167629470633,36.3017658666645,6.33189913105645));
#63794=CARTESIAN_POINT('Ctrl Pts',(-18.7720572323024,36.3063629843689,6.3596202454074));
#63795=CARTESIAN_POINT('Ctrl Pts',(-18.8257642986772,36.3109601020734,6.39031841713051));
#63796=CARTESIAN_POINT('Ctrl Pts',(-18.8804035403833,36.3156370103903,6.42154940660611));
#63797=CARTESIAN_POINT('Ctrl Pts',(-18.9333994157732,36.3203139187073,6.45586165797432));
#63798=CARTESIAN_POINT('Ctrl Pts',(-18.9843863082443,36.3249908270242,6.49305302229481));
#63799=CARTESIAN_POINT('Ctrl Pts',(-19.0343654148208,36.3295752934997,6.52950927744225));
#63800=CARTESIAN_POINT('Ctrl Pts',(-19.0824138018446,36.3341597599751,6.56873155216557));
#63801=CARTESIAN_POINT('Ctrl Pts',(-19.1282137998569,36.3387442264506,6.61048425757431));
#63802=CARTESIAN_POINT('Ctrl Pts',(-19.1739857914902,36.3433258895568,6.65221143149514));
#63803=CARTESIAN_POINT('Ctrl Pts',(-19.2175117448531,36.347907552663,6.69646562570516));
#63804=CARTESIAN_POINT('Ctrl Pts',(-19.2585073365847,36.3524892157692,6.74297123998581));
#63805=CARTESIAN_POINT('Ctrl Pts',(-19.2994929193627,36.3570697602757,6.78946550005701));
#63806=CARTESIAN_POINT('Ctrl Pts',(-19.3379490304058,36.3616503047823,6.8382097072997));
#63807=CARTESIAN_POINT('Ctrl Pts',(-19.3736298999924,36.3662308492889,6.88889320792929));
#63808=CARTESIAN_POINT('Ctrl Pts',(-19.4106145752701,36.3709787703215,6.94142872162177));
#63809=CARTESIAN_POINT('Ctrl Pts',(-19.444616876485,36.3757266913541,6.99604755945913));
#63810=CARTESIAN_POINT('Ctrl Pts',(-19.4754119986822,36.3804746123866,7.05237062809768));
#63811=CARTESIAN_POINT('Ctrl Pts',(-19.5051591562389,36.385060960644,7.10677701058069));
#63812=CARTESIAN_POINT('Ctrl Pts',(-19.5319137604025,36.3896473089013,7.16277298205991));
#63813=CARTESIAN_POINT('Ctrl Pts',(-19.555521143059,36.3942336571586,7.21999387435651));
#63814=CARTESIAN_POINT('Ctrl Pts',(-19.5803760248537,36.3990623645789,7.2802385247234));
#63815=CARTESIAN_POINT('Ctrl Pts',(-19.6017416168723,36.4038910719991,7.34184053833335));
#63816=CARTESIAN_POINT('Ctrl Pts',(-19.619497059826,36.4087197794193,7.40435611630556));
#63817=CARTESIAN_POINT('Ctrl Pts',(-19.6372525027796,36.4135484868395,7.46687169427777));
#63818=CARTESIAN_POINT('Ctrl Pts',(-19.651397730968,36.4183771942597,7.53030018536893));
#63819=CARTESIAN_POINT('Ctrl Pts',(-19.661874824937,36.4232059016799,7.59418863539891));
#63820=CARTESIAN_POINT('Ctrl Pts',(-19.676726058949,36.4300505729299,7.68475022861004));
#63821=CARTESIAN_POINT('Ctrl Pts',(-19.6842653206136,36.4368952441799,7.77654262605148));
#63822=CARTESIAN_POINT('Ctrl Pts',(-19.6843394477962,36.4437399154299,7.86862803584488));
#63823=CARTESIAN_POINT('',(-19.6843399609503,37.2374899153791,7.86963516025695));
#63824=CARTESIAN_POINT('Ctrl Pts',(-19.6843394477967,36.443739915472,7.86862803641127));
#63825=CARTESIAN_POINT('Ctrl Pts',(-19.6843884176661,36.4482616412974,7.92946148777897));
#63826=CARTESIAN_POINT('Ctrl Pts',(-19.6811761431254,36.4527833671228,7.99041301810678));
#63827=CARTESIAN_POINT('Ctrl Pts',(-19.6746912185231,36.4573050929483,8.05109806586693));
#63828=CARTESIAN_POINT('Ctrl Pts',(-19.6682129609578,36.4618221700668,8.11172072439519));
#63829=CARTESIAN_POINT('Ctrl Pts',(-19.6584687697771,36.4663392471853,8.17207692326294));
#63830=CARTESIAN_POINT('Ctrl Pts',(-19.6454992584212,36.4708563243038,8.23178316129772));
#63831=CARTESIAN_POINT('Ctrl Pts',(-19.6325379840047,36.4753705326256,8.29145147988756));
#63832=CARTESIAN_POINT('Ctrl Pts',(-19.6163555582859,36.4798847409475,8.35047014286125));
#63833=CARTESIAN_POINT('Ctrl Pts',(-19.5970439853245,36.4843989492693,8.40846409827013));
#63834=CARTESIAN_POINT('Ctrl Pts',(-19.5777370902191,36.4889120641113,8.46644400576209));
#63835=CARTESIAN_POINT('Ctrl Pts',(-19.5553027178393,36.4934251789532,8.52339919969336));
#63836=CARTESIAN_POINT('Ctrl Pts',(-19.5298825606297,36.4979382937952,8.578970298289));
#63837=CARTESIAN_POINT('Ctrl Pts',(-19.5044407789576,36.5024552478613,8.63458867020125));
#63838=CARTESIAN_POINT('Ctrl Pts',(-19.4760083566962,36.5069722019275,8.68882011513211));
#63839=CARTESIAN_POINT('Ctrl Pts',(-19.4447743476152,36.5114891559936,8.74132711777411));
#63840=CARTESIAN_POINT('Ctrl Pts',(-19.4135273527354,36.516007988021,8.79385595063864));
#63841=CARTESIAN_POINT('Ctrl Pts',(-19.3794767452545,36.5205268200483,8.84465847661094));
#63842=CARTESIAN_POINT('Ctrl Pts',(-19.342854838816,36.5250456520757,8.89342636467692));
#63843=CARTESIAN_POINT('Ctrl Pts',(-19.3061658589121,36.5295727603986,8.94228357172081));
#63844=CARTESIAN_POINT('Ctrl Pts',(-19.2668965152215,36.5340998687216,8.9890982968607));
#63845=CARTESIAN_POINT('Ctrl Pts',(-19.2253185702707,36.5386269770445,9.033596362206));
#63846=CARTESIAN_POINT('Ctrl Pts',(-19.1928184511077,36.5421656694963,9.06837904393669));
#63847=CARTESIAN_POINT('Ctrl Pts',(-19.1589085972443,36.5457043619481,9.10174690959737));
#63848=CARTESIAN_POINT('Ctrl Pts',(-19.1237326718399,36.5492430543999,9.13358632905155));
#63849=CARTESIAN_POINT('Ctrl Pts',(-19.0780356034287,36.5538401721501,9.17494894033305));
#63850=CARTESIAN_POINT('Ctrl Pts',(-19.02999799142,36.5584372899004,9.21391438730474));
#63851=CARTESIAN_POINT('Ctrl Pts',(-18.9799014841208,36.5630344076506,9.25020717924991));
#63852=CARTESIAN_POINT('Ctrl Pts',(-18.9289354693085,36.5677113159618,9.28712989246045));
#63853=CARTESIAN_POINT('Ctrl Pts',(-18.8758387360898,36.572388224273,9.32128586270452));
#63854=CARTESIAN_POINT('Ctrl Pts',(-18.8209460962525,36.5770651325842,9.35242520850049));
#63855=CARTESIAN_POINT('Ctrl Pts',(-18.7671384411369,36.5816495991022,9.38294906714675));
#63856=CARTESIAN_POINT('Ctrl Pts',(-18.711605691783,36.5862340656202,9.41057420322532));
#63857=CARTESIAN_POINT('Ctrl Pts',(-18.6546933796397,36.5908185321382,9.43510820043547));
#63858=CARTESIAN_POINT('Ctrl Pts',(-18.597815868994,36.5954001952856,9.4596271952707));
#63859=CARTESIAN_POINT('Ctrl Pts',(-18.5395609347949,36.599981858433,9.48105859813366));
#63860=CARTESIAN_POINT('Ctrl Pts',(-18.4802968307819,36.6045635215804,9.49925686026162));
#63861=CARTESIAN_POINT('Ctrl Pts',(-18.4210471959441,36.6091440661268,9.51745067933173));
#63862=CARTESIAN_POINT('Ctrl Pts',(-18.3607893668345,36.6137246106732,9.53241277529591));
#63863=CARTESIAN_POINT('Ctrl Pts',(-18.2999076567283,36.6183051552197,9.54404716981531));
#63864=CARTESIAN_POINT('Ctrl Pts',(-18.236801284441,36.6230530762113,9.55610669361312));
#63865=CARTESIAN_POINT('Ctrl Pts',(-18.1730251143417,36.627800997203,9.56459044266918));
#63866=CARTESIAN_POINT('Ctrl Pts',(-18.1090171864571,36.6325489181947,9.56944973482557));
#63867=CARTESIAN_POINT('Ctrl Pts',(-18.0471874611272,36.6371352664879,9.57414366430051));
#63868=CARTESIAN_POINT('Ctrl Pts',(-17.985142028619,36.6417216147811,9.57545593148886));
#63869=CARTESIAN_POINT('Ctrl Pts',(-17.9232768925918,36.6463079630743,9.57339582149481));
#63870=CARTESIAN_POINT('Ctrl Pts',(-17.8581425815048,36.6511366704153,9.5712268479203));
#63871=CARTESIAN_POINT('Ctrl Pts',(-17.79320879456,36.6559653777562,9.56531924259274));
#63872=CARTESIAN_POINT('Ctrl Pts',(-17.7289297131063,36.6607940850972,9.55574569453376));
#63873=CARTESIAN_POINT('Ctrl Pts',(-17.6646506316526,36.6656227924381,9.54617214647477));
#63874=CARTESIAN_POINT('Ctrl Pts',(-17.601026876175,36.6704514997791,9.53293286408911));
#63875=CARTESIAN_POINT('Ctrl Pts',(-17.5384950431571,36.67528020712,9.51616165934064));
#63876=CARTESIAN_POINT('Ctrl Pts',(-17.4789622998473,36.6798773247923,9.50019481846777));
#63877=CARTESIAN_POINT('Ctrl Pts',(-17.4201745493426,36.6844744424645,9.48096155356177));
#63878=CARTESIAN_POINT('Ctrl Pts',(-17.3625159870928,36.6890715601368,9.45854912716101));
#63879=CARTESIAN_POINT('Ctrl Pts',(-17.3038566642767,36.6937484684578,9.43574769569905));
#63880=CARTESIAN_POINT('Ctrl Pts',(-17.2463666384539,36.6984253767787,9.40965573658915));
#63881=CARTESIAN_POINT('Ctrl Pts',(-17.1904374154254,36.7031022850997,9.38041906788806));
#63882=CARTESIAN_POINT('Ctrl Pts',(-17.1356136668515,36.7076867515379,9.35176027938338));
#63883=CARTESIAN_POINT('Ctrl Pts',(-17.0822900553124,36.7122712179762,9.32008021122148));
#63884=CARTESIAN_POINT('Ctrl Pts',(-17.0308156159192,36.7168556844144,9.28556484860887));
#63885=CARTESIAN_POINT('Ctrl Pts',(-16.9793726528064,36.7214373474817,9.25107059191304));
#63886=CARTESIAN_POINT('Ctrl Pts',(-16.9297770416608,36.7260190105489,9.21374476148654));
#63887=CARTESIAN_POINT('Ctrl Pts',(-16.8823507596549,36.7306006736161,9.17381784800244));
#63888=CARTESIAN_POINT('Ctrl Pts',(-16.8349360566544,36.735181218082,9.13390068257217));
#63889=CARTESIAN_POINT('Ctrl Pts',(-16.7896900206579,36.7397617625479,9.09138402245842));
#63890=CARTESIAN_POINT('Ctrl Pts',(-16.7469016870263,36.7443423070139,9.04653873125422));
#63891=CARTESIAN_POINT('Ctrl Pts',(-16.702549834913,36.7490902280827,9.00005475876336));
#63892=CARTESIAN_POINT('Ctrl Pts',(-16.6608392231333,36.7538381491515,8.95106905795808));
#63893=CARTESIAN_POINT('Ctrl Pts',(-16.6220482810392,36.7585860702204,8.89992328091535));
#63894=CARTESIAN_POINT('Ctrl Pts',(-16.584577403708,36.7631724184332,8.85051800653634));
#63895=CARTESIAN_POINT('Ctrl Pts',(-16.5498308984838,36.7677587666461,8.79909779660216));
#63896=CARTESIAN_POINT('Ctrl Pts',(-16.5180156953963,36.772345114859,8.74600041592022));
#63897=CARTESIAN_POINT('Ctrl Pts',(-16.4845192615167,36.7771738223558,8.69009717694659));
#63898=CARTESIAN_POINT('Ctrl Pts',(-16.4542728327011,36.7820025298526,8.63233516249499));
#63899=CARTESIAN_POINT('Ctrl Pts',(-16.4274616124387,36.7868312373494,8.57313540001092));
#63900=CARTESIAN_POINT('Ctrl Pts',(-16.4006503921763,36.7916599448463,8.51393563752685));
#63901=CARTESIAN_POINT('Ctrl Pts',(-16.377274541817,36.7964886523431,8.45329876136088));
#63902=CARTESIAN_POINT('Ctrl Pts',(-16.3574583728186,36.8013173598399,8.39166416750968));
#63903=CARTESIAN_POINT('Ctrl Pts',(-16.338592607919,36.8059144774973,8.33298563295686));
#63904=CARTESIAN_POINT('Ctrl Pts',(-16.3228753258776,36.8105115951546,8.27316184919246));
#63905=CARTESIAN_POINT('Ctrl Pts',(-16.3104415356123,36.815108712812,8.21256294252501));
#63906=CARTESIAN_POINT('Ctrl Pts',(-16.2977919361219,36.8197856211348,8.15091224048277));
#63907=CARTESIAN_POINT('Ctrl Pts',(-16.2885411492661,36.8244625294577,8.08845972777955));
#63908=CARTESIAN_POINT('Ctrl Pts',(-16.2827789484866,36.8291394377805,8.02561342454811));
#63909=CARTESIAN_POINT('Ctrl Pts',(-16.2771306410648,36.8337239042026,7.96400931622946));
#63910=CARTESIAN_POINT('Ctrl Pts',(-16.2748343156635,36.8383083706247,7.90202737426948));
#63911=CARTESIAN_POINT('Ctrl Pts',(-16.2759229669212,36.8428928370467,7.84006171458732));
#63912=CARTESIAN_POINT('Ctrl Pts',(-16.2770109524758,36.8474745000974,7.77813394650358));
#63913=CARTESIAN_POINT('Ctrl Pts',(-16.2814798014819,36.852056163148,7.71622294889516));
#63914=CARTESIAN_POINT('Ctrl Pts',(-16.2893104421463,36.8566378261987,7.65472423600295));
#63915=CARTESIAN_POINT('Ctrl Pts',(-16.2971391709792,36.8612183706476,7.59324053786974));
#63916=CARTESIAN_POINT('Ctrl Pts',(-16.3083279978462,36.8657989150965,7.53216942940354));
#63917=CARTESIAN_POINT('Ctrl Pts',(-16.3228060662602,36.8703794595454,7.47190063856369));
#63918=CARTESIAN_POINT('Ctrl Pts',(-16.3378131744878,36.8751273806299,7.40942957950931));
#63919=CARTESIAN_POINT('Ctrl Pts',(-16.3563544867805,36.8798753017145,7.3478211889271));
#63920=CARTESIAN_POINT('Ctrl Pts',(-16.3782939177123,36.884623222799,7.28749466821109));
#63921=CARTESIAN_POINT('Ctrl Pts',(-16.3994867445648,36.8892095709941,7.22922107341622));
#63922=CARTESIAN_POINT('Ctrl Pts',(-16.4238498405645,36.8937959191891,7.17214395764723));
#63923=CARTESIAN_POINT('Ctrl Pts',(-16.4512116161967,36.8983822673842,7.11662033930563));
#63924=CARTESIAN_POINT('Ctrl Pts',(-16.480019287658,36.9032109749135,7.05816265084882));
#63925=CARTESIAN_POINT('Ctrl Pts',(-16.5121510421769,36.9080396824428,7.0014277657604));
#63926=CARTESIAN_POINT('Ctrl Pts',(-16.5473535501985,36.9128683899721,6.94679959625704));
#63927=CARTESIAN_POINT('Ctrl Pts',(-16.5825560582201,36.9176970975014,6.89217142675367));
#63928=CARTESIAN_POINT('Ctrl Pts',(-16.6208288742422,36.9225258050307,6.83965045237918));
#63929=CARTESIAN_POINT('Ctrl Pts',(-16.6618702166072,36.92735451256,6.78957938295643));
#63930=CARTESIAN_POINT('Ctrl Pts',(-16.7009431734319,36.9319516302452,6.74190977419162));
#63931=CARTESIAN_POINT('Ctrl Pts',(-16.7426856445409,36.9365487479304,6.69626457493456));
#63932=CARTESIAN_POINT('Ctrl Pts',(-16.7868598506812,36.9411458656157,6.65295792197494));
#63933=CARTESIAN_POINT('Ctrl Pts',(-16.8318007737431,36.945822773935,6.60889960992414));
#63934=CARTESIAN_POINT('Ctrl Pts',(-16.879258387699,36.9504996822544,6.56726226763398));
#63935=CARTESIAN_POINT('Ctrl Pts',(-16.9289385453971,36.9551765905737,6.52834257194767));
#63936=CARTESIAN_POINT('Ctrl Pts',(-16.9776367452975,36.9597610570248,6.49019214714203));
#63937=CARTESIAN_POINT('Ctrl Pts',(-17.0284700086245,36.9643455234759,6.45465324414821));
#63938=CARTESIAN_POINT('Ctrl Pts',(-17.0811250827108,36.9689299899269,6.4219672936469));
#63939=CARTESIAN_POINT('Ctrl Pts',(-17.1337479585654,36.9735116530069,6.3893013303894));
#63940=CARTESIAN_POINT('Ctrl Pts',(-17.1881900046145,36.9780933160869,6.35948512835093));
#63941=CARTESIAN_POINT('Ctrl Pts',(-17.2441085604581,36.9826749791669,6.33271712921499));
#63942=CARTESIAN_POINT('Ctrl Pts',(-17.300013463928,36.9872555236454,6.30595566541822));
#63943=CARTESIAN_POINT('Ctrl Pts',(-17.3573937026054,36.991836068124,6.28224114686672));
#63944=CARTESIAN_POINT('Ctrl Pts',(-17.4158833977731,36.9964166126025,6.2617253671428));
#63945=CARTESIAN_POINT('Ctrl Pts',(-17.4765103508726,37.001164533659,6.24045992522937));
#63946=CARTESIAN_POINT('Ctrl Pts',(-17.5383288825202,37.0059124547154,6.22263176937869));
#63947=CARTESIAN_POINT('Ctrl Pts',(-17.6009129797018,37.0106603757719,6.20835386840596));
#63948=CARTESIAN_POINT('Ctrl Pts',(-17.6613673258495,37.015246723997,6.19456184764446));
#63949=CARTESIAN_POINT('Ctrl Pts',(-17.722535434032,37.0198330722221,6.18408233538082));
#63950=CARTESIAN_POINT('Ctrl Pts',(-17.7840242866189,37.0244194204472,6.17696475070223));
#63951=CARTESIAN_POINT('Ctrl Pts',(-17.8487624328227,37.0292481279193,6.16947104707702));
#63952=CARTESIAN_POINT('Ctrl Pts',(-17.9138555181008,37.0340768353914,6.16570448675005));
#63953=CARTESIAN_POINT('Ctrl Pts',(-17.978843604896,37.0389055428635,6.16566039230722));
#63954=CARTESIAN_POINT('Ctrl Pts',(-18.0438316916913,37.0437342503356,6.1656162978644));
#63955=CARTESIAN_POINT('Ctrl Pts',(-18.1087141355099,37.0485629578078,6.16929455501697));
#63956=CARTESIAN_POINT('Ctrl Pts',(-18.1730393448705,37.0533916652799,6.17662743410319));
#63957=CARTESIAN_POINT('Ctrl Pts',(-18.2342794507435,37.0579887829537,6.1836086207337));
#63958=CARTESIAN_POINT('Ctrl Pts',(-18.295266142784,37.0625859006275,6.19393051412742));
#63959=CARTESIAN_POINT('Ctrl Pts',(-18.3556065421868,37.0671830183013,6.20756366706376));
#63960=CARTESIAN_POINT('Ctrl Pts',(-18.4169942498921,37.071859926622,6.22143344611464));
#63961=CARTESIAN_POINT('Ctrl Pts',(-18.4777124781656,37.0765368349428,6.23873056012735));
#63962=CARTESIAN_POINT('Ctrl Pts',(-18.5373524530954,37.0812137432636,6.25936873287877));
#63963=CARTESIAN_POINT('Ctrl Pts',(-18.5958136083621,37.0857982097029,6.27959897984085));
#63964=CARTESIAN_POINT('Ctrl Pts',(-18.6532382425253,37.0903826761423,6.30303923706746));
#63965=CARTESIAN_POINT('Ctrl Pts',(-18.709253640683,37.0949671425816,6.32955721847559));
#63966=CARTESIAN_POINT('Ctrl Pts',(-18.7652347857919,37.0995488056498,6.35605898431197));
#63967=CARTESIAN_POINT('Ctrl Pts',(-18.8198079444288,37.104130468718,6.38563452521911));
#63968=CARTESIAN_POINT('Ctrl Pts',(-18.8726205756487,37.1087121317862,6.41810353553407));
#63969=CARTESIAN_POINT('Ctrl Pts',(-18.9254203127977,37.1132926762528,6.45056461862197));
#63970=CARTESIAN_POINT('Ctrl Pts',(-18.9764599423223,37.1178732207195,6.48591750224651));
#63971=CARTESIAN_POINT('Ctrl Pts',(-19.0254135278729,37.1224537651862,6.52393707749591));
#63972=CARTESIAN_POINT('Ctrl Pts',(-19.0761559149126,37.127201686254,6.56334591712811));
#63973=CARTESIAN_POINT('Ctrl Pts',(-19.1246563563058,37.1319496073218,6.60561980035016));
#63974=CARTESIAN_POINT('Ctrl Pts',(-19.1705889294188,37.1366975283896,6.65046203964559));
#63975=CARTESIAN_POINT('Ctrl Pts',(-19.2149584064208,37.1412838766029,6.69377828714254));
#63976=CARTESIAN_POINT('Ctrl Pts',(-19.2569316840539,37.1458702248161,6.73949044725619));
#63977=CARTESIAN_POINT('Ctrl Pts',(-19.2962541270393,37.1504565730293,6.78729509622795));
#63978=CARTESIAN_POINT('Ctrl Pts',(-19.3376545105999,37.1552852805244,6.83762591631826));
#63979=CARTESIAN_POINT('Ctrl Pts',(-19.3761157400387,37.1601139880195,6.89027599323749));
#63980=CARTESIAN_POINT('Ctrl Pts',(-19.4113923459179,37.1649426955146,6.94485634215672));
#63981=CARTESIAN_POINT('Ctrl Pts',(-19.4466689517971,37.1697714030097,6.99943669107596));
#63982=CARTESIAN_POINT('Ctrl Pts',(-19.4787606806699,37.1746001105048,7.05594670850606));
#63983=CARTESIAN_POINT('Ctrl Pts',(-19.5074795664588,37.1794288179999,7.11397023229836));
#63984=CARTESIAN_POINT('Ctrl Pts',(-19.536746626648,37.1843496938979,7.17310128549139));
#63985=CARTESIAN_POINT('Ctrl Pts',(-19.5626186445621,37.189270569796,7.23401934030263));
#63986=CARTESIAN_POINT('Ctrl Pts',(-19.5848908154516,37.194191445694,7.29632735285786));
#63987=CARTESIAN_POINT('Ctrl Pts',(-19.6071102296406,37.1991006653786,7.35848777471911));
#63988=CARTESIAN_POINT('Ctrl Pts',(-19.6257466238498,37.2040098850632,7.42203123622437));
#63989=CARTESIAN_POINT('Ctrl Pts',(-19.6406421908275,37.2089191047479,7.48653898549725));
#63990=CARTESIAN_POINT('Ctrl Pts',(-19.6554847312632,37.2138108481629,7.55081709444244));
#63991=CARTESIAN_POINT('Ctrl Pts',(-19.6666128741679,37.2187025915779,7.61605227192819));
#63992=CARTESIAN_POINT('Ctrl Pts',(-19.67391847149,37.223594334993,7.68181113862676));
#63993=CARTESIAN_POINT('Ctrl Pts',(-19.6808359448899,37.2282261951217,7.7440764389353));
#63994=CARTESIAN_POINT('Ctrl Pts',(-19.6843265124556,37.2328580552504,7.80681084541127));
#63995=CARTESIAN_POINT('Ctrl Pts',(-19.6843399609503,37.2374899153791,7.86963516025696));
#63996=CARTESIAN_POINT('',(-19.6843392863112,38.0312399154724,7.87155972316893));
#63997=CARTESIAN_POINT('Ctrl Pts',(-19.6843399609504,37.2374899154299,7.86963516094604));
#63998=CARTESIAN_POINT('Ctrl Pts',(-19.6843536852301,37.2422167689179,7.93374791986184));
#63999=CARTESIAN_POINT('Ctrl Pts',(-19.6807454522696,37.2469436224059,7.997816708416));
#64000=CARTESIAN_POINT('Ctrl Pts',(-19.6735561124232,37.2516704758939,8.06142238550903));
#64001=CARTESIAN_POINT('Ctrl Pts',(-19.666351501998,37.2564073694956,8.12516316478537));
#64002=CARTESIAN_POINT('Ctrl Pts',(-19.6555506461615,37.2611442630972,8.1884384083136));
#64003=CARTESIAN_POINT('Ctrl Pts',(-19.641246022369,37.2658811566989,8.25083656437254));
#64004=CARTESIAN_POINT('Ctrl Pts',(-19.626925838286,37.2706232030009,8.31330259592769));
#64005=CARTESIAN_POINT('Ctrl Pts',(-19.6090944222083,37.275365249303,8.37488919608283));
#64006=CARTESIAN_POINT('Ctrl Pts',(-19.5878940580458,37.280107295605,8.43520043674885));
#64007=CARTESIAN_POINT('Ctrl Pts',(-19.5666396590223,37.2848614282943,8.49566539692065));
#64008=CARTESIAN_POINT('Ctrl Pts',(-19.5419993287653,37.2896155609837,8.5548480739591));
#64009=CARTESIAN_POINT('Ctrl Pts',(-19.5141633684383,37.294369693673,8.61237294841746));
#64010=CARTESIAN_POINT('Ctrl Pts',(-19.492506734948,37.2980684526886,8.65712783052259));
#64011=CARTESIAN_POINT('Ctrl Pts',(-19.4689167756715,37.3017672117043,8.70087966610814));
#64012=CARTESIAN_POINT('Ctrl Pts',(-19.4435012733911,37.3054659707199,8.7434637132604));
#64013=CARTESIAN_POINT('Ctrl Pts',(-19.4119128259435,37.3100630883962,8.79639062065462));
#64014=CARTESIAN_POINT('Ctrl Pts',(-19.3773846770101,37.3146602060725,8.84771045137129));
#64015=CARTESIAN_POINT('Ctrl Pts',(-19.3401055008303,37.3192573237488,8.89707733993657));
#64016=CARTESIAN_POINT('Ctrl Pts',(-19.3021792823753,37.3239342320692,8.94730107318484));
#64017=CARTESIAN_POINT('Ctrl Pts',(-19.2614058188731,37.3286111403897,8.99550292036121));
#64018=CARTESIAN_POINT('Ctrl Pts',(-19.2180321156265,37.3332880487102,9.04134594218678));
#64019=CARTESIAN_POINT('Ctrl Pts',(-19.1755157194584,37.337872515152,9.08628284938134));
#64020=CARTESIAN_POINT('Ctrl Pts',(-19.1305013054072,37.3424569815939,9.12895294194383));
#64021=CARTESIAN_POINT('Ctrl Pts',(-19.0832629494496,37.3470414480358,9.16907109119239));
#64022=CARTESIAN_POINT('Ctrl Pts',(-19.036053479437,37.3516231111065,9.20916470845568));
#64023=CARTESIAN_POINT('Ctrl Pts',(-18.9866231512652,37.3562047741772,9.24670914778248));
#64024=CARTESIAN_POINT('Ctrl Pts',(-18.9352814865172,37.360786437248,9.28145744431685));
#64025=CARTESIAN_POINT('Ctrl Pts',(-18.8839523567072,37.3653669817172,9.31619725714222));
#64026=CARTESIAN_POINT('Ctrl Pts',(-18.830713238088,37.3699475261864,9.34814199716612));
#64027=CARTESIAN_POINT('Ctrl Pts',(-18.7759035180666,37.3745280706556,9.37708739810577));
#64028=CARTESIAN_POINT('Ctrl Pts',(-18.7190910089807,37.379275991721,9.40709048612073));
#64029=CARTESIAN_POINT('Ctrl Pts',(-18.6605913795709,37.3840239127864,9.43387046693361));
#64030=CARTESIAN_POINT('Ctrl Pts',(-18.6008092348783,37.3887718338517,9.45725257268333));
#64031=CARTESIAN_POINT('Ctrl Pts',(-18.5430614903669,37.3933581820674,9.47983897997796));
#64032=CARTESIAN_POINT('Ctrl Pts',(-18.4841176462316,37.3979445302831,9.49925497493416));
#64033=CARTESIAN_POINT('Ctrl Pts',(-18.4243590797133,37.4025308784989,9.51539352249738));
#64034=CARTESIAN_POINT('Ctrl Pts',(-18.3614426537952,37.407359585989,9.53238488944856));
#64035=CARTESIAN_POINT('Ctrl Pts',(-18.297623641445,37.4121882934792,9.54574267457664));
#64036=CARTESIAN_POINT('Ctrl Pts',(-18.233357608423,37.4170170009694,9.55540344067946));
#64037=CARTESIAN_POINT('Ctrl Pts',(-18.169091575401,37.4218457084596,9.56506420678228));
#64038=CARTESIAN_POINT('Ctrl Pts',(-18.1043791760181,37.4266744159498,9.57102797151584));
#64039=CARTESIAN_POINT('Ctrl Pts',(-18.039677052535,37.4315031234399,9.57329489079276));
#64040=CARTESIAN_POINT('Ctrl Pts',(-17.9780781099484,37.4361002411146,9.57545308627184));
#64041=CARTESIAN_POINT('Ctrl Pts',(-17.9162354219735,37.4406973587893,9.57426985564187));
#64042=CARTESIAN_POINT('Ctrl Pts',(-17.8545418994593,37.445294476464,9.5697161823695));
#64043=CARTESIAN_POINT('Ctrl Pts',(-17.7917775829474,37.4499713847847,9.56508347250123));
#64044=CARTESIAN_POINT('Ctrl Pts',(-17.7291681861668,37.4546482931054,9.55696209132066));
#64045=CARTESIAN_POINT('Ctrl Pts',(-17.6671307498133,37.459325201426,9.54537687338927));
#64046=CARTESIAN_POINT('Ctrl Pts',(-17.6063195203642,37.4639096678663,9.5340206441952));
#64047=CARTESIAN_POINT('Ctrl Pts',(-17.5460583715777,37.4684941343065,9.51933635953746));
#64048=CARTESIAN_POINT('Ctrl Pts',(-17.4867354908501,37.4730786007467,9.50139969339616));
#64049=CARTESIAN_POINT('Ctrl Pts',(-17.4274488856753,37.4776602638157,9.48347399540867));
#64050=CARTESIAN_POINT('Ctrl Pts',(-17.3690998971863,37.4822419268848,9.46230000647829));
#64051=CARTESIAN_POINT('Ctrl Pts',(-17.3120638670408,37.4868235899538,9.43800387687261));
#64052=CARTESIAN_POINT('Ctrl Pts',(-17.2550417620984,37.4914041344213,9.41371367910577));
#64053=CARTESIAN_POINT('Ctrl Pts',(-17.1993324472942,37.4959846788889,9.38630305328262));
#64054=CARTESIAN_POINT('Ctrl Pts',(-17.1452915827475,37.5005652233564,9.35594639666704));
#64055=CARTESIAN_POINT('Ctrl Pts',(-17.0892760236635,37.5053131444233,9.32448048459283));
#64056=CARTESIAN_POINT('Ctrl Pts',(-17.0350537472118,37.5100610654903,9.28984930279165));
#64057=CARTESIAN_POINT('Ctrl Pts',(-16.9829909923909,37.5148089865573,9.25229804107014));
#64058=CARTESIAN_POINT('Ctrl Pts',(-16.932699945168,37.5193953347713,9.21602465747729));
#64059=CARTESIAN_POINT('Ctrl Pts',(-16.8844241595334,37.5239816829853,9.17702714293662));
#64060=CARTESIAN_POINT('Ctrl Pts',(-16.8384603688678,37.5285680311993,9.13556789867421));
#64061=CARTESIAN_POINT('Ctrl Pts',(-16.7900676847417,37.5333967386927,9.09191779752615));
#64062=CARTESIAN_POINT('Ctrl Pts',(-16.7442385827226,37.5382254461862,9.04553902894649));
#64063=CARTESIAN_POINT('Ctrl Pts',(-16.7012733928838,37.5430541536796,8.99677996958283));
#64064=CARTESIAN_POINT('Ctrl Pts',(-16.658308203045,37.547882861173,8.94802091021918));
#64065=CARTESIAN_POINT('Ctrl Pts',(-16.6182072653493,37.5527115686665,8.89688211941023));
#64066=CARTESIAN_POINT('Ctrl Pts',(-16.5812180614224,37.5575402761599,8.84374736143876));
#64067=CARTESIAN_POINT('Ctrl Pts',(-16.5460028980728,37.5621373938347,8.79316100155934));
#64068=CARTESIAN_POINT('Ctrl Pts',(-16.5134630960846,37.5667345115094,8.74055796574083));
#64069=CARTESIAN_POINT('Ctrl Pts',(-16.4838360902121,37.5713316291842,8.68625265123493));
#64070=CARTESIAN_POINT('Ctrl Pts',(-16.4536948582306,37.5760085375049,8.6310047774069));
#64071=CARTESIAN_POINT('Ctrl Pts',(-16.4265688806328,37.5806854458255,8.5739953506703));
#64072=CARTESIAN_POINT('Ctrl Pts',(-16.4026634297552,37.5853623541462,8.51558824320787));
#64073=CARTESIAN_POINT('Ctrl Pts',(-16.3792304843616,37.5899468205864,8.45833558703483));
#64074=CARTESIAN_POINT('Ctrl Pts',(-16.3588921153774,37.5945312870267,8.399740493246));
#64075=CARTESIAN_POINT('Ctrl Pts',(-16.3417952332691,37.599115753467,8.34017015841104));
#64076=CARTESIAN_POINT('Ctrl Pts',(-16.3247088057923,37.6036974165361,8.28063625044553));
#64077=CARTESIAN_POINT('Ctrl Pts',(-16.3108600750346,37.6082790796052,8.22012877221842));
#64078=CARTESIAN_POINT('Ctrl Pts',(-16.3003465747455,37.6128607426743,8.15903149764472));
#64079=CARTESIAN_POINT('Ctrl Pts',(-16.289835641301,37.6174412871418,8.09794913981678));
#64080=CARTESIAN_POINT('Ctrl Pts',(-16.2826584081404,37.6220218316094,8.03627777297429));
#64081=CARTESIAN_POINT('Ctrl Pts',(-16.2788611987016,37.626602376077,7.97441079598));
#64082=CARTESIAN_POINT('Ctrl Pts',(-16.2749252363249,37.6313502971439,7.91028315231327));
#64083=CARTESIAN_POINT('Ctrl Pts',(-16.2746211964079,37.6360982182108,7.84594590356721));
#64084=CARTESIAN_POINT('Ctrl Pts',(-16.2779416574722,37.6408461392777,7.78183972418737));
#64085=CARTESIAN_POINT('Ctrl Pts',(-16.2811491224778,37.6454324874918,7.71991509292971));
#64086=CARTESIAN_POINT('Ctrl Pts',(-16.2877382238244,37.6500188357059,7.65820657356212));
#64087=CARTESIAN_POINT('Ctrl Pts',(-16.2976493894911,37.6546051839199,7.597105773384));
#64088=CARTESIAN_POINT('Ctrl Pts',(-16.3080842971102,37.6594338914132,7.53277618524577));
#64089=CARTESIAN_POINT('Ctrl Pts',(-16.3222019775441,37.6642625989066,7.46912095870547));
#64090=CARTESIAN_POINT('Ctrl Pts',(-16.339872570839,37.6690913063999,7.40658134293734));
#64091=CARTESIAN_POINT('Ctrl Pts',(-16.3575431641339,37.6739200138932,7.34404172716922));
#64092=CARTESIAN_POINT('Ctrl Pts',(-16.378766384666,37.6787487213866,7.28261831111605));
#64093=CARTESIAN_POINT('Ctrl Pts',(-16.4033539822187,37.6835774288799,7.22272712847324));
#64094=CARTESIAN_POINT('Ctrl Pts',(-16.4267623330982,37.688174546555,7.16570838905066));
#64095=CARTESIAN_POINT('Ctrl Pts',(-16.4533158395462,37.6927716642301,7.10984400516698));
#64096=CARTESIAN_POINT('Ctrl Pts',(-16.4828790869993,37.6973687819052,7.05550395491687));
#64097=CARTESIAN_POINT('Ctrl Pts',(-16.5129554539252,37.7020456902258,7.00022074245233));
#64098=CARTESIAN_POINT('Ctrl Pts',(-16.546146922841,37.7067225985464,6.94651580982375));
#64099=CARTESIAN_POINT('Ctrl Pts',(-16.5822590694252,37.7113995068671,6.89475893923818));
#64100=CARTESIAN_POINT('Ctrl Pts',(-16.6176574379125,37.7159839733077,6.8440250740422));
#64101=CARTESIAN_POINT('Ctrl Pts',(-16.6558617716258,37.7205684397483,6.79516340035851));
#64102=CARTESIAN_POINT('Ctrl Pts',(-16.6966432065147,37.725152906189,6.74849646624937));
#64103=CARTESIAN_POINT('Ctrl Pts',(-16.7373997038234,37.7297345692584,6.70185806866457));
#64104=CARTESIAN_POINT('Ctrl Pts',(-16.780729843283,37.7343162323279,6.65741213206746));
#64105=CARTESIAN_POINT('Ctrl Pts',(-16.8263640578861,37.7388978953973,6.61544870624472));
#64106=CARTESIAN_POINT('Ctrl Pts',(-16.8719871310106,37.7434784398653,6.5734955256868));
#64107=CARTESIAN_POINT('Ctrl Pts',(-16.9199127880098,37.7480589843332,6.5340239971402));
#64108=CARTESIAN_POINT('Ctrl Pts',(-16.9698356062,37.7526395288012,6.49728636158201));
#64109=CARTESIAN_POINT('Ctrl Pts',(-17.021582642354,37.7573874498677,6.45920630471912));
#64110=CARTESIAN_POINT('Ctrl Pts',(-17.0754751896956,37.7621353709343,6.42406420237983));
#64111=CARTESIAN_POINT('Ctrl Pts',(-17.1311389606862,37.7668832920008,6.39209277302832));
#64112=CARTESIAN_POINT('Ctrl Pts',(-17.1849084806745,37.7714696402153,6.36120933881292));
#64113=CARTESIAN_POINT('Ctrl Pts',(-17.2403300993967,37.7760559884297,6.33328440733841));
#64114=CARTESIAN_POINT('Ctrl Pts',(-17.2970424780434,37.7806423366441,6.30848027268211));
#64115=CARTESIAN_POINT('Ctrl Pts',(-17.3567517445214,37.7854710441368,6.2823653975651));
#64116=CARTESIAN_POINT('Ctrl Pts',(-17.4178913695572,37.7902997516294,6.25971053018776));
#64117=CARTESIAN_POINT('Ctrl Pts',(-17.4800201908903,37.795128459122,6.24064582546255));
#64118=CARTESIAN_POINT('Ctrl Pts',(-17.5421490122234,37.7999571666146,6.22158112073734));
#64119=CARTESIAN_POINT('Ctrl Pts',(-17.6052663801343,37.8047858741073,6.20610665802978));
#64120=CARTESIAN_POINT('Ctrl Pts',(-17.6689206569898,37.8096145815999,6.19428985861147));
#64121=CARTESIAN_POINT('Ctrl Pts',(-17.7295220087304,37.8142116992748,6.18303980514496));
#64122=CARTESIAN_POINT('Ctrl Pts',(-17.7908588977324,37.8188088169496,6.17505831790774));
#64123=CARTESIAN_POINT('Ctrl Pts',(-17.85254703312,37.8234059346245,6.17043223823424));
#64124=CARTESIAN_POINT('Ctrl Pts',(-17.9153058690002,37.8280828429451,6.16572586523116));
#64125=CARTESIAN_POINT('Ctrl Pts',(-17.9784277562297,37.8327597512658,6.16449267828212));
#64126=CARTESIAN_POINT('Ctrl Pts',(-18.041496570692,37.8374366595864,6.16676983135187));
#64127=CARTESIAN_POINT('Ctrl Pts',(-18.1033187924494,37.8420211260268,6.16900197513409));
#64128=CARTESIAN_POINT('Ctrl Pts',(-18.1650894869301,37.8466055924672,6.17460693477934));
#64129=CARTESIAN_POINT('Ctrl Pts',(-18.2264135422485,37.8511900589076,6.1835673147746));
#64130=CARTESIAN_POINT('Ctrl Pts',(-18.2877000983088,37.8557717219768,6.1925222155562));
#64131=CARTESIAN_POINT('Ctrl Pts',(-18.3485400540762,37.860353385046,6.20482839479221));
#64132=CARTESIAN_POINT('Ctrl Pts',(-18.4085435323183,37.8649350481152,6.22041663547788));
#64133=CARTESIAN_POINT('Ctrl Pts',(-18.4685323608623,37.8695155925829,6.23600107033385));
#64134=CARTESIAN_POINT('Ctrl Pts',(-18.5276846247953,37.8740961370506,6.25486584798509));
#64135=CARTESIAN_POINT('Ctrl Pts',(-18.5856227719727,37.8786766815183,6.27689112309669));
#64136=CARTESIAN_POINT('Ctrl Pts',(-18.6456780233723,37.8834246025851,6.29972121861085));
#64137=CARTESIAN_POINT('Ctrl Pts',(-18.7044281437849,37.8881725236519,6.32594710978269));
#64138=CARTESIAN_POINT('Ctrl Pts',(-18.7614746425419,37.8929204447187,6.35538050366964));
#64139=CARTESIAN_POINT('Ctrl Pts',(-18.816579835745,37.8975067929329,6.38381227235143));
#64140=CARTESIAN_POINT('Ctrl Pts',(-18.8700950818171,37.902093141147,6.41523640411495));
#64141=CARTESIAN_POINT('Ctrl Pts',(-18.9216880834359,37.9066794893612,6.44943729842194));
#64142=CARTESIAN_POINT('Ctrl Pts',(-18.97600744644,37.9115081968543,6.48544549206514));
#64143=CARTESIAN_POINT('Ctrl Pts',(-19.0281952502118,37.9163369043475,6.52453167765242));
#64144=CARTESIAN_POINT('Ctrl Pts',(-19.0779029174026,37.9211656118406,6.56639575807732));
#64145=CARTESIAN_POINT('Ctrl Pts',(-19.1276105845934,37.9259943193337,6.60825983850221));
#64146=CARTESIAN_POINT('Ctrl Pts',(-19.1748376962107,37.9308230268268,6.65290131089329));
#64147=CARTESIAN_POINT('Ctrl Pts',(-19.2192827047016,37.9356517343199,6.69997725944003));
#64148=CARTESIAN_POINT('Ctrl Pts',(-19.261067270979,37.9401913992931,6.74423527983224));
#64149=CARTESIAN_POINT('Ctrl Pts',(-19.3005741516839,37.9447310642663,6.79083660250622));
#64150=CARTESIAN_POINT('Ctrl Pts',(-19.3375250314245,37.9492707292395,6.83951437435744));
#64151=CARTESIAN_POINT('Ctrl Pts',(-19.3744237645193,37.9538039876453,6.88812345007625));
#64152=CARTESIAN_POINT('Ctrl Pts',(-19.4087733272311,37.9583372460512,6.93880275965488));
#64153=CARTESIAN_POINT('Ctrl Pts',(-19.4403330309442,37.962870504457,6.99124959497402));
#64154=CARTESIAN_POINT('Ctrl Pts',(-19.4718604788682,37.9673991296182,7.04364282668281));
#64155=CARTESIAN_POINT('Ctrl Pts',(-19.500603449484,37.9719277547794,7.09779955920494));
#64156=CARTESIAN_POINT('Ctrl Pts',(-19.5263636240853,37.9764563799406,7.15338687026699));
#64157=CARTESIAN_POINT('Ctrl Pts',(-19.5523323855609,37.9810216745647,7.20942428633192));
#64158=CARTESIAN_POINT('Ctrl Pts',(-19.5752695249026,37.9855869691888,7.26691510595684));
#64159=CARTESIAN_POINT('Ctrl Pts',(-19.5950191632529,37.9901522638129,7.32549294042587));
#64160=CARTESIAN_POINT('Ctrl Pts',(-19.6145989101356,37.9946782865987,7.38356687330028));
#64161=CARTESIAN_POINT('Ctrl Pts',(-19.6310456517359,37.9992043093846,7.44270867615168));
#64162=CARTESIAN_POINT('Ctrl Pts',(-19.6442568361512,38.0037303321704,7.50254385442078));
#64163=CARTESIAN_POINT('Ctrl Pts',(-19.6576399687168,38.0083152627136,7.56315780830188));
#64164=CARTESIAN_POINT('Ctrl Pts',(-19.6677025592785,38.0129001932569,7.62448278802777));
#64165=CARTESIAN_POINT('Ctrl Pts',(-19.6743915429074,38.0174851238001,7.68611923721124));
#64166=CARTESIAN_POINT('Ctrl Pts',(-19.6810805265363,38.0220700543433,7.74775568639472));
#64167=CARTESIAN_POINT('Ctrl Pts',(-19.6843958943194,38.0266549848866,7.80970304890221));
#64168=CARTESIAN_POINT('Ctrl Pts',(-19.6843392863117,38.0312399154298,7.87155972259389));
#64169=CARTESIAN_POINT('',(-19.6843399030359,38.8249899154737,7.86942509175251));
#64170=CARTESIAN_POINT('Ctrl Pts',(-19.6843392863112,38.0312399154724,7.87155972316893));
#64171=CARTESIAN_POINT('Ctrl Pts',(-19.6842647470063,38.0372771781012,7.95301024480486));
#64172=CARTESIAN_POINT('Ctrl Pts',(-19.6783476784105,38.0433144407299,8.03420097598546));
#64173=CARTESIAN_POINT('Ctrl Pts',(-19.6667212373974,38.0493517033586,8.11443056869534));
#64174=CARTESIAN_POINT('Ctrl Pts',(-19.6588016692553,38.053464097919,8.16908045904026));
#64175=CARTESIAN_POINT('Ctrl Pts',(-19.6482340032239,38.0575764924794,8.22328503262939));
#64176=CARTESIAN_POINT('Ctrl Pts',(-19.6350725347685,38.0616888870398,8.27682888326031));
#64177=CARTESIAN_POINT('Ctrl Pts',(-19.6203597394925,38.0662860047145,8.33668388464538));
#64178=CARTESIAN_POINT('Ctrl Pts',(-19.6023655918517,38.0708831223893,8.39586267089081));
#64179=CARTESIAN_POINT('Ctrl Pts',(-19.5811692648634,38.075480240064,8.45397929831186));
#64180=CARTESIAN_POINT('Ctrl Pts',(-19.5596050402617,38.0801571483847,8.5131046367489));
#64181=CARTESIAN_POINT('Ctrl Pts',(-19.5347264522261,38.0848340567053,8.57113005579009));
#64182=CARTESIAN_POINT('Ctrl Pts',(-19.506671062814,38.089510965026,8.62766107301773));
#64183=CARTESIAN_POINT('Ctrl Pts',(-19.4791702048946,38.0940954314663,8.68307472099748));
#64184=CARTESIAN_POINT('Ctrl Pts',(-19.4486172226179,38.0986798979065,8.73705202681293));
#64185=CARTESIAN_POINT('Ctrl Pts',(-19.415190728452,38.1032643643468,8.78924012562842));
#64186=CARTESIAN_POINT('Ctrl Pts',(-19.3817846743683,38.1078460274159,8.84139631176353));
#64187=CARTESIAN_POINT('Ctrl Pts',(-19.3455088665287,38.112427690485,8.89176503251976));
#64188=CARTESIAN_POINT('Ctrl Pts',(-19.3065869814173,38.1170093535541,8.94001954016465));
#64189=CARTESIAN_POINT('Ctrl Pts',(-19.2676745989861,38.1215898980217,8.98826226659303));
#64190=CARTESIAN_POINT('Ctrl Pts',(-19.2261177412154,38.1261704424893,9.034391408535));
#64191=CARTESIAN_POINT('Ctrl Pts',(-19.1821811405647,38.1307509869569,9.07811230474259));
#64192=CARTESIAN_POINT('Ctrl Pts',(-19.1366390629114,38.1354989080238,9.12343079594752));
#64193=CARTESIAN_POINT('Ctrl Pts',(-19.08854032802,38.1402468290907,9.1661611799655));
#64194=CARTESIAN_POINT('Ctrl Pts',(-19.0382206640004,38.1449947501577,9.20601791226113));
#64195=CARTESIAN_POINT('Ctrl Pts',(-18.9896133897941,38.1495810983717,9.24451831073169));
#64196=CARTESIAN_POINT('Ctrl Pts',(-18.938934397463,38.1541674465858,9.28033726319256));
#64197=CARTESIAN_POINT('Ctrl Pts',(-18.886517030594,38.1587537947999,9.31326079030887));
#64198=CARTESIAN_POINT('Ctrl Pts',(-18.8313297398854,38.1635825022933,9.3479241160471));
#64199=CARTESIAN_POINT('Ctrl Pts',(-18.7742158154267,38.1684112097866,9.37937719856032));
#64200=CARTESIAN_POINT('Ctrl Pts',(-18.71559230145,38.1732399172799,9.40742603127677));
#64201=CARTESIAN_POINT('Ctrl Pts',(-18.6569687874734,38.1780686247733,9.43547486399322));
#64202=CARTESIAN_POINT('Ctrl Pts',(-18.5968363148,38.1828973322666,9.46011927227349));
#64203=CARTESIAN_POINT('Ctrl Pts',(-18.535631571236,38.18772603976,9.48122574229863));
#64204=CARTESIAN_POINT('Ctrl Pts',(-18.4773622706411,38.1923231574347,9.50131992413451));
#64205=CARTESIAN_POINT('Ctrl Pts',(-18.4178818376672,38.1969202751094,9.51829037444914));
#64206=CARTESIAN_POINT('Ctrl Pts',(-18.3575574810139,38.2015173927841,9.53199433937978));
#64207=CARTESIAN_POINT('Ctrl Pts',(-18.2961860945205,38.2061943011047,9.54593615948215));
#64208=CARTESIAN_POINT('Ctrl Pts',(-18.2339416800988,38.2108712094254,9.55649675940762));
#64209=CARTESIAN_POINT('Ctrl Pts',(-18.1712302821058,38.2155481177461,9.56357781480679));
#64210=CARTESIAN_POINT('Ctrl Pts',(-18.1097584122707,38.2201325841863,9.57051890892562));
#64211=CARTESIAN_POINT('Ctrl Pts',(-18.04783838168,38.2247170506265,9.57411669721915));
#64212=CARTESIAN_POINT('Ctrl Pts',(-17.9858635262238,38.2293015170667,9.57432991367875));
#64213=CARTESIAN_POINT('Ctrl Pts',(-17.9239265679857,38.2338831801358,9.57454299975788));
#64214=CARTESIAN_POINT('Ctrl Pts',(-17.8619353593724,38.2384648432048,9.5713756160478));
#64215=CARTESIAN_POINT('Ctrl Pts',(-17.8002857279752,38.2430465062738,9.56483852211076));
#64216=CARTESIAN_POINT('Ctrl Pts',(-17.7386511481802,38.2476270507413,9.55830302418874));
#64217=CARTESIAN_POINT('Ctrl Pts',(-17.6773584860604,38.2522075952089,9.54839950288427));
#64218=CARTESIAN_POINT('Ctrl Pts',(-17.6167988719718,38.2567881396764,9.53519061257235));
#64219=CARTESIAN_POINT('Ctrl Pts',(-17.5540263632502,38.2615360607433,9.52149905930226));
#64220=CARTESIAN_POINT('Ctrl Pts',(-17.4920420944869,38.2662839818103,9.50425596090198));
#64221=CARTESIAN_POINT('Ctrl Pts',(-17.4312680331346,38.2710319028773,9.48358856718186));
#64222=CARTESIAN_POINT('Ctrl Pts',(-17.3725621271581,38.2756182510913,9.46362448965411));
#64223=CARTESIAN_POINT('Ctrl Pts',(-17.3149858427328,38.2802045993053,9.4404657096611));
#64224=CARTESIAN_POINT('Ctrl Pts',(-17.2588997238343,38.2847909475193,9.41427627946355));
#64225=CARTESIAN_POINT('Ctrl Pts',(-17.1998498109263,38.2896196550127,9.38670290475604));
#64226=CARTESIAN_POINT('Ctrl Pts',(-17.1424524967901,38.2944483625061,9.35576999191488));
#64227=CARTESIAN_POINT('Ctrl Pts',(-17.0870969302704,38.2992770699996,9.3217227502755));
#64228=CARTESIAN_POINT('Ctrl Pts',(-17.0317413637507,38.304105777493,9.28767550863611));
#64229=CARTESIAN_POINT('Ctrl Pts',(-16.9784280336437,38.3089344849864,9.2505143735293));
#64230=CARTESIAN_POINT('Ctrl Pts',(-16.9275059132598,38.3137631924799,9.21053386118251));
#64231=CARTESIAN_POINT('Ctrl Pts',(-16.8790260705578,38.3183603101563,9.17247085565352));
#64232=CARTESIAN_POINT('Ctrl Pts',(-16.8325141158567,38.3229574278327,9.13169640086473));
#64233=CARTESIAN_POINT('Ctrl Pts',(-16.7882891113365,38.3275545455091,9.08844162496235));
#64234=CARTESIAN_POINT('Ctrl Pts',(-16.7432965081072,38.3322314538295,9.0444360902866));
#64235=CARTESIAN_POINT('Ctrl Pts',(-16.7006714757945,38.3369083621499,8.99786356601203));
#64236=CARTESIAN_POINT('Ctrl Pts',(-16.6607168045294,38.3415852704704,8.94901190250561));
#64237=CARTESIAN_POINT('Ctrl Pts',(-16.6215518611389,38.3461697369123,8.90112582122455));
#64238=CARTESIAN_POINT('Ctrl Pts',(-16.5849530149872,38.3507542033542,8.85105029095318));
#64239=CARTESIAN_POINT('Ctrl Pts',(-16.5511682235539,38.3553386697962,8.79909342383743));
#64240=CARTESIAN_POINT('Ctrl Pts',(-16.5174040912993,38.3599203328669,8.74716832800546));
#64241=CARTESIAN_POINT('Ctrl Pts',(-16.4864508786603,38.3645019959376,8.69336460234608));
#64242=CARTESIAN_POINT('Ctrl Pts',(-16.4585141813327,38.3690836590084,8.63802066325994));
#64243=CARTESIAN_POINT('Ctrl Pts',(-16.4305843046794,38.3736642034776,8.58269023625722));
#64244=CARTESIAN_POINT('Ctrl Pts',(-16.4056697106306,38.3782447479468,8.52582079657356));
#64245=CARTESIAN_POINT('Ctrl Pts',(-16.3839298447886,38.3828252924161,8.46777495367685));
#64246=CARTESIAN_POINT('Ctrl Pts',(-16.3613955876316,38.3875732134814,8.40760807131273));
#64247=CARTESIAN_POINT('Ctrl Pts',(-16.3422728282833,38.3923211345467,8.3461776709531));
#64248=CARTESIAN_POINT('Ctrl Pts',(-16.3266834593055,38.397069055612,8.2839072986381));
#64249=CARTESIAN_POINT('Ctrl Pts',(-16.3116246001519,38.4016554038277,8.22375600146463));
#64250=CARTESIAN_POINT('Ctrl Pts',(-16.2998625255837,38.4062417520434,8.16282151842348));
#64251=CARTESIAN_POINT('Ctrl Pts',(-16.2914548993661,38.410828100259,8.10149574234817));
#64252=CARTESIAN_POINT('Ctrl Pts',(-16.2826029836846,38.4156568077492,8.03692928983553));
#64253=CARTESIAN_POINT('Ctrl Pts',(-16.2774699332461,38.4204855152393,7.9719296855735));
#64254=CARTESIAN_POINT('Ctrl Pts',(-16.2760607329453,38.4253142227295,7.90695686389569));
#64255=CARTESIAN_POINT('Ctrl Pts',(-16.2746515326445,38.4301429302196,7.84198404221788));
#64256=CARTESIAN_POINT('Ctrl Pts',(-16.2769660817559,38.4349716377098,7.77703864987683));
#64257=CARTESIAN_POINT('Ctrl Pts',(-16.2829461515228,38.4398003451999,7.71257360142368));
#64258=CARTESIAN_POINT('Ctrl Pts',(-16.2886394109438,38.4443974628727,7.65120036352823));
#64259=CARTESIAN_POINT('Ctrl Pts',(-16.2976779631414,38.4489945805455,7.59001030990863));
#64260=CARTESIAN_POINT('Ctrl Pts',(-16.3100406200581,38.4535916982182,7.5293968512415));
#64261=CARTESIAN_POINT('Ctrl Pts',(-16.3226178515145,38.4582686065391,7.46773134485735));
#64262=CARTESIAN_POINT('Ctrl Pts',(-16.3386357245529,38.46294551486,7.40666317686714));
#64263=CARTESIAN_POINT('Ctrl Pts',(-16.3580165685392,38.4676224231809,7.34660284327611));
#64264=CARTESIAN_POINT('Ctrl Pts',(-16.377014338584,38.4722068896193,7.28772963800249));
#64265=CARTESIAN_POINT('Ctrl Pts',(-16.3992431834038,38.4767913560576,7.22982529685084));
#64266=CARTESIAN_POINT('Ctrl Pts',(-16.4245786752141,38.4813758224959,7.1732652312385));
#64267=CARTESIAN_POINT('Ctrl Pts',(-16.4498986745371,38.4859574855631,7.11673975173547));
#64268=CARTESIAN_POINT('Ctrl Pts',(-16.478321346364,38.4905391486302,7.06155738146749));
#64269=CARTESIAN_POINT('Ctrl Pts',(-16.5096738301586,38.4951208116974,7.00807437102755));
#64270=CARTESIAN_POINT('Ctrl Pts',(-16.5410186593234,38.499701356163,6.9546044183297));
#64271=CARTESIAN_POINT('Ctrl Pts',(-16.5752916231351,38.5042819006287,6.90283344081562));
#64272=CARTESIAN_POINT('Ctrl Pts',(-16.6122745088481,38.5088624450944,6.85309203147319));
#64273=CARTESIAN_POINT('Ctrl Pts',(-16.6506087775312,38.5136103661631,6.80153303293523));
#64274=CARTESIAN_POINT('Ctrl Pts',(-16.6918545511307,38.5183582872319,6.75215530333725));
#64275=CARTESIAN_POINT('Ctrl Pts',(-16.7357220538011,38.5231062083007,6.70529092550838));
#64276=CARTESIAN_POINT('Ctrl Pts',(-16.7780967351684,38.527692556513,6.66002135334033));
#64277=CARTESIAN_POINT('Ctrl Pts',(-16.8229171341829,38.5322789047252,6.6170971241885));
#64278=CARTESIAN_POINT('Ctrl Pts',(-16.8698852428082,38.5368652529374,6.5767791907547));
#64279=CARTESIAN_POINT('Ctrl Pts',(-16.9193353167557,38.5416939604345,6.53433071139147));
#64280=CARTESIAN_POINT('Ctrl Pts',(-16.9711658745846,38.5465226679316,6.49477202020484));
#64281=CARTESIAN_POINT('Ctrl Pts',(-17.0249931735315,38.5513513754286,6.45835670334232));
#64282=CARTESIAN_POINT('Ctrl Pts',(-17.0788204724784,38.5561800829257,6.42194138647981));
#64283=CARTESIAN_POINT('Ctrl Pts',(-17.1346439145111,38.5610087904228,6.38866971000909));
#64284=CARTESIAN_POINT('Ctrl Pts',(-17.1920513776488,38.5658374979199,6.35873834028158));
#64285=CARTESIAN_POINT('Ctrl Pts',(-17.246705519273,38.5704346155938,6.33024251011107));
#64286=CARTESIAN_POINT('Ctrl Pts',(-17.3030197188883,38.5750317332678,6.30465679122923));
#64287=CARTESIAN_POINT('Ctrl Pts',(-17.360651936019,38.5796288509418,6.28217670654351));
#64288=CARTESIAN_POINT('Ctrl Pts',(-17.4192844564284,38.5843057592625,6.25930644248358));
#64289=CARTESIAN_POINT('Ctrl Pts',(-17.4792807570035,38.5889826675833,6.23965097722091));
#64290=CARTESIAN_POINT('Ctrl Pts',(-17.5402538143679,38.593659575904,6.22336764035745));
#64291=CARTESIAN_POINT('Ctrl Pts',(-17.6000217029012,38.5982440423434,6.20740615335526));
#64292=CARTESIAN_POINT('Ctrl Pts',(-17.6607275715857,38.6028285087829,6.19468484152293));
#64293=CARTESIAN_POINT('Ctrl Pts',(-17.7219885219032,38.6074129752223,6.18530272370069));
#64294=CARTESIAN_POINT('Ctrl Pts',(-17.7832120115507,38.6119946382905,6.17592634298207));
#64295=CARTESIAN_POINT('Ctrl Pts',(-17.8449894076318,38.6165763013587,6.16988518440796));
#64296=CARTESIAN_POINT('Ctrl Pts',(-17.9069276484411,38.6211579644269,6.16722718278754));
#64297=CARTESIAN_POINT('Ctrl Pts',(-17.9688507671847,38.6257385088936,6.16456983011153));
#64298=CARTESIAN_POINT('Ctrl Pts',(-18.0309341443209,38.6303190533603,6.1652940164994));
#64299=CARTESIAN_POINT('Ctrl Pts',(-18.0927816840925,38.6348995978269,6.16939565820463));
#64300=CARTESIAN_POINT('Ctrl Pts',(-18.1568891803095,38.6396475188947,6.17364717703744));
#64301=CARTESIAN_POINT('Ctrl Pts',(-18.220742684882,38.6443954399624,6.18152778436431));
#64302=CARTESIAN_POINT('Ctrl Pts',(-18.2839060454256,38.6491433610302,6.19297407558686));
#64303=CARTESIAN_POINT('Ctrl Pts',(-18.3449199421671,38.6537297092433,6.20403084686557));
#64304=CARTESIAN_POINT('Ctrl Pts',(-18.4052894175494,38.6583160574564,6.21841431166702));
#64305=CARTESIAN_POINT('Ctrl Pts',(-18.4646336202325,38.6629024056696,6.23601557848909));
#64306=CARTESIAN_POINT('Ctrl Pts',(-18.5271137859259,38.6677311131646,6.25454696011923));
#64307=CARTESIAN_POINT('Ctrl Pts',(-18.5884567040379,38.6725598206597,6.27664544801783));
#64308=CARTESIAN_POINT('Ctrl Pts',(-18.6482412234039,38.6773885281547,6.30212612020491));
#64309=CARTESIAN_POINT('Ctrl Pts',(-18.7080257427699,38.6822172356498,6.32760679239199));
#64310=CARTESIAN_POINT('Ctrl Pts',(-18.7662513155538,38.6870459431449,6.3564692906635));
#64311=CARTESIAN_POINT('Ctrl Pts',(-18.8225292271859,38.6918746506399,6.3884739837122));
#64312=CARTESIAN_POINT('Ctrl Pts',(-18.8761079919265,38.6964717683256,6.41894369855634));
#64313=CARTESIAN_POINT('Ctrl Pts',(-18.9281417848448,38.7010688860113,6.45238622392788));
#64314=CARTESIAN_POINT('Ctrl Pts',(-18.978280853558,38.7056660036971,6.48862019233682));
#64315=CARTESIAN_POINT('Ctrl Pts',(-19.0292901693113,38.7103429120164,6.52548306161227));
#64316=CARTESIAN_POINT('Ctrl Pts',(-19.0783378532749,38.7150198203356,6.5652350186936));
#64317=CARTESIAN_POINT('Ctrl Pts',(-19.1250818520133,38.7196967286549,6.60763619039921));
#64318=CARTESIAN_POINT('Ctrl Pts',(-19.1709019278808,38.7242811951062,6.64919927778709));
#64319=CARTESIAN_POINT('Ctrl Pts',(-19.2145081616957,38.7288656615575,6.69330744776144));
#64320=CARTESIAN_POINT('Ctrl Pts',(-19.255609730549,38.7334501280088,6.73969267412414));
#64321=CARTESIAN_POINT('Ctrl Pts',(-19.2966861660623,38.7380317910889,6.78604953622483));
#64322=CARTESIAN_POINT('Ctrl Pts',(-19.3352606366053,38.742613454169,6.83468031355844));
#64323=CARTESIAN_POINT('Ctrl Pts',(-19.3710797301173,38.747195117249,6.88528074048647));
#64324=CARTESIAN_POINT('Ctrl Pts',(-19.4068900784875,38.7517756617276,6.93586881344735));
#64325=CARTESIAN_POINT('Ctrl Pts',(-19.4399460912709,38.7563562062061,6.98842516605705));
#64326=CARTESIAN_POINT('Ctrl Pts',(-19.4700364182083,38.7609367506847,7.04261477653218));
#64327=CARTESIAN_POINT('Ctrl Pts',(-19.501226268569,38.765684671741,7.09878451657302));
#64328=CARTESIAN_POINT('Ctrl Pts',(-19.529229161916,38.7704325927972,7.15670870806836));
#64329=CARTESIAN_POINT('Ctrl Pts',(-19.5538618699681,38.7751805138535,7.2159865063621));
#64330=CARTESIAN_POINT('Ctrl Pts',(-19.577656321373,38.7797668620783,7.27324706772241));
#64331=CARTESIAN_POINT('Ctrl Pts',(-19.598306184779,38.7843532103032,7.33177006130215));
#64332=CARTESIAN_POINT('Ctrl Pts',(-19.6156964376789,38.788939558528,7.39117644234587));
#64333=CARTESIAN_POINT('Ctrl Pts',(-19.6340056545113,38.793768266,7.45372207167173));
#64334=CARTESIAN_POINT('Ctrl Pts',(-19.6487010506658,38.798596973472,7.51724641394041));
#64335=CARTESIAN_POINT('Ctrl Pts',(-19.6597096334922,38.803425680944,7.58129533645361));
#64336=CARTESIAN_POINT('Ctrl Pts',(-19.6707182163187,38.8082543884159,7.64534425896682));
#64337=CARTESIAN_POINT('Ctrl Pts',(-19.678039989725,38.8130830958879,7.70991710718719));
#64338=CARTESIAN_POINT('Ctrl Pts',(-19.6816655175308,38.8179118033599,7.77455733633969));
#64339=CARTESIAN_POINT('Ctrl Pts',(-19.6834369986343,38.8202711740499,7.80614141198337));
#64340=CARTESIAN_POINT('Ctrl Pts',(-19.684329226899,38.8226305447399,7.83777526298266));
#64341=CARTESIAN_POINT('Ctrl Pts',(-19.6843399030357,38.8249899154298,7.86942509116366));
#64342=CARTESIAN_POINT('',(-19.6843395759433,39.6187399153728,7.8687977216301));
#64343=CARTESIAN_POINT('Ctrl Pts',(-19.6843399030359,38.8249899154737,7.86942509175251));
#64344=CARTESIAN_POINT('Ctrl Pts',(-19.6843605266318,38.829547627553,7.93056461714531));
#64345=CARTESIAN_POINT('Ctrl Pts',(-19.68108701094,38.8341053396324,7.99183752883473));
#64346=CARTESIAN_POINT('Ctrl Pts',(-19.6745024781758,38.8386630517117,8.05285564540372));
#64347=CARTESIAN_POINT('Ctrl Pts',(-19.6679289612082,38.8432131388264,8.11377167983781));
#64348=CARTESIAN_POINT('Ctrl Pts',(-19.6580554746227,38.8477632259412,8.17443325378262));
#64349=CARTESIAN_POINT('Ctrl Pts',(-19.6449171408284,38.8523133130559,8.2344526715167));
#64350=CARTESIAN_POINT('Ctrl Pts',(-19.6317909666354,38.8568591890396,8.29441654094461));
#64351=CARTESIAN_POINT('Ctrl Pts',(-19.61540604119,38.8614050650233,8.35373892732559));
#64352=CARTESIAN_POINT('Ctrl Pts',(-19.5958490092529,38.865950941007,8.41203949569782));
#64353=CARTESIAN_POINT('Ctrl Pts',(-19.5763025908541,38.8704943499585,8.47030842453947));
#64354=CARTESIAN_POINT('Ctrl Pts',(-19.5535876426938,38.8750377589099,8.52755614371076));
#64355=CARTESIAN_POINT('Ctrl Pts',(-19.5278408334042,38.8795811678614,8.58341684171773));
#64356=CARTESIAN_POINT('Ctrl Pts',(-19.5020981414711,38.8841238502438,8.6392686066408));
#64357=CARTESIAN_POINT('Ctrl Pts',(-19.4733247686859,38.8886665326262,8.69373332027379));
#64358=CARTESIAN_POINT('Ctrl Pts',(-19.4417048915243,38.8932092150087,8.74646656849764));
#64359=CARTESIAN_POINT('Ctrl Pts',(-19.4100557842604,38.8977560967455,8.79924856448326));
#64360=CARTESIAN_POINT('Ctrl Pts',(-19.375555184547,38.9023029784823,8.85029545262463));
#64361=CARTESIAN_POINT('Ctrl Pts',(-19.3384317914997,38.9068498602192,8.89928999968087));
#64362=CARTESIAN_POINT('Ctrl Pts',(-19.3012908955347,38.9113988857174,8.94830764666006));
#64363=CARTESIAN_POINT('Ctrl Pts',(-19.2615250799658,38.9159479112156,8.99527062998618));
#64364=CARTESIAN_POINT('Ctrl Pts',(-19.2194026985627,38.9204969367138,9.0398956305566));
#64365=CARTESIAN_POINT('Ctrl Pts',(-19.1772031503065,38.925054295881,9.08460238269823));
#64366=CARTESIAN_POINT('Ctrl Pts',(-19.1326387927123,38.9296116550482,9.1269622424915));
#64367=CARTESIAN_POINT('Ctrl Pts',(-19.0860133208819,38.9341690142153,9.16673026093779));
#64368=CARTESIAN_POINT('Ctrl Pts',(-19.0526610813367,38.9374289948369,9.19517721118597));
#64369=CARTESIAN_POINT('Ctrl Pts',(-19.018254926862,38.9406889754584,9.22229878469583));
#64370=CARTESIAN_POINT('Ctrl Pts',(-18.982914803714,38.9439489560799,9.24801913342716));
#64371=CARTESIAN_POINT('Ctrl Pts',(-18.933079321978,38.9485460737539,9.28428912501935));
#64372=CARTESIAN_POINT('Ctrl Pts',(-18.8811714116231,38.9531431914279,9.3179267070985));
#64373=CARTESIAN_POINT('Ctrl Pts',(-18.8275004130645,38.9577403091019,9.34868789318622));
#64374=CARTESIAN_POINT('Ctrl Pts',(-18.7728978647845,38.9624172174226,9.37998299097858));
#64375=CARTESIAN_POINT('Ctrl Pts',(-18.7164708149572,38.9670941257434,9.40830050220937));
#64376=CARTESIAN_POINT('Ctrl Pts',(-18.6585787436045,38.9717710340641,9.43342755646948));
#64377=CARTESIAN_POINT('Ctrl Pts',(-18.6018309435631,38.9763555005031,9.45805795951889));
#64378=CARTESIAN_POINT('Ctrl Pts',(-18.5436759985838,38.980939966942,9.47962266770406));
#64379=CARTESIAN_POINT('Ctrl Pts',(-18.4844779382697,38.985524433381,9.49796708977768));
#64380=CARTESIAN_POINT('Ctrl Pts',(-18.425316077184,38.9901060964486,9.51630029435663));
#64381=CARTESIAN_POINT('Ctrl Pts',(-18.3651128507941,38.9946877595161,9.53141696704901));
#64382=CARTESIAN_POINT('Ctrl Pts',(-18.3042498995799,38.9992694225837,9.54321153421271));
#64383=CARTESIAN_POINT('Ctrl Pts',(-18.2434018079045,39.0038499670496,9.55500322176203));
#64384=CARTESIAN_POINT('Ctrl Pts',(-18.1818948107058,39.0084305115155,9.56347431709158));
#64385=CARTESIAN_POINT('Ctrl Pts',(-18.1201212469924,39.0130110559814,9.56857024339333));
#64386=CARTESIAN_POINT('Ctrl Pts',(-18.056090429958,39.0177589770496,9.57385237874434));
#64387=CARTESIAN_POINT('Ctrl Pts',(-17.9917737632777,39.0225068981178,9.575507795877));
#64388=CARTESIAN_POINT('Ctrl Pts',(-17.927611980059,39.027254819186,9.57353465798811));
#64389=CARTESIAN_POINT('Ctrl Pts',(-17.8656336372198,39.0318411673979,9.57162866643969));
#64390=CARTESIAN_POINT('Ctrl Pts',(-17.8038003251905,39.0364275156098,9.56633724512009));
#64391=CARTESIAN_POINT('Ctrl Pts',(-17.7425048162126,39.0410138638217,9.557711726948));
#64392=CARTESIAN_POINT('Ctrl Pts',(-17.6779702300848,39.0458425713181,9.5486304050917));
#64393=CARTESIAN_POINT('Ctrl Pts',(-17.6140324978053,39.0506712788145,9.53585295760223));
#64394=CARTESIAN_POINT('Ctrl Pts',(-17.5511354989815,39.0554999863108,9.51949994706461));
#64395=CARTESIAN_POINT('Ctrl Pts',(-17.4882385001577,39.0603286938072,9.503146936527));
#64396=CARTESIAN_POINT('Ctrl Pts',(-17.4263828296021,39.0651574013035,9.48321863613079));
#64397=CARTESIAN_POINT('Ctrl Pts',(-17.3659883835307,39.0699861087999,9.45989451550748));
#64398=CARTESIAN_POINT('Ctrl Pts',(-17.3084905167746,39.0745832265531,9.43768904353049));
#64399=CARTESIAN_POINT('Ctrl Pts',(-17.2520806849564,39.0791803443063,9.41231486187921));
#64400=CARTESIAN_POINT('Ctrl Pts',(-17.197131629014,39.0837774620595,9.38389958362823));
#64401=CARTESIAN_POINT('Ctrl Pts',(-17.1412288416141,39.0884543703704,9.35499111137642));
#64402=CARTESIAN_POINT('Ctrl Pts',(-17.0868385511607,39.0931312786812,9.32293507173071));
#64403=CARTESIAN_POINT('Ctrl Pts',(-17.0343345422624,39.0978081869921,9.28791807860746));
#64404=CARTESIAN_POINT('Ctrl Pts',(-16.9828683053979,39.1023926535113,9.25359321656022));
#64405=CARTESIAN_POINT('Ctrl Pts',(-16.9332149059744,39.1069771200305,9.21642368176465));
#64406=CARTESIAN_POINT('Ctrl Pts',(-16.8857016283261,39.1115615865497,9.17663151245937));
#64407=CARTESIAN_POINT('Ctrl Pts',(-16.8382174047356,39.1161432496977,9.13686367580475));
#64408=CARTESIAN_POINT('Ctrl Pts',(-16.7928710974951,39.1207249128458,9.09447671076512));
#64409=CARTESIAN_POINT('Ctrl Pts',(-16.7499583548246,39.1253065759938,9.04973403220139));
#64410=CARTESIAN_POINT('Ctrl Pts',(-16.7070560891935,39.1298871205401,9.0050022774514));
#64411=CARTESIAN_POINT('Ctrl Pts',(-16.6665865608835,39.1344676650864,8.95791631815617));
#64412=CARTESIAN_POINT('Ctrl Pts',(-16.6288083708181,39.1390482096328,8.90877621113923));
#64413=CARTESIAN_POINT('Ctrl Pts',(-16.5896497380871,39.1437961306234,8.85784048871027));
#64414=CARTESIAN_POINT('Ctrl Pts',(-16.5533833437414,39.148544051614,8.80469801499726));
#64415=CARTESIAN_POINT('Ctrl Pts',(-16.5202497170263,39.1532919726046,8.74971810653079));
#64416=CARTESIAN_POINT('Ctrl Pts',(-16.4882436342424,39.1578783208961,8.69660917532453));
#64417=CARTESIAN_POINT('Ctrl Pts',(-16.4591606981488,39.1624646691876,8.64178636464811));
#64418=CARTESIAN_POINT('Ctrl Pts',(-16.4331707571701,39.1670510174791,8.58560752450374));
#64419=CARTESIAN_POINT('Ctrl Pts',(-16.4058074147467,39.1718797248192,8.52645999350002));
#64420=CARTESIAN_POINT('Ctrl Pts',(-16.381873270837,39.1767084321594,8.46580973999901));
#64421=CARTESIAN_POINT('Ctrl Pts',(-16.3615077185165,39.1815371394995,8.40409509488335));
#64422=CARTESIAN_POINT('Ctrl Pts',(-16.3411421661961,39.1863658468396,8.3423804497677));
#64423=CARTESIAN_POINT('Ctrl Pts',(-16.3243452984608,39.1911945541798,8.27960206094635));
#64424=CARTESIAN_POINT('Ctrl Pts',(-16.3111940086415,39.1960232615199,8.21621005012255));
#64425=CARTESIAN_POINT('Ctrl Pts',(-16.2986734683704,39.20062037903,8.15585838611979));
#64426=CARTESIAN_POINT('Ctrl Pts',(-16.2894053224898,39.2052174965402,8.09470268886554));
#64427=CARTESIAN_POINT('Ctrl Pts',(-16.2834844654515,39.2098146140503,8.03312534026237));
#64428=CARTESIAN_POINT('Ctrl Pts',(-16.2774608418202,39.2144915223915,7.97047921153508));
#64429=CARTESIAN_POINT('Ctrl Pts',(-16.2749020118353,39.2191684307327,7.90739715505296));
#64430=CARTESIAN_POINT('Ctrl Pts',(-16.2758538622243,39.223845339074,7.84429442270082));
#64431=CARTESIAN_POINT('Ctrl Pts',(-16.2767868986858,39.2284298053507,7.78243895594146));
#64432=CARTESIAN_POINT('Ctrl Pts',(-16.2810930889719,39.2330142716274,7.72056415694667));
#64433=CARTESIAN_POINT('Ctrl Pts',(-16.2887633409867,39.2375987379042,7.65906541580508));
#64434=CARTESIAN_POINT('Ctrl Pts',(-16.2964289026938,39.2421804008105,7.59760428073067));
#64435=CARTESIAN_POINT('Ctrl Pts',(-16.3074543843327,39.2467620637169,7.53651925165197));
#64436=CARTESIAN_POINT('Ctrl Pts',(-16.3217787737923,39.2513437266233,7.47620157370288));
#64437=CARTESIAN_POINT('Ctrl Pts',(-16.3360996659915,39.2559242709293,7.4158986221489));
#64438=CARTESIAN_POINT('Ctrl Pts',(-16.3537177495671,39.2605048152353,7.35636314489289));
#64439=CARTESIAN_POINT('Ctrl Pts',(-16.3745211363523,39.2650853595413,7.29797512818008));
#64440=CARTESIAN_POINT('Ctrl Pts',(-16.3960846962851,39.2698332807662,7.23745356451644));
#64441=CARTESIAN_POINT('Ctrl Pts',(-16.4210707179747,39.2745812019911,7.17816551312208));
#64442=CARTESIAN_POINT('Ctrl Pts',(-16.4492993205381,39.279329123216,7.12051333200989));
#64443=CARTESIAN_POINT('Ctrl Pts',(-16.4765672953818,39.283915471273,7.0648230717245));
#64444=CARTESIAN_POINT('Ctrl Pts',(-16.5068603707055,39.28850181933,7.0106595512061));
#64445=CARTESIAN_POINT('Ctrl Pts',(-16.5399699736584,39.2930881673871,6.95835952325786));
#64446=CARTESIAN_POINT('Ctrl Pts',(-16.5748292116265,39.2979168751959,6.90329576660154));
#64447=CARTESIAN_POINT('Ctrl Pts',(-16.6128105375504,39.3027455830047,6.85029844399803));
#64448=CARTESIAN_POINT('Ctrl Pts',(-16.6536212425395,39.3075742908135,6.79972235968539));
#64449=CARTESIAN_POINT('Ctrl Pts',(-16.6944319475285,39.3124029986223,6.74914627537275));
#64450=CARTESIAN_POINT('Ctrl Pts',(-16.7380715376231,39.3172317064311,6.70099185881445));
#64451=CARTESIAN_POINT('Ctrl Pts',(-16.784203506772,39.3220604142399,6.65556779424143));
#64452=CARTESIAN_POINT('Ctrl Pts',(-16.8281229364164,39.326657531961,6.61232231729808));
#64453=CARTESIAN_POINT('Ctrl Pts',(-16.8744815298284,39.331254649682,6.5713735816584));
#64454=CARTESIAN_POINT('Ctrl Pts',(-16.9230094584221,39.3358517674031,6.53300866471959));
#64455=CARTESIAN_POINT('Ctrl Pts',(-16.9723796696096,39.340528675718,6.49397786109065));
#64456=CARTESIAN_POINT('Ctrl Pts',(-17.023994927625,39.3452055840328,6.457621864394));
#64457=CARTESIAN_POINT('Ctrl Pts',(-17.0775312116696,39.3498824923477,6.42420439837113));
#64458=CARTESIAN_POINT('Ctrl Pts',(-17.130009319699,39.35446695883,6.39144744813983));
#64459=CARTESIAN_POINT('Ctrl Pts',(-17.1843327517215,39.3590514253124,6.36151420496099));
#64460=CARTESIAN_POINT('Ctrl Pts',(-17.2401643630905,39.3636358917947,6.3346114283483));
#64461=CARTESIAN_POINT('Ctrl Pts',(-17.2959618337749,39.3682175549042,6.30772510261687));
#64462=CARTESIAN_POINT('Ctrl Pts',(-17.3532651974793,39.3727992180137,6.28386578953471));
#64463=CARTESIAN_POINT('Ctrl Pts',(-17.4117126387867,39.3773808811231,6.26319437681925));
#64464=CARTESIAN_POINT('Ctrl Pts',(-17.4701458102765,39.3819614256294,6.24252801098495));
#64465=CARTESIAN_POINT('Ctrl Pts',(-17.5297220251438,39.3865419701356,6.22504817011098));
#64466=CARTESIAN_POINT('Ctrl Pts',(-17.59006134055,39.3911225146419,6.21086688976854));
#64467=CARTESIAN_POINT('Ctrl Pts',(-17.6526054996454,39.3958704356684,6.19616741484173));
#64468=CARTESIAN_POINT('Ctrl Pts',(-17.7159690551745,39.4006183566949,6.18501242633746));
#64469=CARTESIAN_POINT('Ctrl Pts',(-17.7797163984031,39.4053662777214,6.17746896201831));
#64470=CARTESIAN_POINT('Ctrl Pts',(-17.8412944057669,39.4099526259694,6.17018220341996));
#64471=CARTESIAN_POINT('Ctrl Pts',(-17.9032299665162,39.4145389742174,6.16626506269091));
#64472=CARTESIAN_POINT('Ctrl Pts',(-17.9651270364674,39.4191253224654,6.16572489587046));
#64473=CARTESIAN_POINT('Ctrl Pts',(-18.0302949706326,39.4239540298812,6.1651561846888));
#64474=CARTESIAN_POINT('Ctrl Pts',(-18.0954195876102,39.4287827372969,6.16833122856295));
#64475=CARTESIAN_POINT('Ctrl Pts',(-18.1600440537407,39.4336114447127,6.17519647914202));
#64476=CARTESIAN_POINT('Ctrl Pts',(-18.2246685198713,39.4384401521284,6.18206172972109));
#64477=CARTESIAN_POINT('Ctrl Pts',(-18.2887922064639,39.4432688595442,6.19261700484584));
#64478=CARTESIAN_POINT('Ctrl Pts',(-18.3519732819213,39.4480975669599,6.20674694855633));
#64479=CARTESIAN_POINT('Ctrl Pts',(-18.4121241356718,39.4526946851866,6.22019920734551));
#64480=CARTESIAN_POINT('Ctrl Pts',(-18.4716678499828,39.4572918034133,6.23694629958069));
#64481=CARTESIAN_POINT('Ctrl Pts',(-18.5302169031767,39.46188892164,6.25691717662774));
#64482=CARTESIAN_POINT('Ctrl Pts',(-18.5897821648267,39.4665658298917,6.27723467882111));
#64483=CARTESIAN_POINT('Ctrl Pts',(-18.6483173698797,39.4712427381433,6.30088891746777));
#64484=CARTESIAN_POINT('Ctrl Pts',(-18.7054252334764,39.475919646395,6.32775064719233));
#64485=CARTESIAN_POINT('Ctrl Pts',(-18.7614043337383,39.4805041133921,6.35408144240603));
#64486=CARTESIAN_POINT('Ctrl Pts',(-18.8160115200929,39.4850885803892,6.38349386045697));
#64487=CARTESIAN_POINT('Ctrl Pts',(-18.8688902536374,39.4896730473864,6.41581674036991));
#64488=CARTESIAN_POINT('Ctrl Pts',(-18.9217366521901,39.4942547110126,6.44811985505796));
#64489=CARTESIAN_POINT('Ctrl Pts',(-18.9728562602278,39.4988363746388,6.48332963772018));
#64490=CARTESIAN_POINT('Ctrl Pts',(-19.0219177035941,39.503418038265,6.52122932470449));
#64491=CARTESIAN_POINT('Ctrl Pts',(-19.0709671687274,39.5079985832891,6.5591197585716));
#64492=CARTESIAN_POINT('Ctrl Pts',(-19.1179590640269,39.5125791283132,6.59969848197639));
#64493=CARTESIAN_POINT('Ctrl Pts',(-19.1625932323363,39.5171596733373,6.64270701035473));
#64494=CARTESIAN_POINT('Ctrl Pts',(-19.2088583564377,39.5219075938658,6.68728709279397));
#64495=CARTESIAN_POINT('Ctrl Pts',(-19.2525896491255,39.5266555143944,6.73447763243855));
#64496=CARTESIAN_POINT('Ctrl Pts',(-19.2934945768315,39.5314034349229,6.78394897346661));
#64497=CARTESIAN_POINT('Ctrl Pts',(-19.333007509586,39.5359897836855,6.83173680444298));
#64498=CARTESIAN_POINT('Ctrl Pts',(-19.3698831051157,39.5405761324481,6.88165222235139));
#64499=CARTESIAN_POINT('Ctrl Pts',(-19.4039004291453,39.5451624812107,6.93336645187149));
#64500=CARTESIAN_POINT('Ctrl Pts',(-19.439715339687,39.5499911876222,6.98781343019293));
#64501=CARTESIAN_POINT('Ctrl Pts',(-19.4723611869233,39.5548198940338,7.04425404942017));
#64502=CARTESIAN_POINT('Ctrl Pts',(-19.5016352469356,39.5596486004453,7.10227543292967));
#64503=CARTESIAN_POINT('Ctrl Pts',(-19.5309093069479,39.5644773068568,7.16029681643917));
#64504=CARTESIAN_POINT('Ctrl Pts',(-19.5568113918848,39.5693060132684,7.21989833721848));
#64505=CARTESIAN_POINT('Ctrl Pts',(-19.5791988445213,39.5741347196799,7.28064620873227));
#64506=CARTESIAN_POINT('Ctrl Pts',(-19.6037514026038,39.5794304135025,7.34726904733508));
#64507=CARTESIAN_POINT('Ctrl Pts',(-19.6241618666497,39.5847261073252,7.41549605425292));
#64508=CARTESIAN_POINT('Ctrl Pts',(-19.6402487498504,39.5900218011479,7.48483909307897));
#64509=CARTESIAN_POINT('Ctrl Pts',(-19.6561960370784,39.5952715409146,7.55358039887612));
#64510=CARTESIAN_POINT('Ctrl Pts',(-19.6678943533168,39.6005212806814,7.62341826524155));
#64511=CARTESIAN_POINT('Ctrl Pts',(-19.6752133150058,39.6057710204481,7.69385616040597));
#64512=CARTESIAN_POINT('Ctrl Pts',(-19.6812402070881,39.610093985423,7.7518591409785));
#64513=CARTESIAN_POINT('Ctrl Pts',(-19.6842982882008,39.6144169503979,7.81026856950894));
#64514=CARTESIAN_POINT('Ctrl Pts',(-19.6843395759433,39.6187399153728,7.86879772163009));
#64515=CARTESIAN_POINT('',(-19.6843395514373,40.4124899154864,7.8712365300618));
#64516=CARTESIAN_POINT('Ctrl Pts',(-19.6843395759439,39.6187399154298,7.86879772240173));
#64517=CARTESIAN_POINT('Ctrl Pts',(-19.6843834605849,39.623334787325,7.93100825561096));
#64518=CARTESIAN_POINT('Ctrl Pts',(-19.6810168737825,39.6279296592201,7.99324607275286));
#64519=CARTESIAN_POINT('Ctrl Pts',(-19.6742574015537,39.6325245311153,8.05511264916427));
#64520=CARTESIAN_POINT('Ctrl Pts',(-19.6674980385379,39.6371193287709,8.11697822599498));
#64521=CARTESIAN_POINT('Ctrl Pts',(-19.65734595536,39.6417141264265,8.17847207298165));
#64522=CARTESIAN_POINT('Ctrl Pts',(-19.6438705362152,39.6463089240822,8.23920140074895));
#64523=CARTESIAN_POINT('Ctrl Pts',(-19.6303798438661,39.6509089295375,8.29999955987628));
#64524=CARTESIAN_POINT('Ctrl Pts',(-19.6135584020532,39.6555089349927,8.36003097560791));
#64525=CARTESIAN_POINT('Ctrl Pts',(-19.5935264115865,39.660108940448,8.41891470622755));
#64526=CARTESIAN_POINT('Ctrl Pts',(-19.5734833716148,39.6647114832339,8.47783091669856));
#64527=CARTESIAN_POINT('Ctrl Pts',(-19.5502264444524,39.6693140260199,8.53559771268408));
#64528=CARTESIAN_POINT('Ctrl Pts',(-19.5239241603994,39.6739165688058,8.59185387893595));
#64529=CARTESIAN_POINT('Ctrl Pts',(-19.4975679111077,39.6785285547762,8.64822546776632));
#64530=CARTESIAN_POINT('Ctrl Pts',(-19.4681540596482,39.6831405407466,8.70307978841625));
#64531=CARTESIAN_POINT('Ctrl Pts',(-19.4358969845023,39.6877525267169,8.7560805866947));
#64532=CARTESIAN_POINT('Ctrl Pts',(-19.4069425912083,39.6918923086113,8.80365483052499));
#64533=CARTESIAN_POINT('Ctrl Pts',(-19.375698142922,39.6960320905056,8.84973584474876));
#64534=CARTESIAN_POINT('Ctrl Pts',(-19.3423463698601,39.7001718723999,8.8941031218237));
#64535=CARTESIAN_POINT('Ctrl Pts',(-19.3053101067791,39.7047689908515,8.94337181116394));
#64536=CARTESIAN_POINT('Ctrl Pts',(-19.2655216553048,39.709366109303,8.99073000183231));
#64537=CARTESIAN_POINT('Ctrl Pts',(-19.2232053905419,39.7139632277546,9.03585384698407));
#64538=CARTESIAN_POINT('Ctrl Pts',(-19.1801546645829,39.7186401359782,9.08176088303107));
#64539=CARTESIAN_POINT('Ctrl Pts',(-19.1344877834538,39.7233170442017,9.12535479199504));
#64540=CARTESIAN_POINT('Ctrl Pts',(-19.0864861736111,39.7279939524253,9.16632680416915));
#64541=CARTESIAN_POINT('Ctrl Pts',(-19.0394333355832,39.7325784196095,9.20648898745478));
#64542=CARTESIAN_POINT('Ctrl Pts',(-18.9901376285894,39.7371628867938,9.2441316298211));
#64543=CARTESIAN_POINT('Ctrl Pts',(-18.938901888341,39.741747353978,9.27900035632927));
#64544=CARTESIAN_POINT('Ctrl Pts',(-18.8876974785648,39.7463290177769,9.31384776073568));
#64545=CARTESIAN_POINT('Ctrl Pts',(-18.8345558078204,39.7509106815759,9.34592432684974));
#64546=CARTESIAN_POINT('Ctrl Pts',(-18.7798108992277,39.7554923453748,9.37501739560596));
#64547=CARTESIAN_POINT('Ctrl Pts',(-18.7250793566459,39.760072890557,9.40410336126743));
#64548=CARTESIAN_POINT('Ctrl Pts',(-18.6687458026009,39.7646534357393,9.43020703680343));
#64549=CARTESIAN_POINT('Ctrl Pts',(-18.6111694173609,39.7692339809215,9.45316139486417));
#64550=CARTESIAN_POINT('Ctrl Pts',(-18.5514891652782,39.7739819012714,9.47695451542484));
#64551=CARTESIAN_POINT('Ctrl Pts',(-18.4904740137347,39.7787298216212,9.49736343306464));
#64552=CARTESIAN_POINT('Ctrl Pts',(-18.4285448545843,39.7834777419711,9.51425738527334));
#64553=CARTESIAN_POINT('Ctrl Pts',(-18.3687231412914,39.7880640908543,9.53057643722366));
#64554=CARTESIAN_POINT('Ctrl Pts',(-18.3080491634902,39.7926504397375,9.54361588246976));
#64555=CARTESIAN_POINT('Ctrl Pts',(-18.2469135163627,39.7972367886208,9.55330983790355));
#64556=CARTESIAN_POINT('Ctrl Pts',(-18.1825472680243,39.8020654947039,9.56351605264325));
#64557=CARTESIAN_POINT('Ctrl Pts',(-18.1176698464845,39.8068942007871,9.57001332349494));
#64558=CARTESIAN_POINT('Ctrl Pts',(-18.0527409794033,39.8117229068703,9.57278700532846));
#64559=CARTESIAN_POINT('Ctrl Pts',(-17.9878121123222,39.8165516129535,9.57556068716197));
#64560=CARTESIAN_POINT('Ctrl Pts',(-17.9228324484238,39.8213803190367,9.57461086709453));
#64561=CARTESIAN_POINT('Ctrl Pts',(-17.8582560250215,39.8262090251199,9.5699862470492));
#64562=CARTESIAN_POINT('Ctrl Pts',(-17.7967766858213,39.8308061465389,9.56558342370503));
#64563=CARTESIAN_POINT('Ctrl Pts',(-17.7354102222827,39.8354032679579,9.55783219221645));
#64564=CARTESIAN_POINT('Ctrl Pts',(-17.6745504038976,39.840000389377,9.54674547258696));
#64565=CARTESIAN_POINT('Ctrl Pts',(-17.6126343184671,39.8446772972296,9.53546633475944));
#64566=CARTESIAN_POINT('Ctrl Pts',(-17.5512431682437,39.8493542050822,9.52073476806028));
#64567=CARTESIAN_POINT('Ctrl Pts',(-17.4907889895575,39.8540311129348,9.50261980352494));
#64568=CARTESIAN_POINT('Ctrl Pts',(-17.4315296688199,39.8586155831654,9.48486287560235));
#64569=CARTESIAN_POINT('Ctrl Pts',(-17.3731711301398,39.8632000533959,9.46385522942179));
#64570=CARTESIAN_POINT('Ctrl Pts',(-17.3160913162341,39.8677845236265,9.43971337995834));
#64571=CARTESIAN_POINT('Ctrl Pts',(-17.2590464061497,39.8723661904924,9.41558629303074));
#64572=CARTESIAN_POINT('Ctrl Pts',(-17.2032791382798,39.8769478573583,9.38832900092216));
#64573=CARTESIAN_POINT('Ctrl Pts',(-17.1491493160739,39.8815295242243,9.35810684314653));
#64574=CARTESIAN_POINT('Ctrl Pts',(-17.0950327095123,39.8861100724891,9.32789206402595));
#64575=CARTESIAN_POINT('Ctrl Pts',(-17.0425531992868,39.8906906207539,9.29471410426889));
#64576=CARTESIAN_POINT('Ctrl Pts',(-16.9920458895369,39.8952711690188,9.25878418453662));
#64577=CARTESIAN_POINT('Ctrl Pts',(-16.9396930878605,39.9000190864205,9.22154141767166));
#64578=CARTESIAN_POINT('Ctrl Pts',(-16.8894599130539,39.9047670038223,9.18134197493637));
#64579=CARTESIAN_POINT('Ctrl Pts',(-16.8416844604441,39.909514921224,9.13846859165122));
#64580=CARTESIAN_POINT('Ctrl Pts',(-16.7955347441432,39.9141012731923,9.09705413365267));
#64581=CARTESIAN_POINT('Ctrl Pts',(-16.7516784831589,39.9186876251606,9.05314522856172));
#64582=CARTESIAN_POINT('Ctrl Pts',(-16.7103828329202,39.9232739771288,9.00703433750092));
#64583=CARTESIAN_POINT('Ctrl Pts',(-16.6669050726911,39.9281026772473,8.95848689354746));
#64584=CARTESIAN_POINT('Ctrl Pts',(-16.6262664506392,39.9329313773658,8.90749879688026));
#64585=CARTESIAN_POINT('Ctrl Pts',(-16.5887285565003,39.9377600774844,8.85444837655531));
#64586=CARTESIAN_POINT('Ctrl Pts',(-16.5511906623615,39.9425887776029,8.80139795623036));
#64587=CARTESIAN_POINT('Ctrl Pts',(-16.5167537747039,39.9474174777214,8.74628580455052));
#64588=CARTESIAN_POINT('Ctrl Pts',(-16.4856231727145,39.9522461778399,8.68951981896229));
#64589=CARTESIAN_POINT('Ctrl Pts',(-16.45598565322,39.9568432843765,8.63547643730633));
#64590=CARTESIAN_POINT('Ctrl Pts',(-16.4292227170486,39.9614403909132,8.57971224002759));
#64591=CARTESIAN_POINT('Ctrl Pts',(-16.4055370287649,39.9660374974498,8.52256508319814));
#64592=CARTESIAN_POINT('Ctrl Pts',(-16.3814401702935,39.9707144071627,8.46442588396258));
#64593=CARTESIAN_POINT('Ctrl Pts',(-16.3605287557726,39.9753913168757,8.40485567186033));
#64594=CARTESIAN_POINT('Ctrl Pts',(-16.3429682111376,39.9800682265886,8.3442380814043));
#64595=CARTESIAN_POINT('Ctrl Pts',(-16.3257548079632,39.9846526819214,8.28481879540422));
#64596=CARTESIAN_POINT('Ctrl Pts',(-16.311761147436,39.9892371372542,8.22439367651532));
#64597=CARTESIAN_POINT('Ctrl Pts',(-16.3010942695617,39.993821592587,8.16334345723332));
#64598=CARTESIAN_POINT('Ctrl Pts',(-16.2904339143323,39.9984032445902,8.10233056929643));
#64599=CARTESIAN_POINT('Ctrl Pts',(-16.2830963955218,40.0029848965935,8.04069383933047));
#64600=CARTESIAN_POINT('Ctrl Pts',(-16.279137893869,40.0075665485967,7.97882523387381));
#64601=CARTESIAN_POINT('Ctrl Pts',(-16.2751803586257,40.0121470820576,7.91697173271963));
#64602=CARTESIAN_POINT('Ctrl Pts',(-16.2746002354141,40.0167276155185,7.85488697626326));
#64603=CARTESIAN_POINT('Ctrl Pts',(-16.2774017616269,40.0213081489793,7.7929670571187));
#64604=CARTESIAN_POINT('Ctrl Pts',(-16.2803056712924,40.0260560807777,7.72878423746007));
#64605=CARTESIAN_POINT('Ctrl Pts',(-16.2868432222247,40.0308040125761,7.66477912115993));
#64606=CARTESIAN_POINT('Ctrl Pts',(-16.2969601845755,40.0355519443745,7.60138910056386));
#64607=CARTESIAN_POINT('Ctrl Pts',(-16.3067328193948,40.0401382818543,7.54015653875443));
#64608=CARTESIAN_POINT('Ctrl Pts',(-16.3198449356221,40.0447246193342,7.47949837470028));
#64609=CARTESIAN_POINT('Ctrl Pts',(-16.336195665568,40.0493109568141,7.4197976613759));
#64610=CARTESIAN_POINT('Ctrl Pts',(-16.3534105442188,40.0541396857717,7.35694171924702));
#64611=CARTESIAN_POINT('Ctrl Pts',(-16.3742156630405,40.0589684147294,7.2951478547041));
#64612=CARTESIAN_POINT('Ctrl Pts',(-16.3984349834176,40.063797143687,7.23484101681334));
#64613=CARTESIAN_POINT('Ctrl Pts',(-16.4226543037948,40.0686258726446,7.17453417892257));
#64614=CARTESIAN_POINT('Ctrl Pts',(-16.4502874790932,40.0734546016022,7.115714922943));
#64615=CARTESIAN_POINT('Ctrl Pts',(-16.481103090757,40.0782833305598,7.0587769165872));
#64616=CARTESIAN_POINT('Ctrl Pts',(-16.5104406821505,40.082880457453,7.00456984831777));
#64617=CARTESIAN_POINT('Ctrl Pts',(-16.5427828906446,40.0874775843461,6.95184497186535));
#64618=CARTESIAN_POINT('Ctrl Pts',(-16.5779557347004,40.0920747112392,6.90095577307296));
#64619=CARTESIAN_POINT('Ctrl Pts',(-16.6137389815674,40.0967516184076,6.84918342391737));
#64620=CARTESIAN_POINT('Ctrl Pts',(-16.6524518797614,40.101428525576,6.79931158585618));
#64621=CARTESIAN_POINT('Ctrl Pts',(-16.6938617948253,40.1061054327443,6.75168727415355));
#64622=CARTESIAN_POINT('Ctrl Pts',(-16.7344533076658,40.1106899081552,6.70500418250723));
#64623=CARTESIAN_POINT('Ctrl Pts',(-16.7776358526656,40.1152743835661,6.66048099082597));
#64624=CARTESIAN_POINT('Ctrl Pts',(-16.8231475709803,40.119858858977,6.61841408881723));
#64625=CARTESIAN_POINT('Ctrl Pts',(-16.8686314580829,40.124440530901,6.57637291145511));
#64626=CARTESIAN_POINT('Ctrl Pts',(-16.9164413212043,40.129022202825,6.53678539022267));
#64627=CARTESIAN_POINT('Ctrl Pts',(-16.9662782841984,40.133603874749,6.49991127348911));
#64628=CARTESIAN_POINT('Ctrl Pts',(-17.0161030782439,40.1381844279424,6.46304616049905));
#64629=CARTESIAN_POINT('Ctrl Pts',(-17.0679535805295,40.1427649811359,6.42889343941496));
#64630=CARTESIAN_POINT('Ctrl Pts',(-17.1214992819713,40.1473455343294,6.39767145217373));
#64631=CARTESIAN_POINT('Ctrl Pts',(-17.1770013774115,40.152093446742,6.36530871027224));
#64632=CARTESIAN_POINT('Ctrl Pts',(-17.234324473639,40.1568413591545,6.33609535606809));
#64633=CARTESIAN_POINT('Ctrl Pts',(-17.2930716667694,40.161589271567,6.31022299651359));
#64634=CARTESIAN_POINT('Ctrl Pts',(-17.3498198855619,40.1661756280896,6.28523098851388));
#64635=CARTESIAN_POINT('Ctrl Pts',(-17.4078963179194,40.1707619846121,6.26335636640238));
#64636=CARTESIAN_POINT('Ctrl Pts',(-17.4669244179725,40.1753483411346,6.24472209061737));
#64637=CARTESIAN_POINT('Ctrl Pts',(-17.5290714438634,40.1801770314922,6.22510321725659));
#64638=CARTESIAN_POINT('Ctrl Pts',(-17.5922728715517,40.1850057218497,6.2090767825581));
#64639=CARTESIAN_POINT('Ctrl Pts',(-17.656076207819,40.1898344122073,6.1967253027494));
#64640=CARTESIAN_POINT('Ctrl Pts',(-17.7198795440864,40.1946631025648,6.18437382294069));
#64641=CARTESIAN_POINT('Ctrl Pts',(-17.7842841344778,40.1994917929224,6.17569730786789));
#64642=CARTESIAN_POINT('Ctrl Pts',(-17.8488337389117,40.2043204832799,6.17071478334209));
#64643=CARTESIAN_POINT('Ctrl Pts',(-17.9102880180637,40.2089176250869,6.16597118412448));
#64644=CARTESIAN_POINT('Ctrl Pts',(-17.9721261674394,40.213514766894,6.1645558626403));
#64645=CARTESIAN_POINT('Ctrl Pts',(-18.0339568376348,40.218111908701,6.16651431022375));
#64646=CARTESIAN_POINT('Ctrl Pts',(-18.0968603114741,40.2227888140051,6.16850673818777));
#64647=CARTESIAN_POINT('Ctrl Pts',(-18.1597555225077,40.2274657193092,6.17399126125987));
#64648=CARTESIAN_POINT('Ctrl Pts',(-18.2222247586303,40.2321426246133,6.18296058080836));
#64649=CARTESIAN_POINT('Ctrl Pts',(-18.2834596204156,40.2367271155989,6.19175266915376));
#64650=CARTESIAN_POINT('Ctrl Pts',(-18.3442846600452,40.2413116065845,6.20389301401672));
#64651=CARTESIAN_POINT('Ctrl Pts',(-18.4043088509711,40.2458960975701,6.21932231050772));
#64652=CARTESIAN_POINT('Ctrl Pts',(-18.4642963388076,40.2504777852695,6.23474217242174));
#64653=CARTESIAN_POINT('Ctrl Pts',(-18.523483456918,40.255059472969,6.25344687177774));
#64654=CARTESIAN_POINT('Ctrl Pts',(-18.581489893297,40.2596411606684,6.27532613244541));
#64655=CARTESIAN_POINT('Ctrl Pts',(-18.6394821681899,40.2642217298108,6.29720005158778));
#64656=CARTESIAN_POINT('Ctrl Pts',(-18.6962938574641,40.2688022989532,6.32224681392534));
#64657=CARTESIAN_POINT('Ctrl Pts',(-18.7515622869704,40.2733828680957,6.3503071123003));
#64658=CARTESIAN_POINT('Ctrl Pts',(-18.8088496721119,40.278130765421,6.37939245332686));
#64659=CARTESIAN_POINT('Ctrl Pts',(-18.8644783167017,40.2828786627463,6.41171555370701));
#64660=CARTESIAN_POINT('Ctrl Pts',(-18.9180720149298,40.2876265600717,6.44704682775378));
#64661=CARTESIAN_POINT('Ctrl Pts',(-18.9698424426039,40.2922129327836,6.48117612332669));
#64662=CARTESIAN_POINT('Ctrl Pts',(-19.0197137857215,40.2967993054956,6.51811181769598));
#64663=CARTESIAN_POINT('Ctrl Pts',(-19.0673785482589,40.3013856782075,6.5576042028464));
#64664=CARTESIAN_POINT('Ctrl Pts',(-19.1175613243197,40.3062143378396,6.5991828746914));
#64665=CARTESIAN_POINT('Ctrl Pts',(-19.1652974388243,40.3110429974716,6.64359542279421));
#64666=CARTESIAN_POINT('Ctrl Pts',(-19.2102722044345,40.3158716571037,6.69050640586911));
#64667=CARTESIAN_POINT('Ctrl Pts',(-19.2552469700448,40.3207003167357,6.73741738894401));
#64668=CARTESIAN_POINT('Ctrl Pts',(-19.2974600236317,40.3255289763678,6.78682626247607));
#64669=CARTESIAN_POINT('Ctrl Pts',(-19.336647989908,40.3303576359998,6.83836001091529));
#64670=CARTESIAN_POINT('Ctrl Pts',(-19.3740406321603,40.3349650795427,6.88753283620867));
#64671=CARTESIAN_POINT('Ctrl Pts',(-19.4088347701809,40.3395725230856,6.93884434070388));
#64672=CARTESIAN_POINT('Ctrl Pts',(-19.4407782109389,40.3441799666285,6.99198983260663));
#64673=CARTESIAN_POINT('Ctrl Pts',(-19.4726722376121,40.348780282805,7.04505311245642));
#64674=CARTESIAN_POINT('Ctrl Pts',(-19.5017240534172,40.3533805989816,7.09994432471515));
#64675=CARTESIAN_POINT('Ctrl Pts',(-19.527722958467,40.3579809151581,7.1563274704502));
#64676=CARTESIAN_POINT('Ctrl Pts',(-19.5536896928802,40.3625755389756,7.21264084856632));
#64677=CARTESIAN_POINT('Ctrl Pts',(-19.576610803041,40.3671701627932,7.27044203976666));
#64678=CARTESIAN_POINT('Ctrl Pts',(-19.5963210577965,40.3717647866107,7.32936974398072));
#64679=CARTESIAN_POINT('Ctrl Pts',(-19.6160164077617,40.376355935998,7.38825288737651));
#64680=CARTESIAN_POINT('Ctrl Pts',(-19.6325055595317,40.3809470853853,7.44826037554428));
#64681=CARTESIAN_POINT('Ctrl Pts',(-19.6456717694011,40.3855382347726,7.50901192232934));
#64682=CARTESIAN_POINT('Ctrl Pts',(-19.6588373065105,40.3901291495638,7.5697603648643));
#64683=CARTESIAN_POINT('Ctrl Pts',(-19.6686801137244,40.3947200643551,7.63125230042118));
#64684=CARTESIAN_POINT('Ctrl Pts',(-19.6751340377647,40.3993109791463,7.69309485702321));
#64685=CARTESIAN_POINT('Ctrl Pts',(-19.6813097026429,40.4037039579075,7.75227108878679));
#64686=CARTESIAN_POINT('Ctrl Pts',(-19.6843826970131,40.4080969366687,7.81176789347959));
#64687=CARTESIAN_POINT('Ctrl Pts',(-19.6843395514378,40.4124899154299,7.87123652929707));
#64688=CARTESIAN_POINT('Ctrl Pts',(-19.6843395514373,40.4124899154864,7.8712365300618));
#64689=CARTESIAN_POINT('Ctrl Pts',(-19.6842878411527,40.4177549291061,7.94251007690588));
#64690=CARTESIAN_POINT('Ctrl Pts',(-19.6797612505141,40.4230199427259,8.01360330873315));
#64691=CARTESIAN_POINT('Ctrl Pts',(-19.6708512413931,40.4282849563456,8.08400213802566));
#64692=CARTESIAN_POINT('Ctrl Pts',(-19.6618564270657,40.4336000822111,8.15507102131738));
#64693=CARTESIAN_POINT('Ctrl Pts',(-19.6483944695626,40.4389152080765,8.22543203500817));
#64694=CARTESIAN_POINT('Ctrl Pts',(-19.6306090111538,40.444230333942,8.29457593890581));
#64695=CARTESIAN_POINT('Ctrl Pts',(-19.6170407903194,40.4482851522013,8.34732463595239));
#64696=CARTESIAN_POINT('Ctrl Pts',(-19.6009573588429,40.4523399704605,8.3993653731387));
#64697=CARTESIAN_POINT('Ctrl Pts',(-19.5824409865512,40.4563947887198,8.45048059418118));
#64698=CARTESIAN_POINT('Ctrl Pts',(-19.5614477628561,40.4609920016846,8.50843326723516));
#64699=CARTESIAN_POINT('Ctrl Pts',(-19.5372635639648,40.4655892146493,8.5653646470191));
#64700=CARTESIAN_POINT('Ctrl Pts',(-19.5100081538699,40.4701864276141,8.62089938386691));
#64701=CARTESIAN_POINT('Ctrl Pts',(-19.4822803260345,40.4748633240235,8.67739670373251));
#64702=CARTESIAN_POINT('Ctrl Pts',(-19.4513738977614,40.4795402204329,8.73244797242256));
#64703=CARTESIAN_POINT('Ctrl Pts',(-19.417467586182,40.4842171168423,8.78567558353173));
#64704=CARTESIAN_POINT('Ctrl Pts',(-19.3842306907973,40.48880167675,8.83785231581559));
#64705=CARTESIAN_POINT('Ctrl Pts',(-19.3481115760661,40.4933862366577,8.88827629507691));
#64706=CARTESIAN_POINT('Ctrl Pts',(-19.3093253636047,40.4979707965654,8.93661563521128));
#64707=CARTESIAN_POINT('Ctrl Pts',(-19.2705628760136,40.5025525521753,8.98492540698873));
#64708=CARTESIAN_POINT('Ctrl Pts',(-19.2291368434709,40.5071343077852,9.03115267183257));
#64709=CARTESIAN_POINT('Ctrl Pts',(-19.18530441965,40.5117160633951,9.07499630355125));
#64710=CARTESIAN_POINT('Ctrl Pts',(-19.1414827074028,40.5162966993359,9.11882922095733));
#64711=CARTESIAN_POINT('Ctrl Pts',(-19.095256131015,40.5208773352767,9.16027930174823));
#64712=CARTESIAN_POINT('Ctrl Pts',(-19.0469192564903,40.5254579712174,9.1990816888853));
#64713=CARTESIAN_POINT('Ctrl Pts',(-18.9968180681141,40.5302058020693,9.23930037754727));
#64714=CARTESIAN_POINT('Ctrl Pts',(-18.9444499631566,40.5349536329212,9.27667393689923));
#64715=CARTESIAN_POINT('Ctrl Pts',(-18.8901790902337,40.5397014637731,9.310954148924));
#64716=CARTESIAN_POINT('Ctrl Pts',(-18.8377530679985,40.544287899782,9.34406906049716));
#64717=CARTESIAN_POINT('Ctrl Pts',(-18.7835520689903,40.5488743357909,9.37429737488332));
#64718=CARTESIAN_POINT('Ctrl Pts',(-18.727930304232,40.5534607717998,9.40146175127277));
#64719=CARTESIAN_POINT('Ctrl Pts',(-18.6693725780964,40.5582893000732,9.43005998292126));
#64720=CARTESIAN_POINT('Ctrl Pts',(-18.6092405334155,40.5631178283465,9.4552615992809));
#64721=CARTESIAN_POINT('Ctrl Pts',(-18.5479694136963,40.5679463566199,9.47691803795511));
#64722=CARTESIAN_POINT('Ctrl Pts',(-18.486698293977,40.5727748848932,9.49857447662932));
#64723=CARTESIAN_POINT('Ctrl Pts',(-18.4242887448175,40.5776034131666,9.51668563102563));
#64724=CARTESIAN_POINT('Ctrl Pts',(-18.361189111174,40.5824319414399,9.53116516250563));
#64725=CARTESIAN_POINT('Ctrl Pts',(-18.301111690253,40.587029203084,9.54495118402799));
#64726=CARTESIAN_POINT('Ctrl Pts',(-18.2401621044606,40.5916264647281,9.55550217781377));
#64727=CARTESIAN_POINT('Ctrl Pts',(-18.1787206854397,40.5962237263722,9.56271525212553));
#64728=CARTESIAN_POINT('Ctrl Pts',(-18.1162150461293,40.6009006166967,9.5700532633309));
#64729=CARTESIAN_POINT('Ctrl Pts',(-18.0532008692111,40.6055775070212,9.57393641178694));
#64730=CARTESIAN_POINT('Ctrl Pts',(-17.9900923324682,40.6102543973457,9.57431011861848));
#64731=CARTESIAN_POINT('Ctrl Pts',(-17.9282289445468,40.6148390113352,9.57467645211125));
#64732=CARTESIAN_POINT('Ctrl Pts',(-17.8662754201515,40.6194236253247,9.571670567226));
#64733=CARTESIAN_POINT('Ctrl Pts',(-17.8046272750187,40.6240082393142,9.56529326163134));
#64734=CARTESIAN_POINT('Ctrl Pts',(-17.7430168138054,40.6285900508475,9.55891985431895));
#64735=CARTESIAN_POINT('Ctrl Pts',(-17.6817118669993,40.6331718623809,9.5491791649594));
#64736=CARTESIAN_POINT('Ctrl Pts',(-17.6211048950814,40.6377536739142,9.53612398676252));
#64737=CARTESIAN_POINT('Ctrl Pts',(-17.5605127109042,40.6423343675128,9.52307199395149));
#64738=CARTESIAN_POINT('Ctrl Pts',(-17.5006186609421,40.6469150611114,9.50670722486737));
#64739=CARTESIAN_POINT('Ctrl Pts',(-17.4418050166596,40.6514957547099,9.48713357379878));
#64740=CARTESIAN_POINT('Ctrl Pts',(-17.3808460947574,40.6562435329974,9.46684595718556));
#64741=CARTESIAN_POINT('Ctrl Pts',(-17.3210484916843,40.6609913112849,9.44311096440126));
#64742=CARTESIAN_POINT('Ctrl Pts',(-17.2628181995382,40.6657390895724,9.4160999646486));
#64743=CARTESIAN_POINT('Ctrl Pts',(-17.2065659782525,40.6703255868232,9.39000652291512));
#64744=CARTESIAN_POINT('Ctrl Pts',(-17.1517767189282,40.6749120840741,9.36085640068078));
#64745=CARTESIAN_POINT('Ctrl Pts',(-17.0987915006898,40.6794985813249,9.3288510603703));
#64746=CARTESIAN_POINT('Ctrl Pts',(-17.0430114990502,40.6843270001307,9.29515755123035));
#64747=CARTESIAN_POINT('Ctrl Pts',(-16.9892316597327,40.6891554189365,9.25829963538069));
#64748=CARTESIAN_POINT('Ctrl Pts',(-16.9378127825556,40.6939838377423,9.21856243437058));
#64749=CARTESIAN_POINT('Ctrl Pts',(-16.8863939053786,40.6988122565482,9.17882523336047));
#64750=CARTESIAN_POINT('Ctrl Pts',(-16.8373364298726,40.703640675354,9.1362092317421));
#64751=CARTESIAN_POINT('Ctrl Pts',(-16.7909559844104,40.7084690941598,9.09104429264079));
#64752=CARTESIAN_POINT('Ctrl Pts',(-16.7468039473542,40.7130655253478,9.04804936137239));
#64753=CARTESIAN_POINT('Ctrl Pts',(-16.7048960713131,40.7176619565358,9.00256812221833));
#64754=CARTESIAN_POINT('Ctrl Pts',(-16.665525008342,40.7222583877239,8.95486419975304));
#64755=CARTESIAN_POINT('Ctrl Pts',(-16.6254638776663,40.7269353818554,8.90632415720873));
#64756=CARTESIAN_POINT('Ctrl Pts',(-16.5880297897841,40.7316123759869,8.85548306815653));
#64757=CARTESIAN_POINT('Ctrl Pts',(-16.5534933249741,40.7362893701184,8.80265939211831));
#64758=CARTESIAN_POINT('Ctrl Pts',(-16.5196451881018,40.7408731495638,8.75088851671246));
#64759=CARTESIAN_POINT('Ctrl Pts',(-16.4885805250383,40.7454569290092,8.69721380371065));
#64760=CARTESIAN_POINT('Ctrl Pts',(-16.4605131055109,40.7500407084546,8.64196788344839));
#64761=CARTESIAN_POINT('Ctrl Pts',(-16.4324628412779,40.7546216862144,8.58675573045232));
#64762=CARTESIAN_POINT('Ctrl Pts',(-16.4074064182867,40.7592026639742,8.529974727469));
#64763=CARTESIAN_POINT('Ctrl Pts',(-16.3855122645559,40.763783641734,8.47198313690539));
#64764=CARTESIAN_POINT('Ctrl Pts',(-16.3636234437673,40.7683635036668,8.41400567183841));
#64765=CARTESIAN_POINT('Ctrl Pts',(-16.344895542964,40.7729433655995,8.35481868075846));
#64766=CARTESIAN_POINT('Ctrl Pts',(-16.3294485300274,40.7775232275322,8.29479957694341));
#64767=CARTESIAN_POINT('Ctrl Pts',(-16.3134324461011,40.7822718124779,8.23256935755861));
#64768=CARTESIAN_POINT('Ctrl Pts',(-16.3009439111735,40.7870203974235,8.16944506758937));
#64769=CARTESIAN_POINT('Ctrl Pts',(-16.2920591288017,40.7917689823691,8.1058610839843));
#64770=CARTESIAN_POINT('Ctrl Pts',(-16.2834791470357,40.7963546627542,8.04445840723785));
#64771=CARTESIAN_POINT('Ctrl Pts',(-16.2782596213027,40.8009403431392,7.98262760078482));
#64772=CARTESIAN_POINT('Ctrl Pts',(-16.2764161851709,40.8055260235242,7.9207643718782));
#64773=CARTESIAN_POINT('Ctrl Pts',(-16.2744745179824,40.8103560607502,7.85560464127183));
#64774=CARTESIAN_POINT('Ctrl Pts',(-16.2762787961322,40.8151860979761,7.79040958364245));
#64775=CARTESIAN_POINT('Ctrl Pts',(-16.281784964333,40.820016135202,7.72563751098501));
#64776=CARTESIAN_POINT('Ctrl Pts',(-16.2872911325338,40.824846172428,7.66086543832757));
#64777=CARTESIAN_POINT('Ctrl Pts',(-16.2964990212439,40.8296762096539,7.59651698449358));
#64778=CARTESIAN_POINT('Ctrl Pts',(-16.3093023662471,40.8345062468799,7.53303671984536));
#64779=CARTESIAN_POINT('Ctrl Pts',(-16.3214907112066,40.8391042765246,7.47260568690377));
#64780=CARTESIAN_POINT('Ctrl Pts',(-16.3369870654642,40.8437023061694,7.412712884101));
#64781=CARTESIAN_POINT('Ctrl Pts',(-16.3557284589915,40.8483003358141,7.35374735190046));
#64782=CARTESIAN_POINT('Ctrl Pts',(-16.37479089435,40.8529771301385,7.29377173459539));
#64783=CARTESIAN_POINT('Ctrl Pts',(-16.3972105797347,40.8576539244629,7.23475599390204));
#64784=CARTESIAN_POINT('Ctrl Pts',(-16.4228666501253,40.8623307187874,7.17709988720741));
#64785=CARTESIAN_POINT('Ctrl Pts',(-16.4480211573433,40.8669160841531,7.12057092817619));
#64786=CARTESIAN_POINT('Ctrl Pts',(-16.4762864321406,40.8715014495189,7.06534940841457));
#64787=CARTESIAN_POINT('Ctrl Pts',(-16.5074987781142,40.8760868148846,7.01179548641081));
#64788=CARTESIAN_POINT('Ctrl Pts',(-16.5386919922201,40.8806693696124,6.95827439073013));
#64789=CARTESIAN_POINT('Ctrl Pts',(-16.5728284398669,40.8852519243403,6.90641930469754));
#64790=CARTESIAN_POINT('Ctrl Pts',(-16.6096983038783,40.8898344790681,6.85656618508852));
#64791=CARTESIAN_POINT('Ctrl Pts',(-16.6465590984013,40.8944159065493,6.80672532867346));
#64792=CARTESIAN_POINT('Ctrl Pts',(-16.6861516720603,40.8989973340306,6.75888587002064));
#64793=CARTESIAN_POINT('Ctrl Pts',(-16.728223839013,40.9035787615118,6.7133534341102));
#64794=CARTESIAN_POINT('Ctrl Pts',(-16.7718169799035,40.9083258146859,6.66617493018474));
#64795=CARTESIAN_POINT('Ctrl Pts',(-16.8180720839233,40.9130728678599,6.62147392010099));
#64796=CARTESIAN_POINT('Ctrl Pts',(-16.8666660075634,40.9178199210339,6.57954959146613));
#64797=CARTESIAN_POINT('Ctrl Pts',(-16.9136235679298,40.9224071208169,6.53903703258589));
#64798=CARTESIAN_POINT('Ctrl Pts',(-16.9627644637704,40.9269943206,6.50111737585054));
#64799=CARTESIAN_POINT('Ctrl Pts',(-17.0137645727833,40.9315815203831,6.46601854186343));
#64800=CARTESIAN_POINT('Ctrl Pts',(-17.0674305370288,40.9364085002526,6.42908503708725));
#64801=CARTESIAN_POINT('Ctrl Pts',(-17.1231548723184,40.941235480122,6.39527568975556));
#64802=CARTESIAN_POINT('Ctrl Pts',(-17.1805296351771,40.9460624599915,6.36480168370747));
#64803=CARTESIAN_POINT('Ctrl Pts',(-17.2379043980357,40.950889439861,6.33432767765938));
#64804=CARTESIAN_POINT('Ctrl Pts',(-17.2969289675865,40.9557164197304,6.30718921361192));
#64805=CARTESIAN_POINT('Ctrl Pts',(-17.3571732524428,40.9605433995999,6.28353799978463));
#64806=CARTESIAN_POINT('Ctrl Pts',(-17.4145580294188,40.9651412658363,6.26100939588588));
#64807=CARTESIAN_POINT('Ctrl Pts',(-17.4732841783451,40.9697391320727,6.24155223822962));
#64808=CARTESIAN_POINT('Ctrl Pts',(-17.5329906431261,40.9743369983091,6.2253245090696));
#64809=CARTESIAN_POINT('Ctrl Pts',(-17.5937223088222,40.9790138130595,6.20881813867956));
#64810=CARTESIAN_POINT('Ctrl Pts',(-17.6554678145706,40.98369062781,6.19565342837095));
#64811=CARTESIAN_POINT('Ctrl Pts',(-17.7178256722736,40.9883674425604,6.18594553013236));
#64812=CARTESIAN_POINT('Ctrl Pts',(-17.7789625958245,40.9929526877307,6.17642770745023));
#64813=CARTESIAN_POINT('Ctrl Pts',(-17.840687581427,40.9975379329009,6.17023263360172));
#64814=CARTESIAN_POINT('Ctrl Pts',(-17.9026092417226,41.0021231780712,6.16741798842662));
#64815=CARTESIAN_POINT('Ctrl Pts',(-17.9644931649934,41.0067056288476,6.16460505858562));
#64816=CARTESIAN_POINT('Ctrl Pts',(-18.0265730179909,41.0112880796239,6.16516849546682));
#64817=CARTESIAN_POINT('Ctrl Pts',(-18.0884527516576,41.0158705304003,6.16911410251661));
#64818=CARTESIAN_POINT('Ctrl Pts',(-18.1503174830268,41.0204518701943,6.17305875298227));
#64819=CARTESIAN_POINT('Ctrl Pts',(-18.2119816837657,41.0250332099883,6.18038391343445));
#64820=CARTESIAN_POINT('Ctrl Pts',(-18.2730518285094,41.0296145497823,6.19104334141489));
#64821=CARTESIAN_POINT('Ctrl Pts',(-18.3363324803282,41.0343617166605,6.20208860016527));
#64822=CARTESIAN_POINT('Ctrl Pts',(-18.3989746623878,41.0391088835386,6.21671409507796));
#64823=CARTESIAN_POINT('Ctrl Pts',(-18.4605517470838,41.0438560504167,6.23481045319672));
#64824=CARTESIAN_POINT('Ctrl Pts',(-18.520053238235,41.0484432034037,6.25229683303733));
#64825=CARTESIAN_POINT('Ctrl Pts',(-18.5785598237685,41.0530303563906,6.27302355336963));
#64826=CARTESIAN_POINT('Ctrl Pts',(-18.6357042839605,41.0576175093776,6.29684179829368));
#64827=CARTESIAN_POINT('Ctrl Pts',(-18.6958388038233,41.0624446832013,6.32190632279299));
#64828=CARTESIAN_POINT('Ctrl Pts',(-18.7544641529891,41.067271857025,6.35039451360709));
#64829=CARTESIAN_POINT('Ctrl Pts',(-18.8111816878708,41.0720990308487,6.38207801368881));
#64830=CARTESIAN_POINT('Ctrl Pts',(-18.8678992227526,41.0769262046724,6.41376151377053));
#64831=CARTESIAN_POINT('Ctrl Pts',(-18.9227084380972,41.0817533784961,6.44863990994636));
#64832=CARTESIAN_POINT('Ctrl Pts',(-18.9752486778418,41.0865805523198,6.48643398970117));
#64833=CARTESIAN_POINT('Ctrl Pts',(-19.0248466829921,41.0911374061395,6.52211161453584));
#64834=CARTESIAN_POINT('Ctrl Pts',(-19.0726347189551,41.0956942599593,6.56053956304578));
#64835=CARTESIAN_POINT('Ctrl Pts',(-19.1182874020377,41.100251113779,6.60150615848472));
#64836=CARTESIAN_POINT('Ctrl Pts',(-19.1638599640665,41.1047999702609,6.64240085701476));
#64837=CARTESIAN_POINT('Ctrl Pts',(-19.2073042273338,41.1093488267428,6.68582501751963));
#64838=CARTESIAN_POINT('Ctrl Pts',(-19.2483254139918,41.1138976832247,6.73152493227887));
#64839=CARTESIAN_POINT('Ctrl Pts',(-19.2893065428958,41.1184420976855,6.77718022044173));
#64840=CARTESIAN_POINT('Ctrl Pts',(-19.3278689372972,41.1229865121464,6.82510647678214));
#64841=CARTESIAN_POINT('Ctrl Pts',(-19.3637537214592,41.1275309266073,6.87501232472565));
#64842=CARTESIAN_POINT('Ctrl Pts',(-19.399617222011,41.1320726457323,6.92488857303136));
#64843=CARTESIAN_POINT('Ctrl Pts',(-19.4328059574439,41.1366143648573,6.97674166550847));
#64844=CARTESIAN_POINT('Ctrl Pts',(-19.4631019211595,41.1411560839822,7.03024793715464));
#64845=CARTESIAN_POINT('Ctrl Pts',(-19.4933915305055,41.145696850513,7.0837429862291));
#64846=CARTESIAN_POINT('Ctrl Pts',(-19.5207893171996,41.1502376170437,7.13889007462835));
#64847=CARTESIAN_POINT('Ctrl Pts',(-19.5451222840827,41.1547783835744,7.19533929159332));
#64848=CARTESIAN_POINT('Ctrl Pts',(-19.5694763472953,41.1593230868838,7.25183744921097));
#64849=CARTESIAN_POINT('Ctrl Pts',(-19.5907600761388,41.1638677901933,7.30963951323497));
#64850=CARTESIAN_POINT('Ctrl Pts',(-19.6088484657843,41.1684124935028,7.36837512909319));
#64851=CARTESIAN_POINT('Ctrl Pts',(-19.6269446131302,41.1729591459325,7.42713593532626));
#64852=CARTESIAN_POINT('Ctrl Pts',(-19.6418425658306,41.1775057983622,7.48683058660605));
#64853=CARTESIAN_POINT('Ctrl Pts',(-19.6534679622412,41.182052450792,7.54707614682026));
#64854=CARTESIAN_POINT('Ctrl Pts',(-19.6651144382153,41.1866073473663,7.60743094633072));
#64855=CARTESIAN_POINT('Ctrl Pts',(-19.6734764366779,41.1911622439407,7.66833813464));
#64856=CARTESIAN_POINT('Ctrl Pts',(-19.6785313660541,41.1957171405151,7.72940827147221));
#64857=CARTESIAN_POINT('Ctrl Pts',(-19.6824240182035,41.1992247321392,7.77643658417713));
#64858=CARTESIAN_POINT('Ctrl Pts',(-19.6843566180351,41.2027323237633,7.82356137122071));
#64859=CARTESIAN_POINT('Ctrl Pts',(-19.6843398922845,41.2062399153875,7.87060594373627));
#64860=CARTESIAN_POINT('Origin',(-17.98,42.93984859951,7.87));
#64861=CARTESIAN_POINT('',(-19.24999991436,34.6054735995751,7.87046639652064));
#64862=CARTESIAN_POINT('Ctrl Pts',(-18.810359785549,34.7139132859163,8.83093840933901));
#64863=CARTESIAN_POINT('Ctrl Pts',(-18.8480000770215,34.7089793142232,8.79841292794362));
#64864=CARTESIAN_POINT('Ctrl Pts',(-18.8837142939927,34.7040453425301,8.76368311649533));
#64865=CARTESIAN_POINT('Ctrl Pts',(-18.9172453719093,34.699111370837,8.72701290120657));
#64866=CARTESIAN_POINT('Ctrl Pts',(-18.9507928644184,34.6941749837985,8.69032473461191));
#64867=CARTESIAN_POINT('Ctrl Pts',(-18.9821547422459,34.68923859676,8.65169469762151));
#64868=CARTESIAN_POINT('Ctrl Pts',(-19.0111143192575,34.6843022097216,8.61141976006991));
#64869=CARTESIAN_POINT('Ctrl Pts',(-19.0401293155334,34.6793563760348,8.57106774931358));
#64870=CARTESIAN_POINT('Ctrl Pts',(-19.0667325374929,34.674410542348,8.52906501637736));
#64871=CARTESIAN_POINT('Ctrl Pts',(-19.0907515469335,34.6694647086613,8.48573614558909));
#64872=CARTESIAN_POINT('Ctrl Pts',(-19.1060831698011,34.6663077234809,8.4580788057703));
#64873=CARTESIAN_POINT('Ctrl Pts',(-19.1203628104226,34.6631507383005,8.4298816437122));
#64874=CARTESIAN_POINT('Ctrl Pts',(-19.1335559487169,34.6599937531201,8.40123316272596));
#64875=CARTESIAN_POINT('Ctrl Pts',(-19.1560538394946,34.65461023434,8.35237970710382));
#64876=CARTESIAN_POINT('Ctrl Pts',(-19.1754766558247,34.64922671556,8.30202519731203));
#64877=CARTESIAN_POINT('Ctrl Pts',(-19.1916417683459,34.6438431967799,8.25055778168331));
#64878=CARTESIAN_POINT('Ctrl Pts',(-19.2077585403069,34.6384757770101,8.19924427551205));
#64879=CARTESIAN_POINT('Ctrl Pts',(-19.22063686448,34.6331083572404,8.14682484893595));
#64880=CARTESIAN_POINT('Ctrl Pts',(-19.2301420171886,34.6277409374706,8.09370725705597));
#64881=CARTESIAN_POINT('Ctrl Pts',(-19.2396044484566,34.6223976418693,8.04082840516496));
#64882=CARTESIAN_POINT('Ctrl Pts',(-19.2457238109817,34.6170543462681,7.9872580131992));
#64883=CARTESIAN_POINT('Ctrl Pts',(-19.2484157084143,34.6117110506668,7.93341601255157));
#64884=CARTESIAN_POINT('Ctrl Pts',(-19.2494631630086,34.6096319003029,7.91246534397657));
#64885=CARTESIAN_POINT('Ctrl Pts',(-19.2499921996046,34.607552749939,7.89147371151049));
#64886=CARTESIAN_POINT('Ctrl Pts',(-19.24999991436,34.6054735995751,7.87046639652063));
#64887=CARTESIAN_POINT('',(-17.7961609204192,34.0285,9.12662372762052));
#64888=CARTESIAN_POINT('Ctrl Pts',(-19.2499999143602,34.60547359951,7.87046639586325));
#64889=CARTESIAN_POINT('Ctrl Pts',(-19.2500186228147,34.600431606206,7.81952311472636));
#64890=CARTESIAN_POINT('Ctrl Pts',(-19.246967776457,34.5953896129021,7.76860069349798));
#64891=CARTESIAN_POINT('Ctrl Pts',(-19.2408810348543,34.5903476195981,7.71808220662215));
#64892=CARTESIAN_POINT('Ctrl Pts',(-19.2347835878813,34.5852967584287,7.66747486775573));
#64893=CARTESIAN_POINT('Ctrl Pts',(-19.2256396491361,34.5802458972594,7.6172733915475));
#64894=CARTESIAN_POINT('Ctrl Pts',(-19.2135345173812,34.57519503609,7.56785335608491));
#64895=CARTESIAN_POINT('Ctrl Pts',(-19.2014184031309,34.5701395924791,7.51838848382752));
#64896=CARTESIAN_POINT('Ctrl Pts',(-19.1863358983142,34.5650841488681,7.4697069540304));
#64897=CARTESIAN_POINT('Ctrl Pts',(-19.168422001748,34.5600287052572,7.42216839575436));
#64898=CARTESIAN_POINT('Ctrl Pts',(-19.1504644036985,34.5549609287412,7.37451386575195));
#64899=CARTESIAN_POINT('Ctrl Pts',(-19.129661823782,34.5498931522253,7.32800834707118));
#64900=CARTESIAN_POINT('Ctrl Pts',(-19.1061968005565,34.5448253757093,7.28298997758443));
#64901=CARTESIAN_POINT('Ctrl Pts',(-19.0894217866189,34.5412024506063,7.25080659688501));
#64902=CARTESIAN_POINT('Ctrl Pts',(-19.0712870579479,34.5375795255032,7.21938276448517));
#64903=CARTESIAN_POINT('Ctrl Pts',(-19.051872661738,34.5339566004002,7.18883262187727));
#64904=CARTESIAN_POINT('Ctrl Pts',(-19.0253535487371,34.5290078624037,7.14710262547379));
#64905=CARTESIAN_POINT('Ctrl Pts',(-18.9963354076115,34.5240591244073,7.10683163003986));
#64906=CARTESIAN_POINT('Ctrl Pts',(-18.9650042712288,34.5191103864108,7.06833511636029));
#64907=CARTESIAN_POINT('Ctrl Pts',(-18.9337306655237,34.5141707353574,7.02990929052597));
#64908=CARTESIAN_POINT('Ctrl Pts',(-18.9001528311632,34.5092310843039,6.99325190543645));
#64909=CARTESIAN_POINT('Ctrl Pts',(-18.8644999814156,34.5042914332505,6.95864947310278));
#64910=CARTESIAN_POINT('Ctrl Pts',(-18.828883254654,34.4993567869848,6.92408209948645));
#64911=CARTESIAN_POINT('Ctrl Pts',(-18.7911960657585,34.4944221407191,6.89156593650389));
#64912=CARTESIAN_POINT('Ctrl Pts',(-18.7517063628538,34.4894874944534,6.86135274276335));
#64913=CARTESIAN_POINT('Ctrl Pts',(-18.7122398805274,34.4845557498389,6.83115731486508));
#64914=CARTESIAN_POINT('Ctrl Pts',(-18.6709734181886,34.4796240052243,6.8032625057152));
#64915=CARTESIAN_POINT('Ctrl Pts',(-18.6282081130353,34.4746922606097,6.77787993233562));
#64916=CARTESIAN_POINT('Ctrl Pts',(-18.5854497731739,34.4697613192407,6.75250149307909));
#64917=CARTESIAN_POINT('Ctrl Pts',(-18.5411935464605,34.4648303778717,6.72963475584668));
#64918=CARTESIAN_POINT('Ctrl Pts',(-18.4957674568792,34.4598994365027,6.70944671366438));
#64919=CARTESIAN_POINT('Ctrl Pts',(-18.4502969249553,34.4549636709767,6.68923892063199));
#64920=CARTESIAN_POINT('Ctrl Pts',(-18.4036547469488,34.4500279054508,6.67171527708261));
#64921=CARTESIAN_POINT('Ctrl Pts',(-18.3561896772165,34.4450921399248,6.65699491890769));
#64922=CARTESIAN_POINT('Ctrl Pts',(-18.3086990327265,34.4401537149483,6.64226662922451));
#64923=CARTESIAN_POINT('Ctrl Pts',(-18.2603851459658,34.4352152899717,6.6303447640693));
#64924=CARTESIAN_POINT('Ctrl Pts',(-18.2116092631565,34.4302768649952,6.62129781404046));
#64925=CARTESIAN_POINT('Ctrl Pts',(-18.1627422776133,34.4253292161156,6.61223396627789));
#64926=CARTESIAN_POINT('Ctrl Pts',(-18.1134121175931,34.4203815672359,6.60605581906447));
#64927=CARTESIAN_POINT('Ctrl Pts',(-18.0639858589226,34.4154339183563,6.60278006032851));
#64928=CARTESIAN_POINT('Ctrl Pts',(-18.0389630531116,34.4129290947976,6.60112165694256));
#64929=CARTESIAN_POINT('Ctrl Pts',(-18.013915625472,34.4104242712389,6.60020631664651));
#64930=CARTESIAN_POINT('Ctrl Pts',(-17.9888908928602,34.4079194476802,6.60003112163166));
#64931=CARTESIAN_POINT('Ctrl Pts',(-17.9395139360616,34.4029771145666,6.5996854397491));
#64932=CARTESIAN_POINT('Ctrl Pts',(-17.890006080321,34.398034781453,6.60222299368832));
#64933=CARTESIAN_POINT('Ctrl Pts',(-17.8407324357409,34.3930924483394,6.60765910089812));
#64934=CARTESIAN_POINT('Ctrl Pts',(-17.7915496724127,34.3881592309595,6.61308518164788));
#64935=CARTESIAN_POINT('Ctrl Pts',(-17.7426008050934,34.3832260135796,6.62139915367661));
#64936=CARTESIAN_POINT('Ctrl Pts',(-17.6942501103006,34.3782927961996,6.63256434489031));
#64937=CARTESIAN_POINT('Ctrl Pts',(-17.6459485910255,34.3733645961937,6.64371818044383));
#64938=CARTESIAN_POINT('Ctrl Pts',(-17.5982445727108,34.3684363961878,6.65771737207312));
#64939=CARTESIAN_POINT('Ctrl Pts',(-17.551494205748,34.3635081961818,6.67447384625325));
#64940=CARTESIAN_POINT('Ctrl Pts',(-17.5047713711017,34.358582898501,6.69122045217825));
#64941=CARTESIAN_POINT('Ctrl Pts',(-17.4590015915058,34.3536576008201,6.71072093911075));
#64942=CARTESIAN_POINT('Ctrl Pts',(-17.4145253338303,34.3487323031392,6.73283756572764));
#64943=CARTESIAN_POINT('Ctrl Pts',(-17.3700562283285,34.3438077974896,6.75495063579629));
#64944=CARTESIAN_POINT('Ctrl Pts',(-17.3268807230226,34.3388832918399,6.77967876502301));
#64945=CARTESIAN_POINT('Ctrl Pts',(-17.2853163954858,34.3339587861903,6.80683741148444));
#64946=CARTESIAN_POINT('Ctrl Pts',(-17.2437107803969,34.3290293888271,6.83402303574376));
#64947=CARTESIAN_POINT('Ctrl Pts',(-17.2037199986934,34.324099991464,6.86364369561324));
#64948=CARTESIAN_POINT('Ctrl Pts',(-17.1656326711676,34.3191705941008,6.89547147105363));
#64949=CARTESIAN_POINT('Ctrl Pts',(-17.1275245720404,34.3142385084031,6.92731660433739));
#64950=CARTESIAN_POINT('Ctrl Pts',(-17.0913223943485,34.3093064227055,6.9613708728251));
#64951=CARTESIAN_POINT('Ctrl Pts',(-17.0572789666622,34.3043743370078,6.99736840841281));
#64952=CARTESIAN_POINT('Ctrl Pts',(-17.02317104724,34.2994329079863,7.03343413759067));
#64953=CARTESIAN_POINT('Ctrl Pts',(-16.9912303931655,34.2944914789648,7.07145006012652));
#64954=CARTESIAN_POINT('Ctrl Pts',(-16.9616694537387,34.2895500499434,7.11111733545216));
#64955=CARTESIAN_POINT('Ctrl Pts',(-16.9463792721866,34.2869941316156,7.13163494596014));
#64956=CARTESIAN_POINT('Ctrl Pts',(-16.9317250454833,34.2844382132879,7.15259388680391));
#64957=CARTESIAN_POINT('Ctrl Pts',(-16.9177313970105,34.2818822949602,7.17395013461477));
#64958=CARTESIAN_POINT('Ctrl Pts',(-16.8905925241095,34.276925421649,7.21536781750925));
#64959=CARTESIAN_POINT('Ctrl Pts',(-16.8658205031715,34.2719685483378,7.25846521105024));
#64960=CARTESIAN_POINT('Ctrl Pts',(-16.8436263679747,34.2670116750265,7.30294182975858));
#64961=CARTESIAN_POINT('Ctrl Pts',(-16.8214733055949,34.2620639749833,7.34733613933392));
#64962=CARTESIAN_POINT('Ctrl Pts',(-16.8018889075183,34.2571162749401,7.39310412652142));
#64963=CARTESIAN_POINT('Ctrl Pts',(-16.7850399872838,34.252168574897,7.43991795200291));
#64964=CARTESIAN_POINT('Ctrl Pts',(-16.7682083159663,34.2472259400132,7.48668385228935));
#64965=CARTESIAN_POINT('Ctrl Pts',(-16.7541067617319,34.2422833051294,7.53449295983615));
#64966=CARTESIAN_POINT('Ctrl Pts',(-16.7428545015778,34.2373406702457,7.58299648829016));
#64967=CARTESIAN_POINT('Ctrl Pts',(-16.7316090177099,34.2324010118935,7.63147080716473));
#64968=CARTESIAN_POINT('Ctrl Pts',(-16.7232095513179,34.2274613535414,7.6806381876418));
#64969=CARTESIAN_POINT('Ctrl Pts',(-16.7177250290144,34.2225216951893,7.73013614611617));
#64970=CARTESIAN_POINT('Ctrl Pts',(-16.7122414978942,34.2175829295507,7.7796251591342));
#64971=CARTESIAN_POINT('Ctrl Pts',(-16.7096719242146,34.2126441639121,7.82944408920579));
#64972=CARTESIAN_POINT('Ctrl Pts',(-16.7100334996795,34.2077053982735,7.87922431913868));
#64973=CARTESIAN_POINT('Ctrl Pts',(-16.7103954139834,34.2027620044261,7.92905119904701));
#64974=CARTESIAN_POINT('Ctrl Pts',(-16.71369395739,34.1978186105788,7.97883875953236));
#64975=CARTESIAN_POINT('Ctrl Pts',(-16.7198941752857,34.1928752167315,8.02821918506006));
#64976=CARTESIAN_POINT('Ctrl Pts',(-16.7260976023264,34.1879292642535,8.07762516919673));
#64977=CARTESIAN_POINT('Ctrl Pts',(-16.7352055959661,34.1829833117755,8.12662306128246));
#64978=CARTESIAN_POINT('Ctrl Pts',(-16.7471318960423,34.1780373592975,8.174854454197));
#64979=CARTESIAN_POINT('Ctrl Pts',(-16.7590798518372,34.1730824259826,8.22317342544435));
#64980=CARTESIAN_POINT('Ctrl Pts',(-16.7738561668314,34.1681274926678,8.27072259772776));
#64981=CARTESIAN_POINT('Ctrl Pts',(-16.7913249557066,34.1631725593529,8.31715952307225));
#64982=CARTESIAN_POINT('Ctrl Pts',(-16.799935976576,34.160730086982,8.34005002430323));
#64983=CARTESIAN_POINT('Ctrl Pts',(-16.8092004992438,34.1582876146111,8.36267058670134));
#64984=CARTESIAN_POINT('Ctrl Pts',(-16.819098120925,34.1558451422402,8.38498235616398));
#64985=CARTESIAN_POINT('Ctrl Pts',(-16.8391628871209,34.1508936863611,8.43021346845593));
#64986=CARTESIAN_POINT('Ctrl Pts',(-16.8619184940994,34.1459422304821,8.47436813249849));
#64987=CARTESIAN_POINT('Ctrl Pts',(-16.8872269071449,34.140990774603,8.51710661218381));
#64988=CARTESIAN_POINT('Ctrl Pts',(-16.9124896153011,34.1360482606415,8.55976790972885));
#64989=CARTESIAN_POINT('Ctrl Pts',(-16.9402957091205,34.13110574668,8.60101762863171));
#64990=CARTESIAN_POINT('Ctrl Pts',(-16.9704601981101,34.1261632327185,8.64053837568294));
#64991=CARTESIAN_POINT('Ctrl Pts',(-17.0005946724359,34.1212256367218,8.6800197982843));
#64992=CARTESIAN_POINT('Ctrl Pts',(-17.0330825656132,34.1162880407251,8.71777522231424));
#64993=CARTESIAN_POINT('Ctrl Pts',(-17.0676954834215,34.1113504447284,8.75351596987858));
#64994=CARTESIAN_POINT('Ctrl Pts',(-17.1022886214296,34.1064156703563,8.78923629313631));
#64995=CARTESIAN_POINT('Ctrl Pts',(-17.1390039983283,34.1014808959843,8.82294382870522));
#64996=CARTESIAN_POINT('Ctrl Pts',(-17.1775745075821,34.0965461216122,8.85438474648779));
#64997=CARTESIAN_POINT('Ctrl Pts',(-17.2161393118952,34.0916120771396,8.8858210138633));
#64998=CARTESIAN_POINT('Ctrl Pts',(-17.2565582793194,34.0866780326671,8.91499098457647));
#64999=CARTESIAN_POINT('Ctrl Pts',(-17.2985311606618,34.0817439881945,8.94168102577725));
#65000=CARTESIAN_POINT('Ctrl Pts',(-17.3405457934919,34.076805035703,8.96839761623778));
#65001=CARTESIAN_POINT('Ctrl Pts',(-17.3841169632708,34.0718660832114,8.99262905895595));
#65002=CARTESIAN_POINT('Ctrl Pts',(-17.428916880813,34.0669271307199,9.01420601106057));
#65003=CARTESIAN_POINT('Ctrl Pts',(-17.473741395472,34.0619854665271,9.03579480985688));
#65004=CARTESIAN_POINT('Ctrl Pts',(-17.519795494874,34.0570438023344,9.0547260078026));
#65005=CARTESIAN_POINT('Ctrl Pts',(-17.5667315843423,34.0521021381416,9.07087851867697));
#65006=CARTESIAN_POINT('Ctrl Pts',(-17.6137556714152,34.0471512091248,9.08706131290645));
#65007=CARTESIAN_POINT('Ctrl Pts',(-17.6616645218855,34.0422002801079,9.1004548750603));
#65008=CARTESIAN_POINT('Ctrl Pts',(-17.7100971451986,34.0372493510911,9.11098849671142));
#65009=CARTESIAN_POINT('Ctrl Pts',(-17.7343622653189,34.0347688972341,9.11626592290024));
#65010=CARTESIAN_POINT('Ctrl Pts',(-17.7587587284728,34.0322884433771,9.12082628997828));
#65011=CARTESIAN_POINT('Ctrl Pts',(-17.7832407132708,34.0298079895202,9.12466560608227));
#65012=CARTESIAN_POINT('Ctrl Pts',(-17.787543982134,34.0293719930134,9.12534045371341));
#65013=CARTESIAN_POINT('Ctrl Pts',(-17.7918507662628,34.0289359965067,9.12599316912035));
#65014=CARTESIAN_POINT('Ctrl Pts',(-17.7961609204192,34.0285,9.12662372762052));
#65015=CARTESIAN_POINT('',(-16.7144063041452,34.0285,7.97570050620834));
#65016=CARTESIAN_POINT('Origin',(-17.98,34.0285,7.87));
#65017=CARTESIAN_POINT('',(-19.249999578241,34.4358804771951,7.86896498015955));
#65018=CARTESIAN_POINT('Ctrl Pts',(-19.2499995766417,34.4359014004106,7.86896301890149));
#65019=CARTESIAN_POINT('Ctrl Pts',(-19.2499454334291,34.429303487383,7.80265336563593));
#65020=CARTESIAN_POINT('Ctrl Pts',(-19.2446942465949,34.4227055743554,7.73656774318384));
#65021=CARTESIAN_POINT('Ctrl Pts',(-19.2343727205358,34.4161076613278,7.67138208042656));
#65022=CARTESIAN_POINT('Ctrl Pts',(-19.2294208866225,34.4129422602719,7.64010874219643));
#65023=CARTESIAN_POINT('Ctrl Pts',(-19.223302717142,34.409776859216,7.6090421404699));
#65024=CARTESIAN_POINT('Ctrl Pts',(-19.2160359553257,34.40661145816,7.57825504778653));
#65025=CARTESIAN_POINT('Ctrl Pts',(-19.2046689857615,34.4016600068298,7.53009660330325));
#65026=CARTESIAN_POINT('Ctrl Pts',(-19.1904586753062,34.3967085554996,7.48249918143714));
#65027=CARTESIAN_POINT('Ctrl Pts',(-19.1734779460725,34.3917571041694,7.43582216519208));
#65028=CARTESIAN_POINT('Ctrl Pts',(-19.1565278826982,34.3868145947703,7.3892294439613));
#65029=CARTESIAN_POINT('Ctrl Pts',(-19.1368175094606,34.3818720853711,7.34355434149111));
#65030=CARTESIAN_POINT('Ctrl Pts',(-19.1144700226763,34.376929575972,7.29914295340351));
#65031=CARTESIAN_POINT('Ctrl Pts',(-19.0921447724198,34.3719919845418,7.25477575619416));
#65032=CARTESIAN_POINT('Ctrl Pts',(-19.0671878484165,34.3670543931117,7.21167027018952));
#65033=CARTESIAN_POINT('Ctrl Pts',(-19.0397704070058,34.3621168016816,7.17015238484737));
#65034=CARTESIAN_POINT('Ctrl Pts',(-19.0123686334772,34.3571820318715,7.12865822518136));
#65035=CARTESIAN_POINT('Ctrl Pts',(-18.9825094291592,34.3522472620613,7.08875032432696));
#65036=CARTESIAN_POINT('Ctrl Pts',(-18.9504084321542,34.3473124922512,7.05072747220235));
#65037=CARTESIAN_POINT('Ctrl Pts',(-18.9183121831044,34.342378452327,7.01271024391541));
#65038=CARTESIAN_POINT('Ctrl Pts',(-18.8839751532307,34.3374444124028,6.97657792775663));
#65039=CARTESIAN_POINT('Ctrl Pts',(-18.8476529763935,34.3325103724785,6.94259592811145));
#65040=CARTESIAN_POINT('Ctrl Pts',(-18.8112946685128,34.3275714244781,6.90858012528547));
#65041=CARTESIAN_POINT('Ctrl Pts',(-18.7729476720726,34.3226324764777,6.87671928311416));
#65042=CARTESIAN_POINT('Ctrl Pts',(-18.7329028661743,34.3176935284773,6.84724036347416));
#65043=CARTESIAN_POINT('Ctrl Pts',(-18.6928360736914,34.3127518687495,6.81774525844512));
#65044=CARTESIAN_POINT('Ctrl Pts',(-18.6510700747914,34.3078102090216,6.79063497815227));
#65045=CARTESIAN_POINT('Ctrl Pts',(-18.6079241248343,34.3028685492938,6.76609271519248));
#65046=CARTESIAN_POINT('Ctrl Pts',(-18.5646972822835,34.2979176246483,6.74150443893814));
#65047=CARTESIAN_POINT('Ctrl Pts',(-18.5200858156786,34.2929667000029,6.71949403160375));
#65048=CARTESIAN_POINT('Ctrl Pts',(-18.4744314489635,34.2880157753574,6.70019764820042));
#65049=CARTESIAN_POINT('Ctrl Pts',(-18.4515579037279,34.2855352853849,6.69052986107689));
#65050=CARTESIAN_POINT('Ctrl Pts',(-18.4284228494437,34.2830547954125,6.68154256543674));
#65051=CARTESIAN_POINT('Ctrl Pts',(-18.4050705842528,34.28057430544,6.67324814668915));
#65052=CARTESIAN_POINT('Ctrl Pts',(-18.3589291304473,34.2756731357871,6.65685930661915));
#65053=CARTESIAN_POINT('Ctrl Pts',(-18.3117254131915,34.2707719661342,6.6431029058274));
#65054=CARTESIAN_POINT('Ctrl Pts',(-18.2637934055715,34.2658707964813,6.63211418016274));
#65055=CARTESIAN_POINT('Ctrl Pts',(-18.2159493949058,34.2609786247408,6.62114562837436));
#65056=CARTESIAN_POINT('Ctrl Pts',(-18.1673802837452,34.2560864530002,6.6129348061338));
#65057=CARTESIAN_POINT('Ctrl Pts',(-18.1184367778866,34.2511942812597,6.60756772121101));
#65058=CARTESIAN_POINT('Ctrl Pts',(-18.0695425146008,34.2463070315842,6.60220603616845));
#65059=CARTESIAN_POINT('Ctrl Pts',(-18.0202751547846,34.2414197819088,6.5996824902367));
#65060=CARTESIAN_POINT('Ctrl Pts',(-17.970994919409,34.2365325322333,6.60003192617942));
#65061=CARTESIAN_POINT('Ctrl Pts',(-17.921742325506,34.2316480238349,6.60038116612218));
#65062=CARTESIAN_POINT('Ctrl Pts',(-17.8724774286441,34.2267635154366,6.60360019434172));
#65063=CARTESIAN_POINT('Ctrl Pts',(-17.823562126101,34.2218790070382,6.60967179210733));
#65064=CARTESIAN_POINT('Ctrl Pts',(-17.7746524847437,34.2169950639457,6.61574268717988));
#65065=CARTESIAN_POINT('Ctrl Pts',(-17.7260929120851,34.2121111208532,6.62466542637155));
#65066=CARTESIAN_POINT('Ctrl Pts',(-17.6782390964949,34.2072271777607,6.63637106181974));
#65067=CARTESIAN_POINT('Ctrl Pts',(-17.6303309640999,34.2023376911148,6.64808998383049));
#65068=CARTESIAN_POINT('Ctrl Pts',(-17.5831307319228,34.1974482044689,6.66259797245389));
#65069=CARTESIAN_POINT('Ctrl Pts',(-17.536980961493,34.192558717823,6.6797755961499));
#65070=CARTESIAN_POINT('Ctrl Pts',(-17.4908030027674,34.187666244677,6.69696371194442));
#65071=CARTESIAN_POINT('Ctrl Pts',(-17.4456772933211,34.1827737715309,6.71682447850852));
#65072=CARTESIAN_POINT('Ctrl Pts',(-17.40192482136,34.1778812983849,6.73919095872013));
#65073=CARTESIAN_POINT('Ctrl Pts',(-17.3580803849902,34.1729785416279,6.76160445159256));
#65074=CARTESIAN_POINT('Ctrl Pts',(-17.3156154268354,34.1680757848709,6.78653388232076));
#65075=CARTESIAN_POINT('Ctrl Pts',(-17.274823394364,34.1631730281139,6.81376803927184));
#65076=CARTESIAN_POINT('Ctrl Pts',(-17.2508725896127,34.1602944029826,6.82975841622004));
#65077=CARTESIAN_POINT('Ctrl Pts',(-17.2274979119499,34.1574157778513,6.84654252814164));
#65078=CARTESIAN_POINT('Ctrl Pts',(-17.2047531057044,34.15453715272,6.86407144742532));
#65079=CARTESIAN_POINT('Ctrl Pts',(-17.1632591851753,34.14928560469,6.89604989454266));
#65080=CARTESIAN_POINT('Ctrl Pts',(-17.1236685159173,34.14403405666,6.93066006210468));
#65081=CARTESIAN_POINT('Ctrl Pts',(-17.0863201058028,34.13878250863,6.96764959871027));
#65082=CARTESIAN_POINT('Ctrl Pts',(-17.0502648631405,34.1337127924629,7.00335839365478));
#65083=CARTESIAN_POINT('Ctrl Pts',(-17.0162995457397,34.1286430762957,7.04128408624179));
#65084=CARTESIAN_POINT('Ctrl Pts',(-16.9846970405727,34.1235733601286,7.08115779844429));
#65085=CARTESIAN_POINT('Ctrl Pts',(-16.9531357999906,34.1185102636814,7.12097944603434));
#65086=CARTESIAN_POINT('Ctrl Pts',(-16.9239315670765,34.1134471672341,7.16274366761761));
#65087=CARTESIAN_POINT('Ctrl Pts',(-16.897318768203,34.1083840707869,7.20614658973942));
#65088=CARTESIAN_POINT('Ctrl Pts',(-16.8707316582046,34.1033258616593,7.24950761577028));
#65089=CARTESIAN_POINT('Ctrl Pts',(-16.8467312842112,34.0982676525316,7.29450376745023));
#65090=CARTESIAN_POINT('Ctrl Pts',(-16.8255090619546,34.0932094434039,7.34080185755137));
#65091=CARTESIAN_POINT('Ctrl Pts',(-16.8043001092413,34.0881543970046,7.3870709990106));
#65092=CARTESIAN_POINT('Ctrl Pts',(-16.785866071209,34.0830993506054,7.43463999713855));
#65093=CARTESIAN_POINT('Ctrl Pts',(-16.7703516593605,34.0780443042061,7.48315262442644));
#65094=CARTESIAN_POINT('Ctrl Pts',(-16.7548369971137,34.0729891762198,7.53166603469493));
#65095=CARTESIAN_POINT('Ctrl Pts',(-16.7422422219879,34.0679340482334,7.58112262009095));
#65096=CARTESIAN_POINT('Ctrl Pts',(-16.7326626587095,34.0628789202471,7.63114950905991));
#65097=CARTESIAN_POINT('Ctrl Pts',(-16.7230831325064,34.0578238118254,7.68117620441224));
#65098=CARTESIAN_POINT('Ctrl Pts',(-16.7165188826359,34.0527687034036,7.73177269408068));
#65099=CARTESIAN_POINT('Ctrl Pts',(-16.7130139277447,34.0477135949819,7.78255691730597));
#65100=CARTESIAN_POINT('Ctrl Pts',(-16.7095063931632,34.0426547659376,7.83337851835005));
#65101=CARTESIAN_POINT('Ctrl Pts',(-16.7090626718887,34.0375959368933,7.88438761672372));
#65102=CARTESIAN_POINT('Ctrl Pts',(-16.7116747290644,34.032537107849,7.93519974774569));
#65103=CARTESIAN_POINT('Ctrl Pts',(-16.712369564202,34.0311914052327,7.94871631789656));
#65104=CARTESIAN_POINT('Ctrl Pts',(-16.713280345878,34.0298457026163,7.96221896542966));
#65105=CARTESIAN_POINT('Ctrl Pts',(-16.7144063041452,34.0285,7.97570050620834));
#65106=CARTESIAN_POINT('Ctrl Pts',(-19.2499995788896,34.435871992073,7.86896577552077));
#65107=CARTESIAN_POINT('Ctrl Pts',(-19.2500561832405,34.4423874535631,7.93847438149077));
#65108=CARTESIAN_POINT('Ctrl Pts',(-19.2444064699017,34.448898524241,8.00786438420913));
#65109=CARTESIAN_POINT('Ctrl Pts',(-19.2297862522652,34.4575354975776,8.09661020094649));
#65110=CARTESIAN_POINT('Ctrl Pts',(-19.2259771711595,34.4595105479342,8.1166954469874));
#65111=CARTESIAN_POINT('Ctrl Pts',(-19.218134183589,34.4631464043062,8.15321324412816));
#65112=CARTESIAN_POINT('Ctrl Pts',(-19.214253362788,34.4648022192572,8.16967410323797));
#65113=CARTESIAN_POINT('Ctrl Pts',(-19.2055381018845,34.4682533448045,8.20359313464447));
#65114=CARTESIAN_POINT('Ctrl Pts',(-19.2006565261306,34.4700498023201,8.22103500930035));
#65115=CARTESIAN_POINT('Ctrl Pts',(-19.1885295438783,34.474225864029,8.26104740325841));
#65116=CARTESIAN_POINT('Ctrl Pts',(-19.1810221144874,34.4766134614314,8.28353043061039));
#65117=CARTESIAN_POINT('Ctrl Pts',(-19.1396848304862,34.48885402516,8.39668365613964));
#65118=CARTESIAN_POINT('Ctrl Pts',(-19.0962061968643,34.4990205318921,8.48346514625448));
#65119=CARTESIAN_POINT('Ctrl Pts',(-19.0218803611092,34.5133528401569,8.59727026210805));
#65120=CARTESIAN_POINT('Ctrl Pts',(-18.9989352040304,34.5174792966232,8.62908378191094));
#65121=CARTESIAN_POINT('Ctrl Pts',(-18.9587636195176,34.5242007179762,8.67967059086213));
#65122=CARTESIAN_POINT('Ctrl Pts',(-18.9423791036808,34.5268214051788,8.69907866701827));
#65123=CARTESIAN_POINT('Ctrl Pts',(-18.917345419193,34.5306399845124,8.72698884109266));
#65124=CARTESIAN_POINT('Ctrl Pts',(-18.9091401754607,34.5318640272109,8.73587810070143));
#65125=CARTESIAN_POINT('Ctrl Pts',(-18.8936886793601,34.5341166862003,8.75214504195841));
#65126=CARTESIAN_POINT('Ctrl Pts',(-18.8864778356671,34.5351473863616,8.7595531618484));
#65127=CARTESIAN_POINT('Ctrl Pts',(-18.86772814022,34.5377773886837,8.77835100657601));
#65128=CARTESIAN_POINT('Ctrl Pts',(-18.8560600923456,34.5393669515313,8.78960948747787));
#65129=CARTESIAN_POINT('Ctrl Pts',(-18.8330834518678,34.5424159449781,8.81094520262985));
#65130=CARTESIAN_POINT('Ctrl Pts',(-18.8218085718806,34.5438761809861,8.82104536020224));
#65131=CARTESIAN_POINT('Ctrl Pts',(-18.8103597424409,34.5453270911211,8.83093844658933));
#65132=CARTESIAN_POINT('Origin',(-17.98,34.0285,7.87));
#65133=CARTESIAN_POINT('',(-18.5116348366204,34.0285,6.25069791697424));
#65134=CARTESIAN_POINT('',(-19.68434,34.0285,7.87));
#65135=CARTESIAN_POINT('Origin',(-17.98,34.0285,7.87));
#65136=CARTESIAN_POINT('Ctrl Pts',(-18.5116348366204,34.0285,6.25069791697424));
#65137=CARTESIAN_POINT('Ctrl Pts',(-18.4477983675585,34.0285,6.23870611066214));
#65138=CARTESIAN_POINT('Ctrl Pts',(-18.3832442000431,34.0285,6.23070689758999));
#65139=CARTESIAN_POINT('Ctrl Pts',(-18.3183243142307,34.0285,6.22660131571174));
#65140=CARTESIAN_POINT('Ctrl Pts',(-18.2609661061129,34.0285,6.22297393995667));
#65141=CARTESIAN_POINT('Ctrl Pts',(-18.2033219294552,34.0285,6.22238700818959));
#65142=CARTESIAN_POINT('Ctrl Pts',(-18.1456465741428,34.0285,6.22480389998478));
#65143=CARTESIAN_POINT('Ctrl Pts',(-18.1314043910992,34.0285,6.22540072015445));
#65144=CARTESIAN_POINT('Ctrl Pts',(-18.1171699644767,34.0285,6.22618044836808));
#65145=CARTESIAN_POINT('Ctrl Pts',(-18.1029488004271,34.0285,6.2271419028461));
#65146=CARTESIAN_POINT('Ctrl Pts',(-18.039457939995,34.0285,6.23143434837749));
#65147=CARTESIAN_POINT('Ctrl Pts',(-17.9762179002088,34.0285,6.23934585586296));
#65148=CARTESIAN_POINT('Ctrl Pts',(-17.9135732010023,34.0285,6.25080658082955));
#65149=CARTESIAN_POINT('Ctrl Pts',(-17.8717765066452,34.0285,6.2584532041609));
#65150=CARTESIAN_POINT('Ctrl Pts',(-17.8302452091138,34.0285,6.26768078671085));
#65151=CARTESIAN_POINT('Ctrl Pts',(-17.7890894280646,34.0285,6.27847894017026));
#65152=CARTESIAN_POINT('Ctrl Pts',(-17.7738772006603,34.0285,6.28247021337135));
#65153=CARTESIAN_POINT('Ctrl Pts',(-17.7587122268377,34.0285,6.28667749313672));
#65154=CARTESIAN_POINT('Ctrl Pts',(-17.7436272591778,34.0285,6.29109218874144));
#65155=CARTESIAN_POINT('Ctrl Pts',(-17.684577575458,34.0285,6.30837339113148));
#65156=CARTESIAN_POINT('Ctrl Pts',(-17.6266753461434,34.0285,6.32884750660487));
#65157=CARTESIAN_POINT('Ctrl Pts',(-17.5702302830355,34.0285,6.35244256448365));
#65158=CARTESIAN_POINT('Ctrl Pts',(-17.5152199185782,34.0285,6.37543789236239));
#65159=CARTESIAN_POINT('Ctrl Pts',(-17.4615928472096,34.0285,6.40139816138878));
#65160=CARTESIAN_POINT('Ctrl Pts',(-17.4096690783012,34.0285,6.4302922821505));
#65161=CARTESIAN_POINT('Ctrl Pts',(-17.3782632796365,34.0285,6.44776872806942));
#65162=CARTESIAN_POINT('Ctrl Pts',(-17.3474813084972,34.0285,6.46631913073517));
#65163=CARTESIAN_POINT('Ctrl Pts',(-17.3174017826758,34.0285,6.48594174657202));
#65164=CARTESIAN_POINT('Ctrl Pts',(-17.2924442615412,34.0285,6.50222298226608));
#65165=CARTESIAN_POINT('Ctrl Pts',(-17.267970417772,34.0285,6.51924244114969));
#65166=CARTESIAN_POINT('Ctrl Pts',(-17.2440288126058,34.0285,6.53700081495576));
#65167=CARTESIAN_POINT('Ctrl Pts',(-17.2333815441399,34.0285,6.5448982876657));
#65168=CARTESIAN_POINT('Ctrl Pts',(-17.2228371138846,34.0285,6.55294403764358));
#65169=CARTESIAN_POINT('Ctrl Pts',(-17.2124195643277,34.0285,6.56112233024434));
#65170=CARTESIAN_POINT('Ctrl Pts',(-17.1676647316062,34.0285,6.59625709157124));
#65171=CARTESIAN_POINT('Ctrl Pts',(-17.1251724160825,34.0285,6.63388991678137));
#65172=CARTESIAN_POINT('Ctrl Pts',(-17.0852264667732,34.0285,6.67398593907778));
#65173=CARTESIAN_POINT('Ctrl Pts',(-17.080151930788,34.0285,6.6790795395936));
#65174=CARTESIAN_POINT('Ctrl Pts',(-17.0751185456676,34.0285,6.68421292889612));
#65175=CARTESIAN_POINT('Ctrl Pts',(-17.0701269456468,34.0285,6.68938606742345));
#65176=CARTESIAN_POINT('Ctrl Pts',(-17.029744147875,34.0285,6.73123753912078));
#65177=CARTESIAN_POINT('Ctrl Pts',(-16.9920920490028,34.0285,6.77568953714568));
#65178=CARTESIAN_POINT('Ctrl Pts',(-16.9572880675087,34.0285,6.82243210278544));
#65179=CARTESIAN_POINT('Ctrl Pts',(-16.9270997258523,34.0285,6.86297575557615));
#65180=CARTESIAN_POINT('Ctrl Pts',(-16.8990548859259,34.0285,6.90524353527338));
#65181=CARTESIAN_POINT('Ctrl Pts',(-16.8732618745741,34.0285,6.94903484153182));
#65182=CARTESIAN_POINT('Ctrl Pts',(-16.8681371425678,34.0285,6.95773559793896));
#65183=CARTESIAN_POINT('Ctrl Pts',(-16.8631002530348,34.0285,6.96649853884193));
#65184=CARTESIAN_POINT('Ctrl Pts',(-16.858155953323,34.0285,6.97531533866574));
#65185=CARTESIAN_POINT('Ctrl Pts',(-16.8306640666196,34.0285,7.02433956372781));
#65186=CARTESIAN_POINT('Ctrl Pts',(-16.8061063757587,34.0285,7.07488941615454));
#65187=CARTESIAN_POINT('Ctrl Pts',(-16.7845650810918,34.0285,7.12667245441139));
#65188=CARTESIAN_POINT('Ctrl Pts',(-16.763360070835,34.0285,7.17764709982381));
#65189=CARTESIAN_POINT('Ctrl Pts',(-16.7450780721175,34.0285,7.22981788604346));
#65190=CARTESIAN_POINT('Ctrl Pts',(-16.7298468231901,34.0285,7.28290675957567));
#65191=CARTESIAN_POINT('Ctrl Pts',(-16.7147402924653,34.0285,7.33556092490247));
#65192=CARTESIAN_POINT('Ctrl Pts',(-16.7026347861426,34.0285,7.38911923149214));
#65193=CARTESIAN_POINT('Ctrl Pts',(-16.6937032695783,34.0285,7.44329516703774));
#65194=CARTESIAN_POINT('Ctrl Pts',(-16.6920623691379,34.0285,7.45324838336542));
#65195=CARTESIAN_POINT('Ctrl Pts',(-16.6905287322653,34.0285,7.46322238082028));
#65196=CARTESIAN_POINT('Ctrl Pts',(-16.6891036091325,34.0285,7.47321528432834));
#65197=CARTESIAN_POINT('Ctrl Pts',(-16.6875741705604,34.0285,7.48393964331189));
#65198=CARTESIAN_POINT('Ctrl Pts',(-16.686170862869,34.0285,7.49467810037056));
#65199=CARTESIAN_POINT('Ctrl Pts',(-16.6848954111995,34.0285,7.50542132298178));
#65200=CARTESIAN_POINT('Ctrl Pts',(-16.6786799335084,34.0285,7.55777474574567));
#65201=CARTESIAN_POINT('Ctrl Pts',(-16.6754890773626,34.0285,7.61029605110518));
#65202=CARTESIAN_POINT('Ctrl Pts',(-16.6754319365421,34.0285,7.66273374271887));
#65203=CARTESIAN_POINT('Ctrl Pts',(-16.6753745061326,34.0285,7.71543718793836));
#65204=CARTESIAN_POINT('Ctrl Pts',(-16.6784826472741,34.0285,7.7680571926682));
#65205=CARTESIAN_POINT('Ctrl Pts',(-16.6849167607292,34.0285,7.82031641789131));
#65206=CARTESIAN_POINT('Ctrl Pts',(-16.6910111090541,34.0285,7.86981599913381));
#65207=CARTESIAN_POINT('Ctrl Pts',(-16.7000898992755,34.0285,7.91899240774701));
#65208=CARTESIAN_POINT('Ctrl Pts',(-16.712329638489,34.0285,7.96757972342322));
#65209=CARTESIAN_POINT('Ctrl Pts',(-16.7130120144162,34.0285,7.97028850781839));
#65210=CARTESIAN_POINT('Ctrl Pts',(-16.7137042249467,34.0285,7.97299545191025));
#65211=CARTESIAN_POINT('Ctrl Pts',(-16.7144063041452,34.0285,7.97570050620834));
#65212=CARTESIAN_POINT('Ctrl Pts',(-17.7958274652882,34.0285,9.12890304511207));
#65213=CARTESIAN_POINT('Ctrl Pts',(-17.8438421718885,34.0285,9.14456709927581));
#65214=CARTESIAN_POINT('Ctrl Pts',(-17.89277854746,34.0285,9.15703166260375));
#65215=CARTESIAN_POINT('Ctrl Pts',(-17.9423455702771,34.0285,9.16645118943153));
#65216=CARTESIAN_POINT('Ctrl Pts',(-17.9788483505988,34.0285,9.1733880377429));
#65217=CARTESIAN_POINT('Ctrl Pts',(-18.0156941104094,34.0285,9.17867267409858));
#65218=CARTESIAN_POINT('Ctrl Pts',(-18.0527778734286,34.0285,9.18235277161469));
#65219=CARTESIAN_POINT('Ctrl Pts',(-18.0659311497185,34.0285,9.1836580690134));
#65220=CARTESIAN_POINT('Ctrl Pts',(-18.079116397763,34.0285,9.18476152516703));
#65221=CARTESIAN_POINT('Ctrl Pts',(-18.0923229261104,34.0285,9.18566448225191));
#65222=CARTESIAN_POINT('Ctrl Pts',(-18.1454432003452,34.0285,9.18929642296404));
#65223=CARTESIAN_POINT('Ctrl Pts',(-18.1987891581145,34.0285,9.18968112794214));
#65224=CARTESIAN_POINT('Ctrl Pts',(-18.2520569989133,34.0285,9.18697003409754));
#65225=CARTESIAN_POINT('Ctrl Pts',(-18.2901479978194,34.0285,9.18503137333863));
#65226=CARTESIAN_POINT('Ctrl Pts',(-18.3281998805904,34.0285,9.18150876304076));
#65227=CARTESIAN_POINT('Ctrl Pts',(-18.3661092456966,34.0285,9.17644326610694));
#65228=CARTESIAN_POINT('Ctrl Pts',(-18.3781547717082,34.0285,9.17483372780664));
#65229=CARTESIAN_POINT('Ctrl Pts',(-18.3901878310136,34.0285,9.17306802072464));
#65230=CARTESIAN_POINT('Ctrl Pts',(-18.4021992137758,34.0285,9.17114816946817));
#65231=CARTESIAN_POINT('Ctrl Pts',(-18.4576095783033,34.0285,9.16229159899116));
#65232=CARTESIAN_POINT('Ctrl Pts',(-18.5123949314096,34.0285,9.15018542975578));
#65233=CARTESIAN_POINT('Ctrl Pts',(-18.5662341053607,34.0285,9.13499667932461));
#65234=CARTESIAN_POINT('Ctrl Pts',(-18.6200732793119,34.0285,9.11980792889344));
#65235=CARTESIAN_POINT('Ctrl Pts',(-18.6729674045624,34.0285,9.10153660156417));
#65236=CARTESIAN_POINT('Ctrl Pts',(-18.7246136905742,34.0285,9.08030056607039));
#65237=CARTESIAN_POINT('Ctrl Pts',(-18.7576957896348,34.0285,9.06669779452361));
#65238=CARTESIAN_POINT('Ctrl Pts',(-18.7902662184505,34.0285,9.0518775916147));
#65239=CARTESIAN_POINT('Ctrl Pts',(-18.8222460418491,34.0285,9.03586036752327));
#65240=CARTESIAN_POINT('Ctrl Pts',(-18.8502323779702,34.0285,9.02184329771136));
#65241=CARTESIAN_POINT('Ctrl Pts',(-18.8777664606405,34.0285,9.0069093719839));
#65242=CARTESIAN_POINT('Ctrl Pts',(-18.9047943322193,34.0285,8.99106711939537));
#65243=CARTESIAN_POINT('Ctrl Pts',(-18.913064824246,34.0285,8.98621941160102));
#65244=CARTESIAN_POINT('Ctrl Pts',(-18.9212849235068,34.0285,8.9812882991084));
#65245=CARTESIAN_POINT('Ctrl Pts',(-18.9294459656864,34.0285,8.97627873609161));
#65246=CARTESIAN_POINT('Ctrl Pts',(-18.9797430547245,34.0285,8.94540443945738));
#65247=CARTESIAN_POINT('Ctrl Pts',(-19.0278778119151,34.0285,8.91150716656161));
#65248=CARTESIAN_POINT('Ctrl Pts',(-19.0735206728694,34.0285,8.87472873332212));
#65249=CARTESIAN_POINT('Ctrl Pts',(-19.0792370626728,34.0285,8.87012253957442));
#65250=CARTESIAN_POINT('Ctrl Pts',(-19.0849143688835,34.0285,8.86547108651176));
#65251=CARTESIAN_POINT('Ctrl Pts',(-19.0905519435273,34.0285,8.86077459547289));
#65252=CARTESIAN_POINT('Ctrl Pts',(-19.1339677064135,34.0285,8.82460625106497));
#65253=CARTESIAN_POINT('Ctrl Pts',(-19.1750287637336,34.0285,8.78577085039626));
#65254=CARTESIAN_POINT('Ctrl Pts',(-19.2137029428852,34.0285,8.74456929570144));
#65255=CARTESIAN_POINT('Ctrl Pts',(-19.234699233103,34.0285,8.72220088818067));
#65256=CARTESIAN_POINT('Ctrl Pts',(-19.2549916655178,34.0285,8.69913421137922));
#65257=CARTESIAN_POINT('Ctrl Pts',(-19.2745721746555,34.0285,8.67541188309048));
#65258=CARTESIAN_POINT('Ctrl Pts',(-19.2887649969517,34.0285,8.65821688639835));
#65259=CARTESIAN_POINT('Ctrl Pts',(-19.3025837319496,34.0285,8.64067733049516));
#65260=CARTESIAN_POINT('Ctrl Pts',(-19.3160244998568,34.0285,8.62280834510891));
#65261=CARTESIAN_POINT('Ctrl Pts',(-19.3251656884946,34.0285,8.61065548544268));
#65262=CARTESIAN_POINT('Ctrl Pts',(-19.3341353501016,34.0285,8.59834525568747));
#65263=CARTESIAN_POINT('Ctrl Pts',(-19.3429129178832,34.0285,8.58591015550462));
#65264=CARTESIAN_POINT('Ctrl Pts',(-19.3772396241466,34.0285,8.53727982396515));
#65265=CARTESIAN_POINT('Ctrl Pts',(-19.4086800748933,34.0285,8.48668186632755));
#65266=CARTESIAN_POINT('Ctrl Pts',(-19.4372102427494,34.0285,8.43446034078614));
#65267=CARTESIAN_POINT('Ctrl Pts',(-19.4666484450477,34.0285,8.38057675198429));
#65268=CARTESIAN_POINT('Ctrl Pts',(-19.4929888584362,34.0285,8.32496401828332));
#65269=CARTESIAN_POINT('Ctrl Pts',(-19.5161757455008,34.0285,8.26795179493227));
#65270=CARTESIAN_POINT('Ctrl Pts',(-19.5393626325653,34.0285,8.21093957158123));
#65271=CARTESIAN_POINT('Ctrl Pts',(-19.5593965687678,34.0285,8.15252693850102));
#65272=CARTESIAN_POINT('Ctrl Pts',(-19.5761835248491,34.0285,8.09300780438079));
#65273=CARTESIAN_POINT('Ctrl Pts',(-19.5793637812432,34.0285,8.08173201942358));
#65274=CARTESIAN_POINT('Ctrl Pts',(-19.5824273766733,34.0285,8.07041644188063));
#65275=CARTESIAN_POINT('Ctrl Pts',(-19.5853734902581,34.0285,8.05906296865037));
#65276=CARTESIAN_POINT('Ctrl Pts',(-19.5884200416724,34.0285,8.0473224369528));
#65277=CARTESIAN_POINT('Ctrl Pts',(-19.5913389660892,34.0285,8.03554884052617));
#65278=CARTESIAN_POINT('Ctrl Pts',(-19.5941280042834,34.0285,8.02375265392161));
#65279=CARTESIAN_POINT('Ctrl Pts',(-19.6089012698,34.0285,7.9612693945833));
#65280=CARTESIAN_POINT('Ctrl Pts',(-19.6200513196573,34.0285,7.89808613178614));
#65281=CARTESIAN_POINT('Ctrl Pts',(-19.6275294811123,34.0285,7.83455530273799));
#65282=CARTESIAN_POINT('Ctrl Pts',(-19.6350208727503,34.0285,7.77091207647897));
#65283=CARTESIAN_POINT('Ctrl Pts',(-19.6388279358374,34.0285,7.70691905863735));
#65284=CARTESIAN_POINT('Ctrl Pts',(-19.6388604237698,34.0285,7.64289952645537));
#65285=CARTESIAN_POINT('Ctrl Pts',(-19.6388926236947,34.0285,7.57944753110339));
#65286=CARTESIAN_POINT('Ctrl Pts',(-19.6352173525578,34.0285,7.51596845155174));
#65287=CARTESIAN_POINT('Ctrl Pts',(-19.6276985634618,34.0285,7.45276180285684));
#65288=CARTESIAN_POINT('Ctrl Pts',(-19.626277169771,34.0285,7.44081286659565));
#65289=CARTESIAN_POINT('Ctrl Pts',(-19.6247182640679,34.0285,7.42887364845075));
#65290=CARTESIAN_POINT('Ctrl Pts',(-19.6230207093981,34.0285,7.41694615762716));
#65291=CARTESIAN_POINT('Origin',(-17.98,34.0285,7.87));
#65292=CARTESIAN_POINT('Ctrl Pts',(-18.5714796494485,41.7180970761119,8.99125045312017));
#65293=CARTESIAN_POINT('Ctrl Pts',(-18.9443656600646,41.6760846918719,8.79454641948545));
#65294=CARTESIAN_POINT('Ctrl Pts',(-19.4718969281881,41.5920599233919,8.00298830736167));
#65295=CARTESIAN_POINT('Ctrl Pts',(-18.9000484458028,41.4660227706719,6.68614628737439));
#65296=CARTESIAN_POINT('Ctrl Pts',(-17.4844919540699,41.3399856179519,6.45621531221888));
#65297=CARTESIAN_POINT('Ctrl Pts',(-16.5232775015748,41.213948465232,7.51911552834859));
#65298=CARTESIAN_POINT('Ctrl Pts',(-16.8953504400754,41.0879113125119,8.90400264567513));
#65299=CARTESIAN_POINT('Ctrl Pts',(-18.2606051857913,40.961874159792,9.34187611889218));
#65300=CARTESIAN_POINT('Ctrl Pts',(-19.368874647327,40.8358370070719,8.43242596995452));
#65301=CARTESIAN_POINT('Ctrl Pts',(-19.2056642802028,40.709799854352,7.00797545227637));
#65302=CARTESIAN_POINT('Ctrl Pts',(-17.9203268783257,40.5837627016319,6.37276257178433));
#65303=CARTESIAN_POINT('Ctrl Pts',(-16.6896320092116,40.457725548912,7.10825717650556));
#65304=CARTESIAN_POINT('Ctrl Pts',(-16.6402725882592,40.3316883961919,8.54114494966668));
#65305=CARTESIAN_POINT('Ctrl Pts',(-17.8174461113438,40.205651243472,9.3595885920492));
#65306=CARTESIAN_POINT('Ctrl Pts',(-19.143437440358,40.079614090752,8.81430625229477));
#65307=CARTESIAN_POINT('Ctrl Pts',(-19.404294163858,39.953576938032,7.40450320966821));
#65308=CARTESIAN_POINT('Ctrl Pts',(-18.3611989837821,39.827539785312,6.42086660001849));
#65309=CARTESIAN_POINT('Ctrl Pts',(-16.9691135802101,39.701502632592,6.76392163550818));
#65310=CARTESIAN_POINT('Ctrl Pts',(-16.5025018622442,39.575465479872,8.11959955528859));
#65311=CARTESIAN_POINT('Ctrl Pts',(-17.3885503485607,39.449428327152,9.24676719033193));
#65312=CARTESIAN_POINT('Ctrl Pts',(-18.8160752155619,39.323391174432,9.11349462344888));
#65313=CARTESIAN_POINT('Ctrl Pts',(-19.4781672291768,39.197354021712,7.84179377198361));
#65314=CARTESIAN_POINT('Ctrl Pts',(-18.7686763775428,39.071316868992,6.59591593747959));
#65315=CARTESIAN_POINT('Ctrl Pts',(-17.3371466403695,38.945279716272,6.51647120732814));
#65316=CARTESIAN_POINT('Ctrl Pts',(-16.494153769907,38.819242563552,7.67619181215477));
#65317=CARTESIAN_POINT('Ctrl Pts',(-17.0114637963517,38.693205410832,9.0133452034285));
#65318=CARTESIAN_POINT('Ctrl Pts',(-18.415475673635,38.567168258112,9.30375784937852));
#65319=CARTESIAN_POINT('Ctrl Pts',(-19.4208064439724,38.441131105392,8.28155488545429));
#65320=CARTESIAN_POINT('Ctrl Pts',(-19.1070685657665,38.315093952672,6.88257046799409));
#65321=CARTESIAN_POINT('Ctrl Pts',(-17.761491320168,38.189056799952,6.38758487946864));
#65322=CARTESIAN_POINT('Ctrl Pts',(-16.6159603404313,38.063019647232,7.24976098169606));
#65323=CARTESIAN_POINT('Ctrl Pts',(-16.7192174666317,37.936982494512,8.67977036019592));
#65324=CARTESIAN_POINT('Ctrl Pts',(-17.9767300580474,37.810945341792,9.36842915754399));
#65325=CARTESIAN_POINT('Ctrl Pts',(-19.2372363048034,37.6849081890721,8.68526529828479));
#65326=CARTESIAN_POINT('Ctrl Pts',(-19.3467336840785,37.558871036352,7.25572020255653));
#65327=CARTESIAN_POINT('Ctrl Pts',(-18.2049765586077,37.4328338836321,6.38855267366891));
#65328=CARTESIAN_POINT('Ctrl Pts',(-16.8572517778355,37.306796730912,6.87766081284674));
#65329=CARTESIAN_POINT('Ctrl Pts',(-16.537411058784,37.1807595781921,8.27526260580466));
#65330=CARTESIAN_POINT('Ctrl Pts',(-17.5382708774487,37.054722425472,9.30184357185776));
#65331=CARTESIAN_POINT('Ctrl Pts',(-18.9435368801747,36.928685272752,9.01756146401863));
#65332=CARTESIAN_POINT('Ctrl Pts',(-19.466677949177,36.8026481200321,7.68267859169109));
#65333=CARTESIAN_POINT('Ctrl Pts',(-18.628754675352,36.676610967312,6.5192898171438));
#65334=CARTESIAN_POINT('Ctrl Pts',(-17.1968918401205,36.5505738145921,6.59248591091588));
#65335=CARTESIAN_POINT('Ctrl Pts',(-16.4819701427196,36.424536661872,7.83525534113844));
#65336=CARTESIAN_POINT('Ctrl Pts',(-17.1385055544403,36.2984995091521,9.10983373266509));
#65337=CARTESIAN_POINT('Ctrl Pts',(-18.5654351459831,36.172462356432,9.24933548309321));
#65338=CARTESIAN_POINT('Ctrl Pts',(-19.4563947146754,36.0464252037121,8.12604559865597));
#65339=CARTESIAN_POINT('Ctrl Pts',(-18.9957042014948,35.9203880509921,6.7683443136604));
#65340=CARTESIAN_POINT('Ctrl Pts',(-17.6051294267902,35.7943508982721,6.41921635646431));
#65341=CARTESIAN_POINT('Ctrl Pts',(-16.5577508962692,35.6683137455521,7.39829197305275));
#65342=CARTESIAN_POINT('Ctrl Pts',(-16.8124525466696,35.5422765928321,8.80921823049927));
#65343=CARTESIAN_POINT('Ctrl Pts',(-18.1360504665275,35.4162394401121,9.3602863258882));
#65344=CARTESIAN_POINT('Ctrl Pts',(-19.3167866617019,35.2902022873921,8.54698087261944));
#65345=CARTESIAN_POINT('Ctrl Pts',(-19.2736779139766,35.1641651346721,7.11390592332082));
#65346=CARTESIAN_POINT('Ctrl Pts',(-18.0462119602502,35.0381279819521,6.37301796104198));
#65347=CARTESIAN_POINT('Ctrl Pts',(-16.7581002235375,34.9120908292321,7.00267267196968));
#65348=CARTESIAN_POINT('Ctrl Pts',(-16.5887026766086,34.7860536765121,8.42628260585971));
#65349=CARTESIAN_POINT('Ctrl Pts',(-17.6929361751755,34.6600165237921,9.34078907379165));
#65350=CARTESIAN_POINT('Ctrl Pts',(-19.0602006334414,34.5339793710721,8.90842522185144));
#65351=CARTESIAN_POINT('Ctrl Pts',(-19.4380918746699,34.4079422183521,7.52607638637724));
#65352=CARTESIAN_POINT('Ctrl Pts',(-18.4819749584899,34.2819050656321,6.45719431747657));
#65353=CARTESIAN_POINT('Ctrl Pts',(-17.0643238211113,34.1558567053176,6.68460455611039));
#65354=CARTESIAN_POINT('Ctrl Pts',(-16.6815128915769,34.071820729243,7.55561568178109));
#65355=CARTESIAN_POINT('Ctrl Pts',(-16.7167313810425,34.0297971374084,7.97584489432982));
#65356=CARTESIAN_POINT('Ctrl Pts',(-18.6397356458259,41.6336362795415,9.12064132385885));
#65357=CARTESIAN_POINT('Ctrl Pts',(-19.0556522259867,41.5916238953015,8.90123789588367));
#65358=CARTESIAN_POINT('Ctrl Pts',(-19.6440599289284,41.5075991268215,8.01833498823901));
#65359=CARTESIAN_POINT('Ctrl Pts',(-19.0062208617807,41.3815619741013,6.54953108041721));
#65360=CARTESIAN_POINT('Ctrl Pts',(-17.4273109582073,41.2555248213815,6.29306636429208));
#65361=CARTESIAN_POINT('Ctrl Pts',(-16.3551735851203,41.1294876686615,7.47862390831015));
#65362=CARTESIAN_POINT('Ctrl Pts',(-16.7701832656815,41.0034505159415,9.02332523082788));
#65363=CARTESIAN_POINT('Ctrl Pts',(-18.2929866659701,40.8774133632215,9.51172874380123));
#65364=CARTESIAN_POINT('Ctrl Pts',(-19.5291490083893,40.7513762105015,8.49732920881249));
#65365=CARTESIAN_POINT('Ctrl Pts',(-19.3471043732769,40.6253390577815,6.90849892005496));
#65366=CARTESIAN_POINT('Ctrl Pts',(-17.9134406762718,40.4993019050615,6.19998328415929));
#65367=CARTESIAN_POINT('Ctrl Pts',(-16.540725190546,40.3732647523415,7.02035302722595));
#65368=CARTESIAN_POINT('Ctrl Pts',(-16.4856697554351,40.2472275996215,8.61859421997696));
#65369=CARTESIAN_POINT('Ctrl Pts',(-17.7986876001328,40.1211904469015,9.53148521374625));
#65370=CARTESIAN_POINT('Ctrl Pts',(-19.2776966355619,39.9951532941815,8.9232779881709));
#65371=CARTESIAN_POINT('Ctrl Pts',(-19.5686558919062,39.8691161414615,7.35078547438482));
#65372=CARTESIAN_POINT('Ctrl Pts',(-18.4051888598166,39.7430789887415,6.25363845583508));
#65373=CARTESIAN_POINT('Ctrl Pts',(-16.852458578011,39.6170418360215,6.63628160442634));
#65374=CARTESIAN_POINT('Ctrl Pts',(-16.3320004635361,39.4910046833015,8.14840302529378));
#65375=CARTESIAN_POINT('Ctrl Pts',(-17.3202978139153,39.3649675305815,9.40564436631503));
#65376=CARTESIAN_POINT('Ctrl Pts',(-18.9125572279824,39.2389303778615,9.2569923153688));
#65377=CARTESIAN_POINT('Ctrl Pts',(-19.6510538146457,39.1128932251415,7.83853880928271));
#65378=CARTESIAN_POINT('Ctrl Pts',(-18.8596886245723,38.9868560724214,6.44888826334574));
#65379=CARTESIAN_POINT('Ctrl Pts',(-17.2629621834282,38.8608189197014,6.36027571276549));
#65380=CARTESIAN_POINT('Ctrl Pts',(-16.3226890120016,38.7347817669814,7.65382659472116));
#65381=CARTESIAN_POINT('Ctrl Pts',(-16.8996959550249,38.6087446142615,9.14528578014338));
#65382=CARTESIAN_POINT('Ctrl Pts',(-18.465729010381,38.4827074615415,9.46921167465304));
#65383=CARTESIAN_POINT('Ctrl Pts',(-19.5870736680637,38.3566703088215,8.3290477937849));
#65384=CARTESIAN_POINT('Ctrl Pts',(-19.2371308392764,38.2306331561015,6.76862236069675));
#65385=CARTESIAN_POINT('Ctrl Pts',(-17.7362756974954,38.1045960033815,6.21651606722604));
#65386=CARTESIAN_POINT('Ctrl Pts',(-16.4585519052485,37.9785588506615,7.1781861908711));
#65387=CARTESIAN_POINT('Ctrl Pts',(-16.5737247719793,37.8525216979416,8.77321682589191));
#65388=CARTESIAN_POINT('Ctrl Pts',(-17.976352710921,37.7264845452215,9.541345969212));
#65389=CARTESIAN_POINT('Ctrl Pts',(-19.382319769207,37.6004473925016,8.77934587282061));
#65390=CARTESIAN_POINT('Ctrl Pts',(-19.5044530062501,37.4744102397814,7.1848330982105));
#65391=CARTESIAN_POINT('Ctrl Pts',(-18.2309385662332,37.3483730870616,6.21759554364139));
#65392=CARTESIAN_POINT('Ctrl Pts',(-16.7276880664614,37.2223359343414,6.76314613761378));
#65393=CARTESIAN_POINT('Ctrl Pts',(-16.3709381367864,37.0962987816215,8.32202939309731));
#65394=CARTESIAN_POINT('Ctrl Pts',(-17.4872959006819,36.9702616289015,9.46707649195042));
#65395=CARTESIAN_POINT('Ctrl Pts',(-19.0547278059556,36.8442244761816,9.14998859182253));
#65396=CARTESIAN_POINT('Ctrl Pts',(-19.6382386864027,36.7181873234616,7.66106194033403));
#65397=CARTESIAN_POINT('Ctrl Pts',(-18.7036201365931,36.5921501707416,6.36341958655524));
#65398=CARTESIAN_POINT('Ctrl Pts',(-17.1065221583002,36.4661130180216,6.44506241609585));
#65399=CARTESIAN_POINT('Ctrl Pts',(-16.3090994097922,36.3400758653015,7.83124585186588));
#65400=CARTESIAN_POINT('Ctrl Pts',(-17.0413981697968,36.2140387125816,9.2529089624626));
#65401=CARTESIAN_POINT('Ctrl Pts',(-18.6329936143779,36.0880015598614,9.40850903678189));
#65402=CARTESIAN_POINT('Ctrl Pts',(-19.6267687797688,35.9619644071416,8.15559293383585));
#65403=CARTESIAN_POINT('Ctrl Pts',(-19.1129151695516,35.8359272544215,6.64121465399068));
#65404=CARTESIAN_POINT('Ctrl Pts',(-17.5618698412561,35.7098901017015,6.25179777628167));
#65405=CARTESIAN_POINT('Ctrl Pts',(-16.3936251655486,35.5838529489816,7.34385746899409));
#65406=CARTESIAN_POINT('Ctrl Pts',(-16.6777190612162,35.4578157962616,8.9176028151563));
#65407=CARTESIAN_POINT('Ctrl Pts',(-18.1540584911281,35.3317786435416,9.53226346517944));
#65408=CARTESIAN_POINT('Ctrl Pts',(-19.471050135726,35.2057414908216,8.6251036009875));
#65409=CARTESIAN_POINT('Ctrl Pts',(-19.4229666935522,35.0797043381016,7.02665363221171));
#65410=CARTESIAN_POINT('Ctrl Pts',(-18.0538527359272,34.9536671853816,6.2002681450112));
#65411=CARTESIAN_POINT('Ctrl Pts',(-16.6170945493887,34.8276300326616,6.90258420567117));
#65412=CARTESIAN_POINT('Ctrl Pts',(-16.4281487418217,34.7015928799416,8.49047690834462));
#65413=CARTESIAN_POINT('Ctrl Pts',(-17.6598093762981,34.5755557272216,9.51051625508399));
#65414=CARTESIAN_POINT('Ctrl Pts',(-19.1848544073993,34.4495185745016,9.02825816664846));
#65415=CARTESIAN_POINT('Ctrl Pts',(-19.6063538153946,34.3234814217816,7.48638804046807));
#65416=CARTESIAN_POINT('Ctrl Pts',(-18.5399022278055,34.1974442690615,6.29415834550658));
#65417=CARTESIAN_POINT('Ctrl Pts',(-16.9586559591529,34.071395908747,6.54781143533374));
#65418=CARTESIAN_POINT('Ctrl Pts',(-16.5316691371024,33.9873599326724,7.51933613284737));
#65419=CARTESIAN_POINT('Ctrl Pts',(-16.5709517952873,33.9453363408379,7.98805925999848));
#65420=CARTESIAN_POINT('Ctrl Pts',(-18.7079916422033,41.5491754829709,9.25003219459753));
#65421=CARTESIAN_POINT('Ctrl Pts',(-19.1669387919087,41.5071630987309,9.00792937228188));
#65422=CARTESIAN_POINT('Ctrl Pts',(-19.8162229296688,41.4231383302509,8.03368166911634));
#65423=CARTESIAN_POINT('Ctrl Pts',(-19.1123932777587,41.2971011775309,6.41291587346004));
#65424=CARTESIAN_POINT('Ctrl Pts',(-17.3701299623446,41.1710640248109,6.12991741636527));
#65425=CARTESIAN_POINT('Ctrl Pts',(-16.1870696686658,41.0450268720909,7.4381322882717));
#65426=CARTESIAN_POINT('Ctrl Pts',(-16.6450160912875,40.9189897193709,9.14264781598064));
#65427=CARTESIAN_POINT('Ctrl Pts',(-18.325368146149,40.7929525666509,9.68158136871029));
#65428=CARTESIAN_POINT('Ctrl Pts',(-19.6894233694515,40.6669154139309,8.56223244767046));
#65429=CARTESIAN_POINT('Ctrl Pts',(-19.488544466351,40.5408782612109,6.80902238783358));
#65430=CARTESIAN_POINT('Ctrl Pts',(-17.906554474218,40.4148411084909,6.02720399653423));
#65431=CARTESIAN_POINT('Ctrl Pts',(-16.3918183718805,40.2888039557709,6.93244887794637));
#65432=CARTESIAN_POINT('Ctrl Pts',(-16.3310669226111,40.1627668030509,8.69604349028723));
#65433=CARTESIAN_POINT('Ctrl Pts',(-17.7799290889218,40.0367296503309,9.7033818354433));
#65434=CARTESIAN_POINT('Ctrl Pts',(-19.4119558307657,39.9106924976109,9.03224972404705));
#65435=CARTESIAN_POINT('Ctrl Pts',(-19.7330176199543,39.784655344891,7.29706773910144));
#65436=CARTESIAN_POINT('Ctrl Pts',(-18.449178735851,39.6586181921709,6.08641031165167));
#65437=CARTESIAN_POINT('Ctrl Pts',(-16.7358035758118,39.5325810394509,6.50864157334445));
#65438=CARTESIAN_POINT('Ctrl Pts',(-16.1614990648281,39.4065438867309,8.177206495299));
#65439=CARTESIAN_POINT('Ctrl Pts',(-17.2520452792698,39.2805067340109,9.56452154229811));
#65440=CARTESIAN_POINT('Ctrl Pts',(-19.009039240403,39.1544695812909,9.40049000728872));
#65441=CARTESIAN_POINT('Ctrl Pts',(-19.8239404001145,39.028432428571,7.8352838465818));
#65442=CARTESIAN_POINT('Ctrl Pts',(-18.9507008716018,38.9023952758509,6.3018605892119));
#65443=CARTESIAN_POINT('Ctrl Pts',(-17.1887777264871,38.776358123131,6.20408021820285));
#65444=CARTESIAN_POINT('Ctrl Pts',(-16.1512242540963,38.6503209704109,7.63146137728754));
#65445=CARTESIAN_POINT('Ctrl Pts',(-16.7879281136981,38.524283817691,9.27722635685827));
#65446=CARTESIAN_POINT('Ctrl Pts',(-18.5159823471268,38.3982466649709,9.63466549992755));
#65447=CARTESIAN_POINT('Ctrl Pts',(-19.7533408921551,38.272209512251,8.37654070211551));
#65448=CARTESIAN_POINT('Ctrl Pts',(-19.3671931127862,38.146172359531,6.65467425339943));
#65449=CARTESIAN_POINT('Ctrl Pts',(-17.7110600748227,38.0201352068109,6.04544725498344));
#65450=CARTESIAN_POINT('Ctrl Pts',(-16.3011434700655,37.894098054091,7.10661140004615));
#65451=CARTESIAN_POINT('Ctrl Pts',(-16.4282320773269,37.768060901371,8.86666329158789));
#65452=CARTESIAN_POINT('Ctrl Pts',(-17.9759753637945,37.642023748651,9.71426278088));
#65453=CARTESIAN_POINT('Ctrl Pts',(-19.5274032336106,37.515986595931,8.87342644735645));
#65454=CARTESIAN_POINT('Ctrl Pts',(-19.6621723284219,37.389949443211,7.11394599386444));
#65455=CARTESIAN_POINT('Ctrl Pts',(-18.2569005738588,37.263912290491,6.0466384136139));
#65456=CARTESIAN_POINT('Ctrl Pts',(-16.5981243550872,37.137875137771,6.6486314623808));
#65457=CARTESIAN_POINT('Ctrl Pts',(-16.2044652147889,37.011837985051,8.36879618038998));
#65458=CARTESIAN_POINT('Ctrl Pts',(-17.4363209239151,36.885800832331,9.63230941204306));
#65459=CARTESIAN_POINT('Ctrl Pts',(-19.1659187317365,36.759763679611,9.28241571962643));
#65460=CARTESIAN_POINT('Ctrl Pts',(-19.8097994236285,36.633726526891,7.63944528897695));
#65461=CARTESIAN_POINT('Ctrl Pts',(-18.7784855978342,36.507689374171,6.20754935596669));
#65462=CARTESIAN_POINT('Ctrl Pts',(-17.0161524764798,36.381652221451,6.29763892127583));
#65463=CARTESIAN_POINT('Ctrl Pts',(-16.1362286768648,36.255615068731,7.82723636259333));
#65464=CARTESIAN_POINT('Ctrl Pts',(-16.9442907851535,36.129577916011,9.39598419226011));
#65465=CARTESIAN_POINT('Ctrl Pts',(-18.7005520827727,36.003540763291,9.56768259047058));
#65466=CARTESIAN_POINT('Ctrl Pts',(-19.797142844862,35.877503610571,8.18514026901571));
#65467=CARTESIAN_POINT('Ctrl Pts',(-19.2301261376084,35.751466457851,6.51408499432096));
#65468=CARTESIAN_POINT('Ctrl Pts',(-17.518610255722,35.625429305131,6.08437919609904));
#65469=CARTESIAN_POINT('Ctrl Pts',(-16.2294994348282,35.499392152411,7.28942296493543));
#65470=CARTESIAN_POINT('Ctrl Pts',(-16.5429855757627,35.373354999691,9.02598739981334));
#65471=CARTESIAN_POINT('Ctrl Pts',(-18.1720665157287,35.247317846971,9.70424060447069));
#65472=CARTESIAN_POINT('Ctrl Pts',(-19.6253136097501,35.121280694251,8.70322632935556));
#65473=CARTESIAN_POINT('Ctrl Pts',(-19.5722554731277,34.995243541531,6.93940134110259));
#65474=CARTESIAN_POINT('Ctrl Pts',(-18.0614935116043,34.869206388811,6.02751832898042));
#65475=CARTESIAN_POINT('Ctrl Pts',(-16.4760888752399,34.7431692360911,6.80249573937267));
#65476=CARTESIAN_POINT('Ctrl Pts',(-16.2675948070349,34.617132083371,8.55467121082956));
#65477=CARTESIAN_POINT('Ctrl Pts',(-17.6266825774209,34.491094930651,9.68024343637631));
#65478=CARTESIAN_POINT('Ctrl Pts',(-19.3095081813571,34.3650577779311,9.14809111144546));
#65479=CARTESIAN_POINT('Ctrl Pts',(-19.7746157561195,34.239020625211,7.44669969455893));
#65480=CARTESIAN_POINT('Ctrl Pts',(-18.597829497121,34.1129834724911,6.13112237353658));
#65481=CARTESIAN_POINT('Ctrl Pts',(-16.8529880971946,33.9869351121764,6.41101831455709));
#65482=CARTESIAN_POINT('Ctrl Pts',(-16.3818253826279,33.902899136102,7.48305658391363));
#65483=CARTESIAN_POINT('Ctrl Pts',(-16.4251722095321,33.8608755442674,8.00027362566716));
#65484=CARTESIAN_POINT('Ctrl Pts',(-18.7762476385807,41.4647146864003,9.37942306533622));
#65485=CARTESIAN_POINT('Ctrl Pts',(-19.2782253578306,41.4227023021603,9.11462084868009));
#65486=CARTESIAN_POINT('Ctrl Pts',(-19.9883859304091,41.3386775336803,8.04902834999368));
#65487=CARTESIAN_POINT('Ctrl Pts',(-19.2185656937367,41.2126403809603,6.27630066650286));
#65488=CARTESIAN_POINT('Ctrl Pts',(-17.3129489664818,41.0866032282403,5.96676846843845));
#65489=CARTESIAN_POINT('Ctrl Pts',(-16.0189657522113,40.9605660755203,7.39764066823327));
#65490=CARTESIAN_POINT('Ctrl Pts',(-16.5198489168936,40.8345289228003,9.26197040113339));
#65491=CARTESIAN_POINT('Ctrl Pts',(-18.357749626328,40.7084917700804,9.85143399361934));
#65492=CARTESIAN_POINT('Ctrl Pts',(-19.8496977305136,40.5824546173603,8.62713568652844));
#65493=CARTESIAN_POINT('Ctrl Pts',(-19.6299845594252,40.4564174646403,6.70954585561218));
#65494=CARTESIAN_POINT('Ctrl Pts',(-17.8996682721641,40.3303803119205,5.85442470890919));
#65495=CARTESIAN_POINT('Ctrl Pts',(-16.2429115532149,40.2043431592003,6.84454472866676));
#65496=CARTESIAN_POINT('Ctrl Pts',(-16.176464089787,40.0783060064804,8.7734927605975));
#65497=CARTESIAN_POINT('Ctrl Pts',(-17.7611705777108,39.9522688537603,9.87527845714036));
#65498=CARTESIAN_POINT('Ctrl Pts',(-19.5462150259696,39.8262317010404,9.14122145992317));
#65499=CARTESIAN_POINT('Ctrl Pts',(-19.8973793480026,39.7001945483203,7.24335000381806));
#65500=CARTESIAN_POINT('Ctrl Pts',(-18.4931686118854,39.5741573956004,5.91918216746824));
#65501=CARTESIAN_POINT('Ctrl Pts',(-16.6191485736127,39.4481202428803,6.3810015422626));
#65502=CARTESIAN_POINT('Ctrl Pts',(-15.99099766612,39.3220830901604,8.20600996530419));
#65503=CARTESIAN_POINT('Ctrl Pts',(-17.1837927446244,39.1960459374403,9.7233987182812));
#65504=CARTESIAN_POINT('Ctrl Pts',(-19.1055212528237,39.0700087847204,9.54398769920866));
#65505=CARTESIAN_POINT('Ctrl Pts',(-19.9968269855834,38.9439716320003,7.8320288838809));
#65506=CARTESIAN_POINT('Ctrl Pts',(-19.0417131186312,38.8179344792804,6.15483291507804));
#65507=CARTESIAN_POINT('Ctrl Pts',(-17.1145932695458,38.6918973265603,6.04788472364022));
#65508=CARTESIAN_POINT('Ctrl Pts',(-15.979759496191,38.5658601738404,7.60909615985389));
#65509=CARTESIAN_POINT('Ctrl Pts',(-16.6761602723712,38.4398230211204,9.40916693357315));
#65510=CARTESIAN_POINT('Ctrl Pts',(-18.5662356838727,38.3137858684004,9.80011932520205));
#65511=CARTESIAN_POINT('Ctrl Pts',(-19.9196081162464,38.1877487156804,8.42403361044614));
#65512=CARTESIAN_POINT('Ctrl Pts',(-19.4972553862961,38.0617115629604,6.54072614610208));
#65513=CARTESIAN_POINT('Ctrl Pts',(-17.6858444521501,37.9356744102404,5.87437844274086));
#65514=CARTESIAN_POINT('Ctrl Pts',(-16.1437350348827,37.8096372575204,7.03503660922119));
#65515=CARTESIAN_POINT('Ctrl Pts',(-16.2827393826746,37.6836001048004,8.96010975728389));
#65516=CARTESIAN_POINT('Ctrl Pts',(-17.9755980166681,37.5575629520803,9.88717959254801));
#65517=CARTESIAN_POINT('Ctrl Pts',(-19.6724866980142,37.4315257993604,8.96750702189228));
#65518=CARTESIAN_POINT('Ctrl Pts',(-19.8198916505935,37.3054886466404,7.0430588895184));
#65519=CARTESIAN_POINT('Ctrl Pts',(-18.2828625814843,37.1794514939204,5.87568128358639));
#65520=CARTESIAN_POINT('Ctrl Pts',(-16.4685606437131,37.0534143412004,6.53411678714783));
#65521=CARTESIAN_POINT('Ctrl Pts',(-16.0379922927914,36.9273771884804,8.41556296768266));
#65522=CARTESIAN_POINT('Ctrl Pts',(-17.3853459471484,36.8013400357604,9.79754233213571));
#65523=CARTESIAN_POINT('Ctrl Pts',(-19.2771096575173,36.6753028830404,9.41484284743033));
#65524=CARTESIAN_POINT('Ctrl Pts',(-19.9813601608543,36.5492657303204,7.61782863761985));
#65525=CARTESIAN_POINT('Ctrl Pts',(-18.8533510590753,36.4232285776004,6.05167912537815));
#65526=CARTESIAN_POINT('Ctrl Pts',(-16.9257827946596,36.2971914248804,6.15021542645577));
#65527=CARTESIAN_POINT('Ctrl Pts',(-15.9633579439374,36.1711542721604,7.82322687332076));
#65528=CARTESIAN_POINT('Ctrl Pts',(-16.84718340051,36.0451171194404,9.53905942205762));
#65529=CARTESIAN_POINT('Ctrl Pts',(-18.7681105511675,35.9190799667204,9.72685614415925));
#65530=CARTESIAN_POINT('Ctrl Pts',(-19.9675169099553,35.7930428140004,8.21468760419558));
#65531=CARTESIAN_POINT('Ctrl Pts',(-19.3473371056652,35.6670056612804,6.38695533465123));
#65532=CARTESIAN_POINT('Ctrl Pts',(-17.4753506701879,35.5409685085604,5.91696061591641));
#65533=CARTESIAN_POINT('Ctrl Pts',(-16.0653737041077,35.4149313558404,7.23498846087677));
#65534=CARTESIAN_POINT('Ctrl Pts',(-16.4082520903093,35.2888942031204,9.13437198447035));
#65535=CARTESIAN_POINT('Ctrl Pts',(-18.1900745403292,35.1628570504005,9.87621774376195));
#65536=CARTESIAN_POINT('Ctrl Pts',(-19.7795770837743,35.0368198976804,8.78134905772361));
#65537=CARTESIAN_POINT('Ctrl Pts',(-19.7215442527032,34.9107827449605,6.8521490499935));
#65538=CARTESIAN_POINT('Ctrl Pts',(-18.0691342872814,34.7847455922404,5.85476851294963));
#65539=CARTESIAN_POINT('Ctrl Pts',(-16.335083201091,34.6587084395204,6.70240727307417));
#65540=CARTESIAN_POINT('Ctrl Pts',(-16.1070408722481,34.5326712868005,8.61886551331448));
#65541=CARTESIAN_POINT('Ctrl Pts',(-17.5935557785435,34.4066341340805,9.84997061766864));
#65542=CARTESIAN_POINT('Ctrl Pts',(-19.4341619553151,34.2805969813605,9.26792405624247));
#65543=CARTESIAN_POINT('Ctrl Pts',(-19.9428776968442,34.1545598286405,7.40701134864978));
#65544=CARTESIAN_POINT('Ctrl Pts',(-18.6557567664365,34.0285226759205,5.96808640156658));
#65545=CARTESIAN_POINT('Ctrl Pts',(-16.7473202352362,33.902474315606,6.27422519378043));
#65546=CARTESIAN_POINT('Ctrl Pts',(-16.2319816281533,33.8184383395314,7.44677703497991));
#65547=CARTESIAN_POINT('Ctrl Pts',(-16.2793926237768,33.7764147476968,8.01248799133582));
#65548=CARTESIAN_POINT('Ctrl Pts',(-18.5338892852531,34.0285,6.25817448361128));
#65549=CARTESIAN_POINT('Ctrl Pts',(-18.5264711357089,34.0285,6.25568229473227));
#65550=CARTESIAN_POINT('Ctrl Pts',(-18.5190529861647,34.0285,6.25319010585325));
#65551=CARTESIAN_POINT('Ctrl Pts',(-18.5116348366204,34.0285,6.25069791697424));
#65552=CARTESIAN_POINT('Ctrl Pts',(-18.7711332099614,41.4659999999999,6.8735740585268));
#65553=CARTESIAN_POINT('Ctrl Pts',(-18.8150325114478,41.466,6.89761174551022));
#65554=CARTESIAN_POINT('Ctrl Pts',(-18.8572623534118,41.466,6.92446099914179));
#65555=CARTESIAN_POINT('Ctrl Pts',(-18.8977382984637,41.466,6.95381227460289));
#65556=CARTESIAN_POINT('Ctrl Pts',(-18.9281859213735,41.466,6.97589147660826));
#65557=CARTESIAN_POINT('Ctrl Pts',(-18.9576411714496,41.466,6.99938767928607));
#65558=CARTESIAN_POINT('Ctrl Pts',(-18.9860655235891,41.466,7.02418759153614));
#65559=CARTESIAN_POINT('Ctrl Pts',(-18.9960253921561,41.466,7.03287745948003));
#65560=CARTESIAN_POINT('Ctrl Pts',(-19.0058600905433,41.466,7.04172886589521));
#65561=CARTESIAN_POINT('Ctrl Pts',(-19.0155632740424,41.466,7.05073310140044));
#65562=CARTESIAN_POINT('Ctrl Pts',(-19.0545719021686,41.466,7.08693182673792));
#65563=CARTESIAN_POINT('Ctrl Pts',(-19.0913713554988,41.466,7.12551658131604));
#65564=CARTESIAN_POINT('Ctrl Pts',(-19.1258640554372,41.466,7.16616277809746));
#65565=CARTESIAN_POINT('Ctrl Pts',(-19.1505598681049,41.466,7.19526432315358));
#65566=CARTESIAN_POINT('Ctrl Pts',(-19.1740730954751,41.466,7.22542383308934));
#65567=CARTESIAN_POINT('Ctrl Pts',(-19.1963627498986,41.466,7.25653761332732));
#65568=CARTESIAN_POINT('Ctrl Pts',(-19.2034400634619,41.466,7.26641672471689));
#65569=CARTESIAN_POINT('Ctrl Pts',(-19.2103950492517,41.466,7.27639371368076));
#65570=CARTESIAN_POINT('Ctrl Pts',(-19.2172228745623,41.466,7.28646048298054));
#65571=CARTESIAN_POINT('Ctrl Pts',(-19.2487206908539,41.466,7.33290004984561));
#65572=CARTESIAN_POINT('Ctrl Pts',(-19.2774226769727,41.466,7.38110989018601));
#65573=CARTESIAN_POINT('Ctrl Pts',(-19.3032305569381,41.466,7.43074160061262));
#65574=CARTESIAN_POINT('Ctrl Pts',(-19.3290384369034,41.466,7.48037331103924));
#65575=CARTESIAN_POINT('Ctrl Pts',(-19.351952988103,41.466,7.53142771228986));
#65576=CARTESIAN_POINT('Ctrl Pts',(-19.3718527099145,41.466,7.58360345354479));
#65577=CARTESIAN_POINT('Ctrl Pts',(-19.3845995020632,41.466,7.61702469105144));
#65578=CARTESIAN_POINT('Ctrl Pts',(-19.3961087909219,41.466,7.65090693892874));
#65579=CARTESIAN_POINT('Ctrl Pts',(-19.4063413847352,41.466,7.68517870375625));
#65580=CARTESIAN_POINT('Ctrl Pts',(-19.4152961833237,41.466,7.71517078170846));
#65581=CARTESIAN_POINT('Ctrl Pts',(-19.4232731813879,41.466,7.74546129662054));
#65582=CARTESIAN_POINT('Ctrl Pts',(-19.4302416374854,41.466,7.77600509182718));
#65583=CARTESIAN_POINT('Ctrl Pts',(-19.4323739776039,41.466,7.78535146051786));
#65584=CARTESIAN_POINT('Ctrl Pts',(-19.4344110319851,41.466,7.7947182361204));
#65585=CARTESIAN_POINT('Ctrl Pts',(-19.4363504761414,41.466,7.80409571244044));
#65586=CARTESIAN_POINT('Ctrl Pts',(-19.4483033966471,41.466,7.86188970905142));
#65587=CARTESIAN_POINT('Ctrl Pts',(-19.4565726897916,41.466,7.92017862831491));
#65588=CARTESIAN_POINT('Ctrl Pts',(-19.4610359660074,41.466,7.97862520969174));
#65589=CARTESIAN_POINT('Ctrl Pts',(-19.4615949525186,41.466,7.98594513546783));
#65590=CARTESIAN_POINT('Ctrl Pts',(-19.4620941934996,41.466,7.99326758225861));
#65591=CARTESIAN_POINT('Ctrl Pts',(-19.4625334064251,41.466,8.0005919263415));
#65592=CARTESIAN_POINT('Ctrl Pts',(-19.4659158586079,41.466,8.05699792486926));
#65593=CARTESIAN_POINT('Ctrl Pts',(-19.4657422592885,41.466,8.11351490517321));
#65594=CARTESIAN_POINT('Ctrl Pts',(-19.4622098192675,41.466,8.1699133343397));
#65595=CARTESIAN_POINT('Ctrl Pts',(-19.4602920504131,41.466,8.20053215596072));
#65596=CARTESIAN_POINT('Ctrl Pts',(-19.4573834243698,41.466,8.23111637650103));
#65597=CARTESIAN_POINT('Ctrl Pts',(-19.4535094695855,41.466,8.26163092984805));
#65598=CARTESIAN_POINT('Ctrl Pts',(-19.4507014550128,41.466,8.28374923407363));
#65599=CARTESIAN_POINT('Ctrl Pts',(-19.4473861691094,41.466,8.30583095869765));
#65600=CARTESIAN_POINT('Ctrl Pts',(-19.4435719785325,41.466,8.32786291427628));
#65601=CARTESIAN_POINT('Ctrl Pts',(-19.4409779138594,41.466,8.34284704170591));
#65602=CARTESIAN_POINT('Ctrl Pts',(-19.4381517046733,41.466,8.3578139735458));
#65603=CARTESIAN_POINT('Ctrl Pts',(-19.4351029448282,41.466,8.37272646495416));
#65604=CARTESIAN_POINT('Ctrl Pts',(-19.423146378304,41.466,8.43120998107918));
#65605=CARTESIAN_POINT('Ctrl Pts',(-19.407760050003,41.466,8.48893384781506));
#65606=CARTESIAN_POINT('Ctrl Pts',(-19.3891801125346,41.466,8.54564278007359));
#65607=CARTESIAN_POINT('Ctrl Pts',(-19.3701830601375,41.466,8.60362481361556));
#65608=CARTESIAN_POINT('Ctrl Pts',(-19.3478473647113,41.466,8.66054673865175));
#65609=CARTESIAN_POINT('Ctrl Pts',(-19.322371280564,41.466,8.7161471563606));
#65610=CARTESIAN_POINT('Ctrl Pts',(-19.2966429325138,41.466,8.77229812878943));
#65611=CARTESIAN_POINT('Ctrl Pts',(-19.2677115047853,41.466,8.82710235142388));
#65612=CARTESIAN_POINT('Ctrl Pts',(-19.2357284380611,41.466,8.88028714355455));
#65613=CARTESIAN_POINT('Ctrl Pts',(-19.2296907577689,41.466,8.8903272305188));
#65614=CARTESIAN_POINT('Ctrl Pts',(-19.2235441817892,41.466,8.90030956924581));
#65615=CARTESIAN_POINT('Ctrl Pts',(-19.2172895300246,41.466,8.91023226242081));
#65616=CARTESIAN_POINT('Ctrl Pts',(-19.2108216298987,41.466,8.92049326348867));
#65617=CARTESIAN_POINT('Ctrl Pts',(-19.2042422248717,41.466,8.93068391788601));
#65618=CARTESIAN_POINT('Ctrl Pts',(-19.1975573996987,41.466,8.94079540529106));
#65619=CARTESIAN_POINT('Ctrl Pts',(-19.1621485581562,41.466,8.99435492944009));
#65620=CARTESIAN_POINT('Ctrl Pts',(-19.1237481043056,41.466,9.04575390697403));
#65621=CARTESIAN_POINT('Ctrl Pts',(-19.0825794977659,41.466,9.09471548562896));
#65622=CARTESIAN_POINT('Ctrl Pts',(-19.0413380622158,41.466,9.14376367939251));
#65623=CARTESIAN_POINT('Ctrl Pts',(-18.9973183329169,41.466,9.19036693480611));
#65624=CARTESIAN_POINT('Ctrl Pts',(-18.9506940483373,41.466,9.23423807965469));
#65625=CARTESIAN_POINT('Ctrl Pts',(-18.904483092379,41.466,9.27772030272191));
#65626=CARTESIAN_POINT('Ctrl Pts',(-18.8557131262279,41.466,9.31851969980534));
#65627=CARTESIAN_POINT('Ctrl Pts',(-18.8045092055452,41.466,9.35633200217432));
#65628=CARTESIAN_POINT('Ctrl Pts',(-18.7948293201577,41.466,9.36348025856348));
#65629=CARTESIAN_POINT('Ctrl Pts',(-18.7850623324094,41.466,9.37052166322747));
#65630=CARTESIAN_POINT('Ctrl Pts',(-18.7752089275578,41.466,9.3774540116144));
#65631=CARTESIAN_POINT('Origin',(-17.98,41.466,7.87));
#65632=CARTESIAN_POINT('',(-17.1642490230617,41.466,9.36643749592967));
#65633=CARTESIAN_POINT('',(-17.98,41.466,6.16566));
#65634=CARTESIAN_POINT('Origin',(-17.98,41.466,7.87));
#65635=CARTESIAN_POINT('Ctrl Pts',(-17.1642490230617,41.466,9.36643749592966));
#65636=CARTESIAN_POINT('Ctrl Pts',(-17.111789340126,41.466,9.32813761290297));
#65637=CARTESIAN_POINT('Ctrl Pts',(-17.0617472209979,41.466,9.28658023314859));
#65638=CARTESIAN_POINT('Ctrl Pts',(-17.0142916333355,41.466,9.24208960048121));
#65639=CARTESIAN_POINT('Ctrl Pts',(-16.9723635246812,41.466,9.20278109810107));
#65640=CARTESIAN_POINT('Ctrl Pts',(-16.9324549121243,41.466,9.16118180478115));
#65641=CARTESIAN_POINT('Ctrl Pts',(-16.8947136208791,41.466,9.11750245025616));
#65642=CARTESIAN_POINT('Ctrl Pts',(-16.8853938943848,41.466,9.10671639540251));
#65643=CARTESIAN_POINT('Ctrl Pts',(-16.8762127526669,41.466,9.09581071679169));
#65644=CARTESIAN_POINT('Ctrl Pts',(-16.8671731058919,41.466,9.0847902358313));
#65645=CARTESIAN_POINT('Ctrl Pts',(-16.8267762849462,41.466,9.03554136503217));
#65646=CARTESIAN_POINT('Ctrl Pts',(-16.7891936371374,41.466,8.98399208345677));
#65647=CARTESIAN_POINT('Ctrl Pts',(-16.754610798532,41.466,8.93044211916827));
#65648=CARTESIAN_POINT('Ctrl Pts',(-16.7315927675667,41.466,8.89479973740068));
#65649=CARTESIAN_POINT('Ctrl Pts',(-16.7099046708807,41.466,8.85827062428873));
#65650=CARTESIAN_POINT('Ctrl Pts',(-16.6896140741525,41.466,8.82094175216212));
#65651=CARTESIAN_POINT('Ctrl Pts',(-16.6821032533031,41.466,8.80712399831256));
#65652=CARTESIAN_POINT('Ctrl Pts',(-16.6747821860011,41.466,8.79319273006064));
#65653=CARTESIAN_POINT('Ctrl Pts',(-16.6676670453304,41.466,8.7791776958499));
#65654=CARTESIAN_POINT('Ctrl Pts',(-16.6397849483158,41.466,8.72425699060802));
#65655=CARTESIAN_POINT('Ctrl Pts',(-16.6150219263874,41.466,8.66798258419846));
#65656=CARTESIAN_POINT('Ctrl Pts',(-16.5935382103396,41.466,8.61063032490477));
#65657=CARTESIAN_POINT('Ctrl Pts',(-16.5726544678895,41.466,8.55487973644248));
#65658=CARTESIAN_POINT('Ctrl Pts',(-16.5548694058506,41.466,8.49810968578338));
#65659=CARTESIAN_POINT('Ctrl Pts',(-16.5403786854517,41.466,8.44057349599969));
#65660=CARTESIAN_POINT('Ctrl Pts',(-16.5315952966197,41.466,8.40569857516278));
#65661=CARTESIAN_POINT('Ctrl Pts',(-16.5240232072093,41.466,8.37054223600281));
#65662=CARTESIAN_POINT('Ctrl Pts',(-16.5177150916484,41.466,8.33516306780605));
#65663=CARTESIAN_POINT('Ctrl Pts',(-16.5124844857984,41.466,8.3058271302586));
#65664=CARTESIAN_POINT('Ctrl Pts',(-16.5081230458163,41.466,8.27633800030858));
#65665=CARTESIAN_POINT('Ctrl Pts',(-16.5046645357234,41.466,8.24673058741785));
#65666=CARTESIAN_POINT('Ctrl Pts',(-16.5031264715678,41.466,8.23356361687713));
#65667=CARTESIAN_POINT('Ctrl Pts',(-16.5017668817373,41.466,8.22037002113934));
#65668=CARTESIAN_POINT('Ctrl Pts',(-16.500590768404,41.466,8.20717809512951));
#65669=CARTESIAN_POINT('Ctrl Pts',(-16.4955380736504,41.466,8.15050432615207));
#65670=CARTESIAN_POINT('Ctrl Pts',(-16.4938551585946,41.466,8.09376815400606));
#65671=CARTESIAN_POINT('Ctrl Pts',(-16.4957110288904,41.466,8.03720028052094));
#65672=CARTESIAN_POINT('Ctrl Pts',(-16.4959467899537,41.466,8.03001416302452));
#65673=CARTESIAN_POINT('Ctrl Pts',(-16.4962397270978,41.466,8.02283077768763));
#65674=CARTESIAN_POINT('Ctrl Pts',(-16.4965902458921,41.466,8.01565061373279));
#65675=CARTESIAN_POINT('Ctrl Pts',(-16.499426906949,41.466,7.95754334016558));
#65676=CARTESIAN_POINT('Ctrl Pts',(-16.5060310991316,41.466,7.8996447512003));
#65677=CARTESIAN_POINT('Ctrl Pts',(-16.5162572633791,41.466,7.84225298758334));
#65678=CARTESIAN_POINT('Ctrl Pts',(-16.5251210845501,41.466,7.79250703034307));
#65679=CARTESIAN_POINT('Ctrl Pts',(-16.5367071997515,41.466,7.74314182037325));
#65680=CARTESIAN_POINT('Ctrl Pts',(-16.5509437230047,41.466,7.69437344281404));
#65681=CARTESIAN_POINT('Ctrl Pts',(-16.5537733871242,41.466,7.68468019638797));
#65682=CARTESIAN_POINT('Ctrl Pts',(-16.5567085247615,41.466,7.67500836402618));
#65683=CARTESIAN_POINT('Ctrl Pts',(-16.5597463211422,41.466,7.66536710704331));
#65684=CARTESIAN_POINT('Ctrl Pts',(-16.5766386373201,41.466,7.6117548365366));
#65685=CARTESIAN_POINT('Ctrl Pts',(-16.5966526679052,41.466,7.55923575103508));
#65686=CARTESIAN_POINT('Ctrl Pts',(-16.6196315985352,41.466,7.50807009544535));
#65687=CARTESIAN_POINT('Ctrl Pts',(-16.6424239719694,41.466,7.45731983434818));
#65688=CARTESIAN_POINT('Ctrl Pts',(-16.6681341614876,41.466,7.40790030018259));
#65689=CARTESIAN_POINT('Ctrl Pts',(-16.6966444927864,41.466,7.36010176185949));
#65690=CARTESIAN_POINT('Ctrl Pts',(-16.7244863815382,41.466,7.3134238901594));
#65691=CARTESIAN_POINT('Ctrl Pts',(-16.7549994631107,41.466,7.26829134122073));
#65692=CARTESIAN_POINT('Ctrl Pts',(-16.7880956091478,41.466,7.22501906714602));
#65693=CARTESIAN_POINT('Ctrl Pts',(-16.7942239191475,41.466,7.2170064752985));
#65694=CARTESIAN_POINT('Ctrl Pts',(-16.800440835444,41.466,7.20905780493933));
#65695=CARTESIAN_POINT('Ctrl Pts',(-16.8067458480612,41.466,7.201175251189));
#65696=CARTESIAN_POINT('Ctrl Pts',(-16.8135124330135,41.466,7.19271563773047));
#65697=CARTESIAN_POINT('Ctrl Pts',(-16.8203756788944,41.466,7.18433827145502));
#65698=CARTESIAN_POINT('Ctrl Pts',(-16.8273299671494,41.466,7.17605080146591));
#65699=CARTESIAN_POINT('Ctrl Pts',(-16.8612192200063,41.466,7.1356647611257));
#65700=CARTESIAN_POINT('Ctrl Pts',(-16.8973023839425,41.466,7.09736756612636));
#65701=CARTESIAN_POINT('Ctrl Pts',(-16.9354709299001,41.466,7.06141095674866));
#65702=CARTESIAN_POINT('Ctrl Pts',(-16.9728200232057,41.466,7.02622631125308));
#65703=CARTESIAN_POINT('Ctrl Pts',(-17.0121666768651,41.466,6.99328240785907));
#65704=CARTESIAN_POINT('Ctrl Pts',(-17.053425649955,41.466,6.96286170831185));
#65705=CARTESIAN_POINT('Ctrl Pts',(-17.0946846230449,41.466,6.93244100876463));
#65706=CARTESIAN_POINT('Ctrl Pts',(-17.1378565889557,41.466,6.90454300915782));
#65707=CARTESIAN_POINT('Ctrl Pts',(-17.1828623892565,41.466,6.87950438873575));
#65708=CARTESIAN_POINT('Ctrl Pts',(-17.1853034404496,41.466,6.87814632924464));
#65709=CARTESIAN_POINT('Ctrl Pts',(-17.187749886468,41.466,6.87679669586823));
#65710=CARTESIAN_POINT('Ctrl Pts',(-17.1902017145828,41.466,6.87545554732224));
#65711=CARTESIAN_POINT('Origin',(-17.98,41.466,7.87));
#65712=CARTESIAN_POINT('Ctrl Pts',(-16.919120712612,41.7180306875295,6.53336958898414));
#65713=CARTESIAN_POINT('Ctrl Pts',(-16.4744792903503,41.6760070959761,6.88626475233909));
#65714=CARTESIAN_POINT('Ctrl Pts',(-15.9731097926503,41.5919711201828,8.0647797895269));
#65715=CARTESIAN_POINT('Ctrl Pts',(-17.0570912447157,41.4659227601494,9.66491258748614));
#65716=CARTESIAN_POINT('Ctrl Pts',(-18.9869867646696,41.3398856074294,9.61721882671002));
#65717=CARTESIAN_POINT('Ctrl Pts',(-19.9944243161724,41.2138484547095,7.97209135863573));
#65718=CARTESIAN_POINT('Ctrl Pts',(-19.1579218343253,41.0878113019894,6.23241881161424));
#65719=CARTESIAN_POINT('Ctrl Pts',(-17.2428825517742,40.9617741492695,5.9925063653308));
#65720=CARTESIAN_POINT('Ctrl Pts',(-16.002750484554,40.8357369965494,7.47117978806733));
#65721=CARTESIAN_POINT('Ctrl Pts',(-16.5727688803051,40.7096998438294,9.31511334944695));
#65722=CARTESIAN_POINT('Ctrl Pts',(-18.4311354207765,40.5836626911095,9.83596614536317));
#65723=CARTESIAN_POINT('Ctrl Pts',(-19.8764752136172,40.4576255383895,8.55699758717004));
#65724=CARTESIAN_POINT('Ctrl Pts',(-19.5855828694099,40.3315883856694,6.64906030815352));
#65725=CARTESIAN_POINT('Ctrl Pts',(-17.8247655900277,40.2055512329495,5.85891088905231));
#65726=CARTESIAN_POINT('Ctrl Pts',(-16.2060676779772,40.0795140802294,6.90992356756758));
#65727=CARTESIAN_POINT('Ctrl Pts',(-16.2114169699092,39.9534769275095,8.83989534416103));
#65728=CARTESIAN_POINT('Ctrl Pts',(-17.8359170203282,39.8274397747895,9.88191984558327));
#65729=CARTESIAN_POINT('Ctrl Pts',(-19.5923259270914,39.7014026220695,9.08201784123309));
#65730=CARTESIAN_POINT('Ctrl Pts',(-19.8726389403143,39.5753654693495,7.17250451380341));
#65731=CARTESIAN_POINT('Ctrl Pts',(-18.4202273722028,39.4493283166295,5.90155345671652));
#65732=CARTESIAN_POINT('Ctrl Pts',(-16.564784501438,39.3232911639095,6.43272927708271));
#65733=CARTESIAN_POINT('Ctrl Pts',(-16.0049815753982,39.1972540111895,8.27973680401534));
#65734=CARTESIAN_POINT('Ctrl Pts',(-17.2533222079187,39.0712168584695,9.75162732564038));
#65735=CARTESIAN_POINT('Ctrl Pts',(-19.1669415762779,38.9451797057495,9.50087452448219));
#65736=CARTESIAN_POINT('Ctrl Pts',(-19.9939074072142,38.8191425530295,7.75704437735073));
#65737=CARTESIAN_POINT('Ctrl Pts',(-18.977126540798,38.6931054003095,6.11662591640547));
#65738=CARTESIAN_POINT('Ctrl Pts',(-17.047469164447,38.5670682475894,6.08143402191977));
#65739=CARTESIAN_POINT('Ctrl Pts',(-15.971550466053,38.4410310948696,7.68368712782179));
#65740=CARTESIAN_POINT('Ctrl Pts',(-16.7343817423075,38.3149939421494,9.45651100615227));
#65741=CARTESIAN_POINT('Ctrl Pts',(-18.6375854804388,38.1889567894296,9.77687266294394));
#65742=CARTESIAN_POINT('Ctrl Pts',(-19.9387649879574,38.0629196367095,8.35147870009828));
#65743=CARTESIAN_POINT('Ctrl Pts',(-19.4466810796223,37.9368824839895,6.48528752899183));
#65744=CARTESIAN_POINT('Ctrl Pts',(-17.6118401080523,37.8108453312696,5.88681057116351));
#65745=CARTESIAN_POINT('Ctrl Pts',(-16.1140521619751,37.6848081785495,7.10395778023238));
#65746=CARTESIAN_POINT('Ctrl Pts',(-16.3245528642827,37.5587710258296,9.0224221438397));
#65747=CARTESIAN_POINT('Ctrl Pts',(-18.0506273100736,37.4327338731095,9.885835757102));
#65748=CARTESIAN_POINT('Ctrl Pts',(-19.7120419461359,37.3066967203895,8.90373725558146));
#65749=CARTESIAN_POINT('Ctrl Pts',(-19.7877597397529,37.1806595676696,6.97524487118986));
#65750=CARTESIAN_POINT('Ctrl Pts',(-18.2084605066696,37.0546224149495,5.86590723461282));
#65751=CARTESIAN_POINT('Ctrl Pts',(-16.4200040391922,36.9285852622296,6.59133091857842));
#65752=CARTESIAN_POINT('Ctrl Pts',(-16.0597350780566,36.8025481095095,8.48738533320445));
#65753=CARTESIAN_POINT('Ctrl Pts',(-17.4574824475422,36.6765109567896,9.81821903631862));
#65754=CARTESIAN_POINT('Ctrl Pts',(-19.3335983859541,36.5504738040695,9.36544422685155));
#65755=CARTESIAN_POINT('Ctrl Pts',(-19.9704852863384,36.4244366513495,7.54357946878979));
#65756=CARTESIAN_POINT('Ctrl Pts',(-18.7850685961396,36.2983994986295,6.02055508638104));
#65757=CARTESIAN_POINT('Ctrl Pts',(-16.8626058508363,36.1723623459096,6.19071073752218));
#65758=CARTESIAN_POINT('Ctrl Pts',(-15.9631254208457,36.0463251931896,7.89826790759811));
#65759=CARTESIAN_POINT('Ctrl Pts',(-16.9101082626336,35.9202880404696,9.57994533257586));
#65760=CARTESIAN_POINT('Ctrl Pts',(-18.8365844605054,35.7942508877495,9.69615606533807));
#65761=CARTESIAN_POINT('Ctrl Pts',(-19.9788518580036,35.6682137350296,8.14050672632103));
#65762=CARTESIAN_POINT('Ctrl Pts',(-19.2911551757379,35.5421765823096,6.33720867716853));
#65763=CARTESIAN_POINT('Ctrl Pts',(-17.4030881947443,35.4161394295896,5.9371878387631));
#65764=CARTESIAN_POINT('Ctrl Pts',(-16.0431847714053,35.2901022768696,7.30667887406427));
#65765=CARTESIAN_POINT('Ctrl Pts',(-16.456456247779,35.1640651241495,9.19187763717425));
#65766=CARTESIAN_POINT('Ctrl Pts',(-18.2645297627139,35.0380279714296,9.86692133823987));
#65767=CARTESIAN_POINT('Ctrl Pts',(-19.8121404918094,34.9119908187095,8.71370280670959));
#65768=CARTESIAN_POINT('Ctrl Pts',(-19.6823612553971,34.7859536659897,6.78820027878308));
#65769=CARTESIAN_POINT('Ctrl Pts',(-17.9941617887159,34.6599165132695,5.85283083503748));
#65770=CARTESIAN_POINT('Ctrl Pts',(-16.2927908841274,34.5338793605497,6.76471570606888));
#65771=CARTESIAN_POINT('Ctrl Pts',(-16.1364825910008,34.4078422078296,8.68745919491244));
#65772=CARTESIAN_POINT('Ctrl Pts',(-17.6671032609381,34.2818050551096,9.86388249352386));
#65773=CARTESIAN_POINT('Ctrl Pts',(-19.4859215301242,34.1557679023896,9.2106775978793));
#65774=CARTESIAN_POINT('Ctrl Pts',(-19.7759329669726,34.0717431339096,7.96347022487569));
#65775=CARTESIAN_POINT('Ctrl Pts',(-19.6250757346175,34.0297307496696,7.41637949582761));
#65776=CARTESIAN_POINT('Ctrl Pts',(-17.0100469219083,41.6335880900653,6.64792997106398));
#65777=CARTESIAN_POINT('Ctrl Pts',(-16.6035149806241,41.5915644985119,6.97057907356705));
#65778=CARTESIAN_POINT('Ctrl Pts',(-16.1451170334339,41.5075285227186,8.04808553588302));
#65779=CARTESIAN_POINT('Ctrl Pts',(-17.1361922278737,41.3814801626852,9.51107359794373));
#65780=CARTESIAN_POINT('Ctrl Pts',(-18.9006795943709,41.2554430099652,9.46746759053033));
#65781=CARTESIAN_POINT('Ctrl Pts',(-19.8217713393811,41.1294058572452,7.96334127712032));
#65782=CARTESIAN_POINT('Ctrl Pts',(-19.0569641018898,41.0033687045251,6.37277318712605));
#65783=CARTESIAN_POINT('Ctrl Pts',(-17.306059669256,40.8773315518052,6.15342323985913));
#65784=CARTESIAN_POINT('Ctrl Pts',(-16.1722172706527,40.7512943990851,7.50536200888441));
#65785=CARTESIAN_POINT('Ctrl Pts',(-16.69338033237,40.6252572463652,9.1912550741175));
#65786=CARTESIAN_POINT('Ctrl Pts',(-18.3924693499255,40.4992200936452,9.6674664382544));
#65787=CARTESIAN_POINT('Ctrl Pts',(-19.7139314593479,40.3731829409252,8.49811616009379));
#65788=CARTESIAN_POINT('Ctrl Pts',(-19.4479710169003,40.2471457882052,6.75370503001651));
#65789=CARTESIAN_POINT('Ctrl Pts',(-17.8380704745879,40.1211086354852,6.03127801091937));
#65790=CARTESIAN_POINT('Ctrl Pts',(-16.3581084836628,39.9950714827652,6.992210130868));
#65791=CARTESIAN_POINT('Ctrl Pts',(-16.3629992966297,39.8690343300452,8.75676721817435));
#65792=CARTESIAN_POINT('Ctrl Pts',(-17.8482661342392,39.7429971773252,9.70948152282443));
#65793=CARTESIAN_POINT('Ctrl Pts',(-19.4541361382593,39.6169600246052,8.97813779643167));
#65794=CARTESIAN_POINT('Ctrl Pts',(-19.7104239866857,39.4909228718852,7.23228569844436));
#65795=CARTESIAN_POINT('Ctrl Pts',(-18.3824962121559,39.3648857191652,6.07026575462908));
#65796=CARTESIAN_POINT('Ctrl Pts',(-16.6860802814116,39.2388485664453,6.55591537386204));
#65797=CARTESIAN_POINT('Ctrl Pts',(-16.1742571383903,39.1128114137252,8.24461894014414));
#65798=CARTESIAN_POINT('Ctrl Pts',(-17.3156045597369,38.9867742610053,9.59035615929501));
#65799=CARTESIAN_POINT('Ctrl Pts',(-19.065210776676,38.8607371082852,9.3610949660424));
#65800=CARTESIAN_POINT('Ctrl Pts',(-19.8212987338348,38.7346999555652,7.766725616968));
#65801=CARTESIAN_POINT('Ctrl Pts',(-18.8916644739812,38.6086628028452,6.26690470947348));
#65802=CARTESIAN_POINT('Ctrl Pts',(-17.1273948401923,38.4826256501252,6.23472905406568));
#65803=CARTESIAN_POINT('Ctrl Pts',(-16.1436913541404,38.3565884974052,7.69965569598187));
#65804=CARTESIAN_POINT('Ctrl Pts',(-16.8411416232371,38.2305513446852,9.32053377150254));
#65805=CARTESIAN_POINT('Ctrl Pts',(-18.5812249163903,38.1045141919653,9.61343776048767));
#65806=CARTESIAN_POINT('Ctrl Pts',(-19.770882480141,37.9784770392452,8.31021195695673));
#65807=CARTESIAN_POINT('Ctrl Pts',(-19.3209742698072,37.8524398865252,6.60396894491806));
#65808=CARTESIAN_POINT('Ctrl Pts',(-17.6433944835478,37.7264027338052,6.05678645741582));
#65809=CARTESIAN_POINT('Ctrl Pts',(-16.2739794653669,37.6003655810852,7.16961399204876));
#65810=CARTESIAN_POINT('Ctrl Pts',(-16.4664385005945,37.4743284283653,8.9236499477057));
#65811=CARTESIAN_POINT('Ctrl Pts',(-18.0445739601269,37.3482912756453,9.71306180804281));
#65812=CARTESIAN_POINT('Ctrl Pts',(-19.5635914952915,37.2222541229252,8.81513734494529));
#65813=CARTESIAN_POINT('Ctrl Pts',(-19.6328196420356,37.0962169702053,7.05193285358171));
#65814=CARTESIAN_POINT('Ctrl Pts',(-18.1888795344588,36.9701798174852,6.03767471127206));
#65815=CARTESIAN_POINT('Ctrl Pts',(-16.5537087131546,36.8441426647653,6.70092353095212));
#65816=CARTESIAN_POINT('Ctrl Pts',(-16.2243178088843,36.7181055120452,8.43447025729455));
#65817=CARTESIAN_POINT('Ctrl Pts',(-17.5022665628516,36.5920683593253,9.65124040457685));
#65818=CARTESIAN_POINT('Ctrl Pts',(-19.217583706803,36.4660312066053,9.23727217525425));
#65819=CARTESIAN_POINT('Ctrl Pts',(-19.7998840842051,36.3399940538853,7.57155643270289));
#65820=CARTESIAN_POINT('Ctrl Pts',(-18.7160674981441,36.2139569011653,6.17906795141363));
#65821=CARTESIAN_POINT('Ctrl Pts',(-16.9583758554741,36.0879197484453,6.33463984308984));
#65822=CARTESIAN_POINT('Ctrl Pts',(-16.1359884056251,35.9618825957253,7.89584511198585));
#65823=CARTESIAN_POINT('Ctrl Pts',(-17.0018069141132,35.8358454430053,9.43338874593749));
#65824=CARTESIAN_POINT('Ctrl Pts',(-18.7631680229694,35.7098082902853,9.53963924897777));
#65825=CARTESIAN_POINT('Ctrl Pts',(-19.807533570849,35.5837711375653,8.11732204215769));
#65826=CARTESIAN_POINT('Ctrl Pts',(-19.1787782339442,35.4577339848453,6.4685816865996));
#65827=CARTESIAN_POINT('Ctrl Pts',(-17.4525343515067,35.3316968321253,6.10284597272071));
#65828=CARTESIAN_POINT('Ctrl Pts',(-16.209186001646,35.2056596794053,7.3549601961777));
#65829=CARTESIAN_POINT('Ctrl Pts',(-16.5870366632261,35.0796225266853,9.07858169094301));
#65830=CARTESIAN_POINT('Ctrl Pts',(-18.2401431872918,34.9535853739653,9.69576851274171));
#65831=CARTESIAN_POINT('Ctrl Pts',(-19.655110760153,34.8275482212453,8.64139043441735));
#65832=CARTESIAN_POINT('Ctrl Pts',(-19.5364546874716,34.7015110685253,6.88091954386572));
#65833=CARTESIAN_POINT('Ctrl Pts',(-17.9929480052251,34.5754739158053,6.02571906827927));
#65834=CARTESIAN_POINT('Ctrl Pts',(-16.437398787232,34.4494367630853,6.8594477950413));
#65835=CARTESIAN_POINT('Ctrl Pts',(-16.2944874194151,34.3233996103653,8.61739611918706));
#65836=CARTESIAN_POINT('Ctrl Pts',(-17.6939211229911,34.1973624576453,9.69299012238081));
#65837=CARTESIAN_POINT('Ctrl Pts',(-19.3568514861902,34.0713253049253,9.0957703381064));
#65838=CARTESIAN_POINT('Ctrl Pts',(-19.6220065223918,33.9873005364453,7.95545904647767));
#65839=CARTESIAN_POINT('Ctrl Pts',(-19.4840790139423,33.9452881522053,7.45525855906674));
#65840=CARTESIAN_POINT('Ctrl Pts',(-17.1009731312045,41.549145492601,6.76249035314384));
#65841=CARTESIAN_POINT('Ctrl Pts',(-16.7325506708981,41.5071219010477,7.05489339479501));
#65842=CARTESIAN_POINT('Ctrl Pts',(-16.3171242742175,41.4230859252543,8.03139128223913));
#65843=CARTESIAN_POINT('Ctrl Pts',(-17.2152932110317,41.2970375652208,9.35723460840133));
#65844=CARTESIAN_POINT('Ctrl Pts',(-18.8143724240723,41.1710004125009,9.31771635435063));
#65845=CARTESIAN_POINT('Ctrl Pts',(-19.6491183625899,41.0449632597809,7.95459119560491));
#65846=CARTESIAN_POINT('Ctrl Pts',(-18.9560063694543,40.9189261070609,6.51312756263786));
#65847=CARTESIAN_POINT('Ctrl Pts',(-17.3692367867377,40.7928889543409,6.31434011438746));
#65848=CARTESIAN_POINT('Ctrl Pts',(-16.3416840567515,40.6668518016209,7.53954422970151));
#65849=CARTESIAN_POINT('Ctrl Pts',(-16.813991784435,40.5408146489009,9.06739679878805));
#65850=CARTESIAN_POINT('Ctrl Pts',(-18.3538032790746,40.4147774961809,9.49896673114564));
#65851=CARTESIAN_POINT('Ctrl Pts',(-19.5513877050788,40.2887403434609,8.43923473301753));
#65852=CARTESIAN_POINT('Ctrl Pts',(-19.3103591643909,40.1627031907409,6.8583497518795));
#65853=CARTESIAN_POINT('Ctrl Pts',(-17.8513753591482,40.0366660380209,6.20364513278643));
#65854=CARTESIAN_POINT('Ctrl Pts',(-16.5101492893484,39.9106288853009,7.07449669416841));
#65855=CARTESIAN_POINT('Ctrl Pts',(-16.5145816233501,39.7845917325809,8.6736390921877));
#65856=CARTESIAN_POINT('Ctrl Pts',(-17.8606152481501,39.6585545798609,9.53704320006559));
#65857=CARTESIAN_POINT('Ctrl Pts',(-19.3159463494272,39.5325174271409,8.87425775163027));
#65858=CARTESIAN_POINT('Ctrl Pts',(-19.548209033057,39.406480274421,7.2920668830853));
#65859=CARTESIAN_POINT('Ctrl Pts',(-18.344765052109,39.2804431217009,6.23897805254165));
#65860=CARTESIAN_POINT('Ctrl Pts',(-16.8073760613852,39.154405968981,6.67910147064134));
#65861=CARTESIAN_POINT('Ctrl Pts',(-16.3435327013825,39.0283688162609,8.20950107627294));
#65862=CARTESIAN_POINT('Ctrl Pts',(-17.377886911555,38.902331663541,9.42908499294963));
#65863=CARTESIAN_POINT('Ctrl Pts',(-18.9634799770742,38.7762945108209,9.22131540760264));
#65864=CARTESIAN_POINT('Ctrl Pts',(-19.6486900604556,38.6502573581009,7.77640685658525));
#65865=CARTESIAN_POINT('Ctrl Pts',(-18.8062024071642,38.524220205381,6.4171835025415));
#65866=CARTESIAN_POINT('Ctrl Pts',(-17.2073205159376,38.3981830526609,6.38802408621161));
#65867=CARTESIAN_POINT('Ctrl Pts',(-16.3158322422279,38.272145899941,7.71562426414195));
#65868=CARTESIAN_POINT('Ctrl Pts',(-16.9479015041667,38.1461087472209,9.1845565368528));
#65869=CARTESIAN_POINT('Ctrl Pts',(-18.5248643523418,38.020071594501,9.45000285803138));
#65870=CARTESIAN_POINT('Ctrl Pts',(-19.6029999723246,37.894034441781,8.26894521381518));
#65871=CARTESIAN_POINT('Ctrl Pts',(-19.1952674599919,37.7679972890609,6.72265036084428));
#65872=CARTESIAN_POINT('Ctrl Pts',(-17.6749488590434,37.641960136341,6.22676234366814));
#65873=CARTESIAN_POINT('Ctrl Pts',(-16.4339067687587,37.5159229836209,7.23527020386514));
#65874=CARTESIAN_POINT('Ctrl Pts',(-16.6083241369064,37.389885830901,8.82487775157168));
#65875=CARTESIAN_POINT('Ctrl Pts',(-18.0385206101803,37.2638486781809,9.54028785898363));
#65876=CARTESIAN_POINT('Ctrl Pts',(-19.4151410444472,37.137811525461,8.72653743430914));
#65877=CARTESIAN_POINT('Ctrl Pts',(-19.4778795443183,37.011774372741,7.12862083597354));
#65878=CARTESIAN_POINT('Ctrl Pts',(-18.169298562248,36.885737220021,6.20944218793131));
#65879=CARTESIAN_POINT('Ctrl Pts',(-16.687413387117,36.7597000673009,6.81051614332581));
#65880=CARTESIAN_POINT('Ctrl Pts',(-16.388900539712,36.633662914581,8.38155518138464));
#65881=CARTESIAN_POINT('Ctrl Pts',(-17.547050678161,36.507625761861,9.48426177283507));
#65882=CARTESIAN_POINT('Ctrl Pts',(-19.101569027652,36.381588609141,9.10910012365699));
#65883=CARTESIAN_POINT('Ctrl Pts',(-19.6292828820718,36.255551456421,7.59953339661598));
#65884=CARTESIAN_POINT('Ctrl Pts',(-18.6470664001486,36.129514303701,6.33758081644621));
#65885=CARTESIAN_POINT('Ctrl Pts',(-17.0541458601119,36.003477150981,6.47856894865749));
#65886=CARTESIAN_POINT('Ctrl Pts',(-16.3088513904044,35.877439998261,7.89342231637359));
#65887=CARTESIAN_POINT('Ctrl Pts',(-17.0935055655928,35.751402845541,9.28683215929911));
#65888=CARTESIAN_POINT('Ctrl Pts',(-18.6897515854333,35.625365692821,9.38312243261748));
#65889=CARTESIAN_POINT('Ctrl Pts',(-19.6362152836945,35.499328540101,8.09413735799435));
#65890=CARTESIAN_POINT('Ctrl Pts',(-19.0664012921504,35.373291387381,6.59995469603067));
#65891=CARTESIAN_POINT('Ctrl Pts',(-17.5019805082691,35.247254234661,6.2685041066783));
#65892=CARTESIAN_POINT('Ctrl Pts',(-16.3751872318868,35.121217081941,7.40324151829113));
#65893=CARTESIAN_POINT('Ctrl Pts',(-16.7176170786733,34.995179929221,8.96528574471179));
#65894=CARTESIAN_POINT('Ctrl Pts',(-18.2157566118698,34.869142776501,9.52461568724354));
#65895=CARTESIAN_POINT('Ctrl Pts',(-19.4980810284966,34.7431056237811,8.56907806212513));
#65896=CARTESIAN_POINT('Ctrl Pts',(-19.390548119546,34.617068471061,6.97363880894833));
#65897=CARTESIAN_POINT('Ctrl Pts',(-17.9917342217342,34.4910313183411,6.19860730152107));
#65898=CARTESIAN_POINT('Ctrl Pts',(-16.5820066903367,34.3649941656211,6.95417988401373));
#65899=CARTESIAN_POINT('Ctrl Pts',(-16.4524922478294,34.238957012901,8.5473330434617));
#65900=CARTESIAN_POINT('Ctrl Pts',(-17.7207389850441,34.112919860181,9.52209775123777));
#65901=CARTESIAN_POINT('Ctrl Pts',(-19.2277814422563,33.9868827074611,8.98086307833352));
#65902=CARTESIAN_POINT('Ctrl Pts',(-19.4680800778111,33.9028579389811,7.94744786807967));
#65903=CARTESIAN_POINT('Ctrl Pts',(-19.3430822932671,33.8608455547411,7.49413762230587));
#65904=CARTESIAN_POINT('Ctrl Pts',(-17.1918993405008,41.4647028951367,6.87705073522368));
#65905=CARTESIAN_POINT('Ctrl Pts',(-16.8615863611721,41.4226793035834,7.13920771602296));
#65906=CARTESIAN_POINT('Ctrl Pts',(-16.4891315150011,41.33864332779,8.01469702859525));
#65907=CARTESIAN_POINT('Ctrl Pts',(-17.2943941941897,41.2125949677566,9.20339561885893));
#65908=CARTESIAN_POINT('Ctrl Pts',(-18.7280652537737,41.0865578150366,9.16796511817092));
#65909=CARTESIAN_POINT('Ctrl Pts',(-19.4764653857986,40.9605206623167,7.9458411140895));
#65910=CARTESIAN_POINT('Ctrl Pts',(-18.8550486370188,40.8344835095965,6.65348193814967));
#65911=CARTESIAN_POINT('Ctrl Pts',(-17.4324139042195,40.7084463568767,6.47525698891578));
#65912=CARTESIAN_POINT('Ctrl Pts',(-16.5111508428501,40.5824092041566,7.57372645051859));
#65913=CARTESIAN_POINT('Ctrl Pts',(-16.9346032365001,40.4563720514366,8.94353852345861));
#65914=CARTESIAN_POINT('Ctrl Pts',(-18.3151372082236,40.3303348987166,9.33046702403687));
#65915=CARTESIAN_POINT('Ctrl Pts',(-19.3888439508095,40.2042977459966,8.38035330594127));
#65916=CARTESIAN_POINT('Ctrl Pts',(-19.1727473118813,40.0782605932766,6.96299447374249));
#65917=CARTESIAN_POINT('Ctrl Pts',(-17.8646802437086,39.9522234405567,6.37601225465347));
#65918=CARTESIAN_POINT('Ctrl Pts',(-16.6621900950339,39.8261862878366,7.15678325746883));
#65919=CARTESIAN_POINT('Ctrl Pts',(-16.6661639500706,39.7001491351166,8.59051096620103));
#65920=CARTESIAN_POINT('Ctrl Pts',(-17.872964362061,39.5741119823967,9.36460487730674));
#65921=CARTESIAN_POINT('Ctrl Pts',(-19.1777565605952,39.4480748296766,8.77037770682886));
#65922=CARTESIAN_POINT('Ctrl Pts',(-19.3859940794283,39.3220376769567,7.35184806772624));
#65923=CARTESIAN_POINT('Ctrl Pts',(-18.3070338920621,39.1960005242366,6.40769035045421));
#65924=CARTESIAN_POINT('Ctrl Pts',(-16.9286718413587,39.0699633715167,6.80228756742067));
#65925=CARTESIAN_POINT('Ctrl Pts',(-16.5128082643746,38.9439262187966,8.17438321240174));
#65926=CARTESIAN_POINT('Ctrl Pts',(-17.4401692633733,38.8178890660767,9.26781382660424));
#65927=CARTESIAN_POINT('Ctrl Pts',(-18.8617491774723,38.6918519133567,9.08153584916288));
#65928=CARTESIAN_POINT('Ctrl Pts',(-19.4760813870762,38.5658147606367,7.78608809620251));
#65929=CARTESIAN_POINT('Ctrl Pts',(-18.7207403403473,38.4397776079167,6.56746229560953));
#65930=CARTESIAN_POINT('Ctrl Pts',(-17.2872461916829,38.3137404551967,6.54131911835751));
#65931=CARTESIAN_POINT('Ctrl Pts',(-16.4879731303155,38.1877033024767,7.73159283230202));
#65932=CARTESIAN_POINT('Ctrl Pts',(-17.0546613850961,38.0616661497567,9.04857930220307));
#65933=CARTESIAN_POINT('Ctrl Pts',(-18.4685037882934,37.9356289970366,9.28656795557511));
#65934=CARTESIAN_POINT('Ctrl Pts',(-19.4351174645082,37.8095918443167,8.22767847067363));
#65935=CARTESIAN_POINT('Ctrl Pts',(-19.0695606501767,37.6835546915967,6.8413317767705));
#65936=CARTESIAN_POINT('Ctrl Pts',(-17.706503234539,37.5575175388767,6.39673822992046));
#65937=CARTESIAN_POINT('Ctrl Pts',(-16.5938340721504,37.4314803861567,7.30092641568153));
#65938=CARTESIAN_POINT('Ctrl Pts',(-16.7502097732182,37.3054432334367,8.72610555543768));
#65939=CARTESIAN_POINT('Ctrl Pts',(-18.0324672602335,37.1794060807167,9.36751390992444));
#65940=CARTESIAN_POINT('Ctrl Pts',(-19.2666905936027,37.0533689279967,8.63793752367297));
#65941=CARTESIAN_POINT('Ctrl Pts',(-19.3229394466011,36.9273317752767,7.20530881836537));
#65942=CARTESIAN_POINT('Ctrl Pts',(-18.1497175900372,36.8012946225567,6.38120966459056));
#65943=CARTESIAN_POINT('Ctrl Pts',(-16.8211180610794,36.6752574698367,6.9201087556995));
#65944=CARTESIAN_POINT('Ctrl Pts',(-16.5534832705398,36.5492203171167,8.32864010547475));
#65945=CARTESIAN_POINT('Ctrl Pts',(-17.5918347934705,36.4231831643967,9.31728314109329));
#65946=CARTESIAN_POINT('Ctrl Pts',(-18.9855543485009,36.2971460116767,8.98092807205971));
#65947=CARTESIAN_POINT('Ctrl Pts',(-19.4586816799386,36.1711088589567,7.62751036052907));
#65948=CARTESIAN_POINT('Ctrl Pts',(-18.5780653021531,36.0450717062367,6.49609368147881));
#65949=CARTESIAN_POINT('Ctrl Pts',(-17.1499158647496,35.9190345535167,6.62249805422515));
#65950=CARTESIAN_POINT('Ctrl Pts',(-16.4817143751837,35.7929974007967,7.89099952076132));
#65951=CARTESIAN_POINT('Ctrl Pts',(-17.1852042170723,35.6669602480767,9.14027557266074));
#65952=CARTESIAN_POINT('Ctrl Pts',(-18.6163351478973,35.5409230953567,9.22660561625718));
#65953=CARTESIAN_POINT('Ctrl Pts',(-19.46489699654,35.4148859426367,8.07095267383102));
#65954=CARTESIAN_POINT('Ctrl Pts',(-18.9540243503566,35.2888487899167,6.73132770546173));
#65955=CARTESIAN_POINT('Ctrl Pts',(-17.5514266650314,35.1628116371968,6.43416224063591));
#65956=CARTESIAN_POINT('Ctrl Pts',(-16.5411884621276,35.0367744844767,7.45152284040454));
#65957=CARTESIAN_POINT('Ctrl Pts',(-16.8481974941205,34.9107373317568,8.85198979848058));
#65958=CARTESIAN_POINT('Ctrl Pts',(-18.1913700364478,34.7847001790368,9.35346286174535));
#65959=CARTESIAN_POINT('Ctrl Pts',(-19.3410512968401,34.6586630263167,8.49676568983289));
#65960=CARTESIAN_POINT('Ctrl Pts',(-19.2446415516205,34.5326258735968,7.06635807403095));
#65961=CARTESIAN_POINT('Ctrl Pts',(-17.9905204382435,34.4065887208768,6.37149553476286));
#65962=CARTESIAN_POINT('Ctrl Pts',(-16.7266145934414,34.2805515681568,7.04891197298617));
#65963=CARTESIAN_POINT('Ctrl Pts',(-16.6104970762435,34.1545144154369,8.47726996773631));
#65964=CARTESIAN_POINT('Ctrl Pts',(-17.7475568470971,34.0284772627168,9.35120538009473));
#65965=CARTESIAN_POINT('Ctrl Pts',(-19.0987113983223,33.9024401099968,8.86595581856062));
#65966=CARTESIAN_POINT('Ctrl Pts',(-19.3141536332304,33.8184153415168,7.93943668968165));
#65967=CARTESIAN_POINT('Ctrl Pts',(-19.2020855725918,33.7764029572768,7.533016685545));
#65968=CARTESIAN_POINT('Ctrl Pts',(-17.1849388579978,41.466,9.37753196187617));
#65969=CARTESIAN_POINT('Ctrl Pts',(-17.1780422463525,41.466,9.37383380656067));
#65970=CARTESIAN_POINT('Ctrl Pts',(-17.1711456347071,41.466,9.37013565124517));
#65971=CARTESIAN_POINT('Ctrl Pts',(-17.1642490230617,41.466,9.36643749592967));
#65972=CARTESIAN_POINT('Origin',(-17.98,41.466,7.87));
#65973=CARTESIAN_POINT('',(-17.98,41.616,6.01566));
#65974=CARTESIAN_POINT('Origin',(-17.98,41.616,7.87));
#65975=CARTESIAN_POINT('Origin',(-17.98,41.466,6.01566));
#65976=CARTESIAN_POINT('Origin',(-17.98,41.616,7.87));
#65977=CARTESIAN_POINT('',(-20.8502,41.616,7.87));
#65978=CARTESIAN_POINT('Origin',(-17.98,41.616,7.87));
#65979=CARTESIAN_POINT('Origin',(-17.98,33.8535,7.87));
#65980=CARTESIAN_POINT('',(-19.33434,33.6785,7.87));
#65981=CARTESIAN_POINT('',(-19.50934,33.8535,7.87));
#65982=CARTESIAN_POINT('Origin',(-17.98,33.6785,7.87));
#65983=CARTESIAN_POINT('Origin',(-17.98,33.6785,7.87));
#65984=CARTESIAN_POINT('Origin',(-14.830178752974,45.1212,7.47706978764225));
#65985=CARTESIAN_POINT('',(-15.1458469071313,42.216,7.41654185840086));
#65986=CARTESIAN_POINT('',(-15.1458469071313,44.8212,7.41654185840086));
#65987=CARTESIAN_POINT('',(-15.1458469071313,41.616,7.41654185840086));
#65988=CARTESIAN_POINT('',(-15.2715817176658,42.216,7.39243278178041));
#65989=CARTESIAN_POINT('',(-14.830178752974,42.216,7.47706978764225));
#65990=CARTESIAN_POINT('',(-15.2715817176658,44.9412,7.39243278178041));
#65991=CARTESIAN_POINT('',(-15.2715817176658,45.1212,7.39243278178041));
#65992=CARTESIAN_POINT('Ctrl Pts',(-15.1458469071312,44.8212,7.41654185840086));
#65993=CARTESIAN_POINT('Ctrl Pts',(-15.2100565813885,44.8826581248803,7.404229946132));
#65994=CARTESIAN_POINT('Ctrl Pts',(-15.2715817176658,44.9412,7.39243278178041));
#65995=CARTESIAN_POINT('Origin',(-15.2715817176658,45.1212,7.39243278178041));
#65996=CARTESIAN_POINT('',(-15.1616754338717,44.8212,7.32677382246615));
#65997=CARTESIAN_POINT('',(-15.1616754338717,42.216,7.32677382246615));
#65998=CARTESIAN_POINT('',(-15.1616754338717,41.616,7.32677382246615));
#65999=CARTESIAN_POINT('Ctrl Pts',(-15.2715817176658,44.9412,7.39243278178041));
#66000=CARTESIAN_POINT('Ctrl Pts',(-15.2178018689555,44.8826581248802,7.36030423756528));
#66001=CARTESIAN_POINT('Ctrl Pts',(-15.1616754338717,44.8212,7.32677382246614));
#66002=CARTESIAN_POINT('',(-15.2715817176658,42.216,7.39243278178041));
#66003=CARTESIAN_POINT('Origin',(-15.0647720895333,42.216,7.35596666447035));
#66004=CARTESIAN_POINT('Origin',(-17.98,42.216,7.87));
#66005=CARTESIAN_POINT('Origin',(-17.98,44.9712,7.87));
#66006=CARTESIAN_POINT('',(-20.7302,44.9412,7.87));
#66007=CARTESIAN_POINT('',(-20.8498381190176,44.8212,7.91557642629242));
#66008=CARTESIAN_POINT('Ctrl Pts',(-20.7302,44.9412,7.87));
#66009=CARTESIAN_POINT('Ctrl Pts',(-20.7887418751198,44.8826581248802,7.8923016667123));
#66010=CARTESIAN_POINT('Ctrl Pts',(-20.8498381190176,44.8212,7.91557642629242));
#66011=CARTESIAN_POINT('',(-20.8141530928687,44.8212,8.32345814159914));
#66012=CARTESIAN_POINT('Origin',(-17.98,44.8212,7.87));
#66013=CARTESIAN_POINT('',(-20.6884182823342,44.9412,8.34756721821959));
#66014=CARTESIAN_POINT('Ctrl Pts',(-20.8141530928687,44.8212,8.32345814159914));
#66015=CARTESIAN_POINT('Ctrl Pts',(-20.7499434186116,44.8826581248802,8.33577005386797));
#66016=CARTESIAN_POINT('Ctrl Pts',(-20.6884182823342,44.9412,8.34756721821959));
#66017=CARTESIAN_POINT('',(-20.7983245661282,44.8212,8.41322617753386));
#66018=CARTESIAN_POINT('Ctrl Pts',(-20.6884182823342,44.9412,8.34756721821959));
#66019=CARTESIAN_POINT('Ctrl Pts',(-20.7421981310449,44.8826581248798,8.37969576243495));
#66020=CARTESIAN_POINT('Ctrl Pts',(-20.7983245661282,44.8212,8.41322617753386));
#66021=CARTESIAN_POINT('',(-20.6923537591437,44.8212,8.80871461331909));
#66022=CARTESIAN_POINT('Origin',(-17.98,44.8212,7.87));
#66023=CARTESIAN_POINT('',(-20.5643426456854,44.9412,8.81062379817425));
#66024=CARTESIAN_POINT('Ctrl Pts',(-20.6923537591437,44.8212,8.80871461331909));
#66025=CARTESIAN_POINT('Ctrl Pts',(-20.6269816329882,44.8826581248798,8.80968958705249));
#66026=CARTESIAN_POINT('Ctrl Pts',(-20.5643426456854,44.9412,8.81062379817425));
#66027=CARTESIAN_POINT('',(-20.6611776474381,44.8212,8.89437027625664));
#66028=CARTESIAN_POINT('Ctrl Pts',(-20.5643426456854,44.9412,8.81062379817425));
#66029=CARTESIAN_POINT('Ctrl Pts',(-20.6117263944973,44.8826581248799,8.85160301033426));
#66030=CARTESIAN_POINT('Ctrl Pts',(-20.6611776474381,44.8212,8.89437027625664));
#66031=CARTESIAN_POINT('',(-20.4881409289644,44.8212,9.26544871652585));
#66032=CARTESIAN_POINT('Origin',(-17.98,44.8212,7.87));
#66033=CARTESIAN_POINT('',(-20.361743065488,44.9412,9.2451));
#66034=CARTESIAN_POINT('Ctrl Pts',(-20.4881409289644,44.8212,9.26544871652586));
#66035=CARTESIAN_POINT('Ctrl Pts',(-20.423592649883,44.8826581248802,9.25505712764031));
#66036=CARTESIAN_POINT('Ctrl Pts',(-20.361743065488,44.9412,9.2451));
#66037=CARTESIAN_POINT('',(-20.442564502672,44.8212,9.34438940249174));
#66038=CARTESIAN_POINT('Ctrl Pts',(-20.361743065488,44.9412,9.2451));
#66039=CARTESIAN_POINT('Ctrl Pts',(-20.4012909831707,44.8826581248803,9.29368474747942));
#66040=CARTESIAN_POINT('Ctrl Pts',(-20.442564502672,44.8212,9.34438940249174));
#66041=CARTESIAN_POINT('',(-20.207719505839,44.8212,9.67978281661211));
#66042=CARTESIAN_POINT('Origin',(-17.98,44.8212,7.87));
#66043=CARTESIAN_POINT('',(-20.0867754274658,44.9412,9.63779448415992));
#66044=CARTESIAN_POINT('Ctrl Pts',(-20.207719505839,44.8212,9.67978281661211));
#66045=CARTESIAN_POINT('Ctrl Pts',(-20.1459563406293,44.8826581248801,9.65834040827754));
#66046=CARTESIAN_POINT('Ctrl Pts',(-20.0867754274658,44.9412,9.63779448415992));
#66047=CARTESIAN_POINT('',(-20.1491275816099,44.8212,9.74960995280916));
#66048=CARTESIAN_POINT('Ctrl Pts',(-20.0867754274658,44.9412,9.63779448415992));
#66049=CARTESIAN_POINT('Ctrl Pts',(-20.1172858705533,44.8826581248798,9.69250854399236));
#66050=CARTESIAN_POINT('Ctrl Pts',(-20.1491275816099,44.8212,9.74960995280916));
#66051=CARTESIAN_POINT('',(-19.8596099528092,44.8212,10.0391275816099));
#66052=CARTESIAN_POINT('Origin',(-17.98,44.8212,7.87));
#66053=CARTESIAN_POINT('',(-19.7477944841599,44.9412,9.97677542746581));
#66054=CARTESIAN_POINT('Ctrl Pts',(-19.8596099528092,44.8212,10.0391275816099));
#66055=CARTESIAN_POINT('Ctrl Pts',(-19.8025085439922,44.88265812488,10.0072858705532));
#66056=CARTESIAN_POINT('Ctrl Pts',(-19.7477944841599,44.9412,9.97677542746581));
#66057=CARTESIAN_POINT('',(-19.7897828166121,44.8212,10.097719505839));
#66058=CARTESIAN_POINT('Ctrl Pts',(-19.7477944841599,44.9412,9.97677542746581));
#66059=CARTESIAN_POINT('Ctrl Pts',(-19.7683404082775,44.88265812488,10.0359563406293));
#66060=CARTESIAN_POINT('Ctrl Pts',(-19.7897828166121,44.8212,10.097719505839));
#66061=CARTESIAN_POINT('',(-19.4543894024917,44.8212,10.332564502672));
#66062=CARTESIAN_POINT('Origin',(-17.98,44.8212,7.87));
#66063=CARTESIAN_POINT('',(-19.3551,44.9412,10.251743065488));
#66064=CARTESIAN_POINT('Ctrl Pts',(-19.4543894024917,44.8212,10.332564502672));
#66065=CARTESIAN_POINT('Ctrl Pts',(-19.4036847474795,44.8826581248802,10.2912909831707));
#66066=CARTESIAN_POINT('Ctrl Pts',(-19.3551,44.9412,10.251743065488));
#66067=CARTESIAN_POINT('',(-19.3754487165258,44.8212,10.3781409289644));
#66068=CARTESIAN_POINT('Ctrl Pts',(-19.3551,44.9412,10.251743065488));
#66069=CARTESIAN_POINT('Ctrl Pts',(-19.3650571276404,44.8826581248798,10.3135926498835));
#66070=CARTESIAN_POINT('Ctrl Pts',(-19.3754487165258,44.8212,10.3781409289644));
#66071=CARTESIAN_POINT('',(-19.0043702762566,44.8212,10.5511776474381));
#66072=CARTESIAN_POINT('Origin',(-17.98,44.8212,7.87));
#66073=CARTESIAN_POINT('',(-18.9206237981742,44.9412,10.4543426456854));
#66074=CARTESIAN_POINT('Ctrl Pts',(-19.0043702762566,44.8212,10.5511776474381));
#66075=CARTESIAN_POINT('Ctrl Pts',(-18.9616030103341,44.8826581248802,10.5017263944971));
#66076=CARTESIAN_POINT('Ctrl Pts',(-18.9206237981742,44.9412,10.4543426456854));
#66077=CARTESIAN_POINT('',(-18.9187146133191,44.8212,10.5823537591437));
#66078=CARTESIAN_POINT('Ctrl Pts',(-18.9206237981743,44.9412,10.4543426456854));
#66079=CARTESIAN_POINT('Ctrl Pts',(-18.9196895870525,44.8826581248799,10.5169816329881));
#66080=CARTESIAN_POINT('Ctrl Pts',(-18.9187146133191,44.8212,10.5823537591437));
#66081=CARTESIAN_POINT('',(-18.5232261775339,44.8212,10.6883245661282));
#66082=CARTESIAN_POINT('Origin',(-17.98,44.8212,7.87));
#66083=CARTESIAN_POINT('',(-18.4575672182196,44.9412,10.5784182823342));
#66084=CARTESIAN_POINT('Ctrl Pts',(-18.5232261775339,44.8212,10.6883245661282));
#66085=CARTESIAN_POINT('Ctrl Pts',(-18.4896957624347,44.8826581248802,10.6321981310445));
#66086=CARTESIAN_POINT('Ctrl Pts',(-18.4575672182196,44.9412,10.5784182823342));
#66087=CARTESIAN_POINT('',(-18.4334581415991,44.8212,10.7041530928687));
#66088=CARTESIAN_POINT('Ctrl Pts',(-18.4575672182196,44.9412,10.5784182823342));
#66089=CARTESIAN_POINT('Ctrl Pts',(-18.4457700538679,44.8826581248799,10.6399434186118));
#66090=CARTESIAN_POINT('Ctrl Pts',(-18.4334581415991,44.8212,10.7041530928687));
#66091=CARTESIAN_POINT('',(-18.0255764262924,44.8212,10.7398381190176));
#66092=CARTESIAN_POINT('Origin',(-17.98,44.8212,7.87));
#66093=CARTESIAN_POINT('',(-17.98,44.9412,10.6202));
#66094=CARTESIAN_POINT('Ctrl Pts',(-18.0255764262924,44.8212,10.7398381190176));
#66095=CARTESIAN_POINT('Ctrl Pts',(-18.0023016667124,44.88265812488,10.67874187512));
#66096=CARTESIAN_POINT('Ctrl Pts',(-17.98,44.9412,10.6202));
#66097=CARTESIAN_POINT('',(-17.9344235737076,44.8212,10.7398381190176));
#66098=CARTESIAN_POINT('Ctrl Pts',(-17.98,44.9412,10.6202));
#66099=CARTESIAN_POINT('Ctrl Pts',(-17.9576983332875,44.8826581248798,10.6787418751202));
#66100=CARTESIAN_POINT('Ctrl Pts',(-17.9344235737076,44.8212,10.7398381190176));
#66101=CARTESIAN_POINT('',(-17.5265418584009,44.8212,10.7041530928687));
#66102=CARTESIAN_POINT('Origin',(-17.98,44.8212,7.87));
#66103=CARTESIAN_POINT('',(-17.5024327817804,44.9412,10.5784182823342));
#66104=CARTESIAN_POINT('Ctrl Pts',(-17.5265418584009,44.8212,10.7041530928687));
#66105=CARTESIAN_POINT('Ctrl Pts',(-17.5142299461321,44.88265812488,10.6399434186118));
#66106=CARTESIAN_POINT('Ctrl Pts',(-17.5024327817804,44.9412,10.5784182823342));
#66107=CARTESIAN_POINT('',(-17.4367738224661,44.8212,10.6883245661282));
#66108=CARTESIAN_POINT('Ctrl Pts',(-17.5024327817804,44.9412,10.5784182823342));
#66109=CARTESIAN_POINT('Ctrl Pts',(-17.4703042375651,44.8826581248799,10.6321981310448));
#66110=CARTESIAN_POINT('Ctrl Pts',(-17.4367738224661,44.8212,10.6883245661282));
#66111=CARTESIAN_POINT('',(-17.0412853866809,44.8212,10.5823537591437));
#66112=CARTESIAN_POINT('Origin',(-17.98,44.8212,7.87));
#66113=CARTESIAN_POINT('',(-17.0393762018257,44.9412,10.4543426456854));
#66114=CARTESIAN_POINT('Ctrl Pts',(-17.0412853866809,44.8212,10.5823537591437));
#66115=CARTESIAN_POINT('Ctrl Pts',(-17.0403104129475,44.8826581248804,10.5169816329876));
#66116=CARTESIAN_POINT('Ctrl Pts',(-17.0393762018257,44.9412,10.4543426456854));
#66117=CARTESIAN_POINT('',(-16.9556297237434,44.8212,10.5511776474381));
#66118=CARTESIAN_POINT('Ctrl Pts',(-17.0393762018257,44.9412,10.4543426456854));
#66119=CARTESIAN_POINT('Ctrl Pts',(-16.9983969896657,44.8826581248799,10.5017263944974));
#66120=CARTESIAN_POINT('Ctrl Pts',(-16.9556297237434,44.8212,10.5511776474381));
#66121=CARTESIAN_POINT('',(-16.5845512834741,44.8212,10.3781409289644));
#66122=CARTESIAN_POINT('Origin',(-17.98,44.8212,7.87));
#66123=CARTESIAN_POINT('',(-16.6049,44.9412,10.251743065488));
#66124=CARTESIAN_POINT('Ctrl Pts',(-16.5845512834741,44.8212,10.3781409289644));
#66125=CARTESIAN_POINT('Ctrl Pts',(-16.5949428723596,44.8826581248797,10.3135926498836));
#66126=CARTESIAN_POINT('Ctrl Pts',(-16.6049,44.9412,10.251743065488));
#66127=CARTESIAN_POINT('',(-16.5056105975083,44.8212,10.332564502672));
#66128=CARTESIAN_POINT('Ctrl Pts',(-16.6049,44.9412,10.251743065488));
#66129=CARTESIAN_POINT('Ctrl Pts',(-16.5563152525203,44.88265812488,10.2912909831709));
#66130=CARTESIAN_POINT('Ctrl Pts',(-16.5056105975083,44.8212,10.332564502672));
#66131=CARTESIAN_POINT('',(-16.1702171833879,44.8212,10.097719505839));
#66132=CARTESIAN_POINT('Origin',(-17.98,44.8212,7.87));
#66133=CARTESIAN_POINT('',(-16.2122055158401,44.9412,9.97677542746581));
#66134=CARTESIAN_POINT('Ctrl Pts',(-16.1702171833879,44.8212,10.097719505839));
#66135=CARTESIAN_POINT('Ctrl Pts',(-16.1916595917225,44.8826581248802,10.0359563406291));
#66136=CARTESIAN_POINT('Ctrl Pts',(-16.2122055158401,44.9412,9.97677542746581));
#66137=CARTESIAN_POINT('',(-16.1003900471908,44.8212,10.0391275816099));
#66138=CARTESIAN_POINT('Ctrl Pts',(-16.2122055158401,44.9412,9.97677542746581));
#66139=CARTESIAN_POINT('Ctrl Pts',(-16.1574914560079,44.8826581248801,10.0072858705531));
#66140=CARTESIAN_POINT('Ctrl Pts',(-16.1003900471908,44.8212,10.0391275816099));
#66141=CARTESIAN_POINT('',(-15.8108724183901,44.8212,9.74960995280916));
#66142=CARTESIAN_POINT('Origin',(-17.98,44.8212,7.87));
#66143=CARTESIAN_POINT('',(-15.8732245725342,44.9412,9.63779448415992));
#66144=CARTESIAN_POINT('Ctrl Pts',(-15.8108724183901,44.8212,9.74960995280916));
#66145=CARTESIAN_POINT('Ctrl Pts',(-15.8427141294468,44.88265812488,9.69250854399223));
#66146=CARTESIAN_POINT('Ctrl Pts',(-15.8732245725342,44.9412,9.63779448415992));
#66147=CARTESIAN_POINT('',(-15.752280494161,44.8212,9.67978281661211));
#66148=CARTESIAN_POINT('Ctrl Pts',(-15.8732245725342,44.9412,9.63779448415992));
#66149=CARTESIAN_POINT('Ctrl Pts',(-15.8140436593705,44.8826581248799,9.65834040827761));
#66150=CARTESIAN_POINT('Ctrl Pts',(-15.752280494161,44.8212,9.67978281661211));
#66151=CARTESIAN_POINT('',(-15.517435497328,44.8212,9.34438940249174));
#66152=CARTESIAN_POINT('Origin',(-17.98,44.8212,7.87));
#66153=CARTESIAN_POINT('',(-15.598256934512,44.9412,9.2451));
#66154=CARTESIAN_POINT('Ctrl Pts',(-15.517435497328,44.8212,9.34438940249174));
#66155=CARTESIAN_POINT('Ctrl Pts',(-15.5587090168291,44.88265812488,9.29368474747968));
#66156=CARTESIAN_POINT('Ctrl Pts',(-15.598256934512,44.9412,9.2451));
#66157=CARTESIAN_POINT('',(-15.4718590710356,44.8212,9.26544871652585));
#66158=CARTESIAN_POINT('Ctrl Pts',(-15.598256934512,44.9412,9.2451));
#66159=CARTESIAN_POINT('Ctrl Pts',(-15.5364073501168,44.8826581248801,9.25505712764034));
#66160=CARTESIAN_POINT('Ctrl Pts',(-15.4718590710356,44.8212,9.26544871652585));
#66161=CARTESIAN_POINT('',(-15.2988223525619,44.8212,8.89437027625664));
#66162=CARTESIAN_POINT('Origin',(-17.98,44.8212,7.87));
#66163=CARTESIAN_POINT('',(-15.3956573543146,44.9412,8.81062379817425));
#66164=CARTESIAN_POINT('Ctrl Pts',(-15.2988223525619,44.8212,8.89437027625664));
#66165=CARTESIAN_POINT('Ctrl Pts',(-15.3482736055027,44.88265812488,8.85160301033418));
#66166=CARTESIAN_POINT('Ctrl Pts',(-15.3956573543146,44.9412,8.81062379817426));
#66167=CARTESIAN_POINT('',(-15.2676462408563,44.8212,8.80871461331909));
#66168=CARTESIAN_POINT('Ctrl Pts',(-15.3956573543146,44.9412,8.81062379817425));
#66169=CARTESIAN_POINT('Ctrl Pts',(-15.3330183670121,44.8826581248801,8.8096895870525));
#66170=CARTESIAN_POINT('Ctrl Pts',(-15.2676462408562,44.8212,8.80871461331909));
#66171=CARTESIAN_POINT('',(-15.1616754338717,44.8212,8.41322617753385));
#66172=CARTESIAN_POINT('Origin',(-17.98,44.8212,7.87));
#66173=CARTESIAN_POINT('',(-15.2715817176658,44.9412,8.34756721821959));
#66174=CARTESIAN_POINT('Ctrl Pts',(-15.1616754338717,44.8212,8.41322617753386));
#66175=CARTESIAN_POINT('Ctrl Pts',(-15.2178018689556,44.8826581248803,8.37969576243469));
#66176=CARTESIAN_POINT('Ctrl Pts',(-15.2715817176658,44.9412,8.34756721821959));
#66177=CARTESIAN_POINT('',(-15.1458469071313,44.8212,8.32345814159913));
#66178=CARTESIAN_POINT('Ctrl Pts',(-15.2715817176658,44.9412,8.34756721821959));
#66179=CARTESIAN_POINT('Ctrl Pts',(-15.2100565813884,44.8826581248802,8.33577005386797));
#66180=CARTESIAN_POINT('Ctrl Pts',(-15.1458469071312,44.8212,8.32345814159913));
#66181=CARTESIAN_POINT('',(-15.1101618809824,44.8212,7.91557642629241));
#66182=CARTESIAN_POINT('Origin',(-17.98,44.8212,7.87));
#66183=CARTESIAN_POINT('',(-15.2298,44.9412,7.87));
#66184=CARTESIAN_POINT('Ctrl Pts',(-15.1101618809824,44.8212,7.91557642629241));
#66185=CARTESIAN_POINT('Ctrl Pts',(-15.1712581248802,44.8826581248802,7.89230166671231));
#66186=CARTESIAN_POINT('Ctrl Pts',(-15.2298,44.9412,7.87));
#66187=CARTESIAN_POINT('',(-15.1101618809824,44.8212,7.82442357370758));
#66188=CARTESIAN_POINT('Ctrl Pts',(-15.2298,44.9412,7.87));
#66189=CARTESIAN_POINT('Ctrl Pts',(-15.1712581248802,44.8826581248802,7.8476983332877));
#66190=CARTESIAN_POINT('Ctrl Pts',(-15.1101618809824,44.8212,7.82442357370758));
#66191=CARTESIAN_POINT('Origin',(-17.98,44.8212,7.87));
#66192=CARTESIAN_POINT('',(-15.2676462408563,44.8212,6.93128538668091));
#66193=CARTESIAN_POINT('Origin',(-17.98,44.8212,7.87));
#66194=CARTESIAN_POINT('',(-15.3956573543146,44.9412,6.92937620182574));
#66195=CARTESIAN_POINT('Ctrl Pts',(-15.2676462408562,44.8212,6.93128538668091));
#66196=CARTESIAN_POINT('Ctrl Pts',(-15.3330183670122,44.8826581248802,6.93031041294749));
#66197=CARTESIAN_POINT('Ctrl Pts',(-15.3956573543146,44.9412,6.92937620182574));
#66198=CARTESIAN_POINT('',(-15.2988223525619,44.8212,6.84562972374336));
#66199=CARTESIAN_POINT('Ctrl Pts',(-15.3956573543146,44.9412,6.92937620182574));
#66200=CARTESIAN_POINT('Ctrl Pts',(-15.3482736055027,44.8826581248799,6.88839698966574));
#66201=CARTESIAN_POINT('Ctrl Pts',(-15.2988223525619,44.8212,6.84562972374336));
#66202=CARTESIAN_POINT('',(-15.4718590710356,44.8212,6.47455128347414));
#66203=CARTESIAN_POINT('Origin',(-17.98,44.8212,7.87));
#66204=CARTESIAN_POINT('',(-15.598256934512,44.9412,6.4949));
#66205=CARTESIAN_POINT('Ctrl Pts',(-15.4718590710356,44.8212,6.47455128347414));
#66206=CARTESIAN_POINT('Ctrl Pts',(-15.5364073501167,44.88265812488,6.48494287235965));
#66207=CARTESIAN_POINT('Ctrl Pts',(-15.598256934512,44.9412,6.4949));
#66208=CARTESIAN_POINT('',(-15.517435497328,44.8212,6.39561059750826));
#66209=CARTESIAN_POINT('Ctrl Pts',(-15.598256934512,44.9412,6.4949));
#66210=CARTESIAN_POINT('Ctrl Pts',(-15.5587090168292,44.8826581248801,6.44631525252043));
#66211=CARTESIAN_POINT('Ctrl Pts',(-15.517435497328,44.8212,6.39561059750826));
#66212=CARTESIAN_POINT('',(-15.752280494161,44.8212,6.0602171833879));
#66213=CARTESIAN_POINT('Origin',(-17.98,44.8212,7.87));
#66214=CARTESIAN_POINT('',(-15.8732245725342,44.9412,6.10220551584008));
#66215=CARTESIAN_POINT('Ctrl Pts',(-15.752280494161,44.8212,6.06021718338789));
#66216=CARTESIAN_POINT('Ctrl Pts',(-15.8140436593704,44.8826581248798,6.08165959172236));
#66217=CARTESIAN_POINT('Ctrl Pts',(-15.8732245725342,44.9412,6.10220551584008));
#66218=CARTESIAN_POINT('',(-15.8108724183901,44.8212,5.99039004719084));
#66219=CARTESIAN_POINT('Ctrl Pts',(-15.8732245725342,44.9412,6.10220551584008));
#66220=CARTESIAN_POINT('Ctrl Pts',(-15.8427141294467,44.8826581248798,6.04749145600765));
#66221=CARTESIAN_POINT('Ctrl Pts',(-15.8108724183901,44.8212,5.99039004719084));
#66222=CARTESIAN_POINT('',(-16.1003900471908,44.8212,5.70087241839011));
#66223=CARTESIAN_POINT('Origin',(-17.98,44.8212,7.87));
#66224=CARTESIAN_POINT('',(-16.2122055158401,44.9412,5.76322457253418));
#66225=CARTESIAN_POINT('Ctrl Pts',(-16.1003900471908,44.8212,5.70087241839011));
#66226=CARTESIAN_POINT('Ctrl Pts',(-16.1574914560079,44.8826581248801,5.73271412944688));
#66227=CARTESIAN_POINT('Ctrl Pts',(-16.2122055158401,44.9412,5.76322457253418));
#66228=CARTESIAN_POINT('',(-16.1702171833879,44.8212,5.642280494161));
#66229=CARTESIAN_POINT('Ctrl Pts',(-16.2122055158401,44.9412,5.76322457253418));
#66230=CARTESIAN_POINT('Ctrl Pts',(-16.1916595917224,44.88265812488,5.70404365937061));
#66231=CARTESIAN_POINT('Ctrl Pts',(-16.1702171833879,44.8212,5.64228049416099));
#66232=CARTESIAN_POINT('',(-16.5056105975083,44.8212,5.40743549732803));
#66233=CARTESIAN_POINT('Origin',(-17.98,44.8212,7.87));
#66234=CARTESIAN_POINT('',(-16.6049,44.9412,5.48825693451204));
#66235=CARTESIAN_POINT('Ctrl Pts',(-16.5056105975083,44.8212,5.40743549732802));
#66236=CARTESIAN_POINT('Ctrl Pts',(-16.5563152525204,44.8826581248801,5.44870901682921));
#66237=CARTESIAN_POINT('Ctrl Pts',(-16.6049,44.9412,5.48825693451204));
#66238=CARTESIAN_POINT('',(-16.5845512834741,44.8212,5.36185907103561));
#66239=CARTESIAN_POINT('Ctrl Pts',(-16.6049,44.9412,5.48825693451204));
#66240=CARTESIAN_POINT('Ctrl Pts',(-16.5949428723597,44.8826581248804,5.42640735011712));
#66241=CARTESIAN_POINT('Ctrl Pts',(-16.5845512834741,44.8212,5.36185907103561));
#66242=CARTESIAN_POINT('',(-16.9556297237434,44.8212,5.18882235256186));
#66243=CARTESIAN_POINT('Origin',(-17.98,44.8212,7.87));
#66244=CARTESIAN_POINT('',(-17.0393762018257,44.9412,5.28565735431459));
#66245=CARTESIAN_POINT('Ctrl Pts',(-16.9556297237434,44.8212,5.18882235256186));
#66246=CARTESIAN_POINT('Ctrl Pts',(-16.998396989666,44.8826581248802,5.23827360550292));
#66247=CARTESIAN_POINT('Ctrl Pts',(-17.0393762018257,44.9412,5.28565735431459));
#66248=CARTESIAN_POINT('',(-17.0412853866809,44.8212,5.15764624085626));
#66249=CARTESIAN_POINT('Ctrl Pts',(-17.0393762018257,44.9412,5.28565735431459));
#66250=CARTESIAN_POINT('Ctrl Pts',(-17.0403104129475,44.8826581248803,5.22301836701232));
#66251=CARTESIAN_POINT('Ctrl Pts',(-17.0412853866809,44.8212,5.15764624085625));
#66252=CARTESIAN_POINT('',(-17.4367738224661,44.8212,5.05167543387175));
#66253=CARTESIAN_POINT('Origin',(-17.98,44.8212,7.87));
#66254=CARTESIAN_POINT('',(-17.5024327817804,44.9412,5.16158171766583));
#66255=CARTESIAN_POINT('Ctrl Pts',(-17.4367738224661,44.8212,5.05167543387175));
#66256=CARTESIAN_POINT('Ctrl Pts',(-17.4703042375652,44.8826581248801,5.10780186895543));
#66257=CARTESIAN_POINT('Ctrl Pts',(-17.5024327817804,44.9412,5.16158171766583));
#66258=CARTESIAN_POINT('',(-17.5265418584009,44.8212,5.03584690713126));
#66259=CARTESIAN_POINT('Ctrl Pts',(-17.5024327817804,44.9412,5.16158171766583));
#66260=CARTESIAN_POINT('Ctrl Pts',(-17.514229946132,44.8826581248803,5.10005658138852));
#66261=CARTESIAN_POINT('Ctrl Pts',(-17.5265418584009,44.8212,5.03584690713125));
#66262=CARTESIAN_POINT('',(-17.9344235737076,44.8212,5.00016188098241));
#66263=CARTESIAN_POINT('Origin',(-17.98,44.8212,7.87));
#66264=CARTESIAN_POINT('',(-17.98,44.9412,5.1198));
#66265=CARTESIAN_POINT('Ctrl Pts',(-17.9344235737076,44.8212,5.00016188098241));
#66266=CARTESIAN_POINT('Ctrl Pts',(-17.9576983332877,44.8826581248802,5.06125812488014));
#66267=CARTESIAN_POINT('Ctrl Pts',(-17.98,44.9412,5.1198));
#66268=CARTESIAN_POINT('',(-18.0255764262924,44.8212,5.00016188098241));
#66269=CARTESIAN_POINT('Ctrl Pts',(-17.98,44.9412,5.1198));
#66270=CARTESIAN_POINT('Ctrl Pts',(-18.0023016667124,44.8826581248799,5.06125812487993));
#66271=CARTESIAN_POINT('Ctrl Pts',(-18.0255764262924,44.8212,5.00016188098241));
#66272=CARTESIAN_POINT('',(-18.4334581415991,44.8212,5.03584690713126));
#66273=CARTESIAN_POINT('Origin',(-17.98,44.8212,7.87));
#66274=CARTESIAN_POINT('',(-18.4575672182196,44.9412,5.16158171766583));
#66275=CARTESIAN_POINT('Ctrl Pts',(-18.4334581415991,44.8212,5.03584690713125));
#66276=CARTESIAN_POINT('Ctrl Pts',(-18.4457700538679,44.8826581248799,5.10005658138809));
#66277=CARTESIAN_POINT('Ctrl Pts',(-18.4575672182196,44.9412,5.16158171766583));
#66278=CARTESIAN_POINT('',(-18.5232261775339,44.8212,5.05167543387175));
#66279=CARTESIAN_POINT('Ctrl Pts',(-18.4575672182196,44.9412,5.16158171766583));
#66280=CARTESIAN_POINT('Ctrl Pts',(-18.4896957624347,44.8826581248803,5.10780186895555));
#66281=CARTESIAN_POINT('Ctrl Pts',(-18.5232261775339,44.8212,5.05167543387175));
#66282=CARTESIAN_POINT('',(-18.9187146133191,44.8212,5.15764624085626));
#66283=CARTESIAN_POINT('Origin',(-17.98,44.8212,7.87));
#66284=CARTESIAN_POINT('',(-18.9206237981743,44.9412,5.28565735431459));
#66285=CARTESIAN_POINT('Ctrl Pts',(-18.9187146133191,44.8212,5.15764624085625));
#66286=CARTESIAN_POINT('Ctrl Pts',(-18.9196895870525,44.8826581248801,5.22301836701204));
#66287=CARTESIAN_POINT('Ctrl Pts',(-18.9206237981743,44.9412,5.28565735431459));
#66288=CARTESIAN_POINT('',(-19.0043702762566,44.8212,5.18882235256187));
#66289=CARTESIAN_POINT('Ctrl Pts',(-18.9206237981743,44.9412,5.28565735431459));
#66290=CARTESIAN_POINT('Ctrl Pts',(-18.9616030103343,44.8826581248799,5.23827360550266));
#66291=CARTESIAN_POINT('Ctrl Pts',(-19.0043702762566,44.8212,5.18882235256186));
#66292=CARTESIAN_POINT('',(-19.3754487165259,44.8212,5.36185907103561));
#66293=CARTESIAN_POINT('Origin',(-17.98,44.8212,7.87));
#66294=CARTESIAN_POINT('',(-19.3551,44.9412,5.48825693451204));
#66295=CARTESIAN_POINT('Ctrl Pts',(-19.3754487165259,44.8212,5.36185907103561));
#66296=CARTESIAN_POINT('Ctrl Pts',(-19.3650571276403,44.8826581248801,5.4264073501168));
#66297=CARTESIAN_POINT('Ctrl Pts',(-19.3551,44.9412,5.48825693451204));
#66298=CARTESIAN_POINT('',(-19.4543894024917,44.8212,5.40743549732803));
#66299=CARTESIAN_POINT('Ctrl Pts',(-19.3551,44.9412,5.48825693451204));
#66300=CARTESIAN_POINT('Ctrl Pts',(-19.4036847474797,44.88265812488,5.44870901682913));
#66301=CARTESIAN_POINT('Ctrl Pts',(-19.4543894024917,44.8212,5.40743549732802));
#66302=CARTESIAN_POINT('',(-19.7897828166121,44.8212,5.642280494161));
#66303=CARTESIAN_POINT('Origin',(-17.98,44.8212,7.87));
#66304=CARTESIAN_POINT('',(-19.7477944841599,44.9412,5.76322457253419));
#66305=CARTESIAN_POINT('Ctrl Pts',(-19.7897828166121,44.8212,5.642280494161));
#66306=CARTESIAN_POINT('Ctrl Pts',(-19.7683404082776,44.88265812488,5.70404365937065));
#66307=CARTESIAN_POINT('Ctrl Pts',(-19.7477944841599,44.9412,5.76322457253419));
#66308=CARTESIAN_POINT('',(-19.8596099528092,44.8212,5.70087241839011));
#66309=CARTESIAN_POINT('Ctrl Pts',(-19.7477944841599,44.9412,5.76322457253419));
#66310=CARTESIAN_POINT('Ctrl Pts',(-19.8025085439923,44.8826581248798,5.73271412944674));
#66311=CARTESIAN_POINT('Ctrl Pts',(-19.8596099528092,44.8212,5.70087241839011));
#66312=CARTESIAN_POINT('',(-20.1491275816099,44.8212,5.99039004719085));
#66313=CARTESIAN_POINT('Origin',(-17.98,44.8212,7.87));
#66314=CARTESIAN_POINT('',(-20.0867754274658,44.9412,6.10220551584008));
#66315=CARTESIAN_POINT('Ctrl Pts',(-20.1491275816099,44.8212,5.99039004719084));
#66316=CARTESIAN_POINT('Ctrl Pts',(-20.1172858705531,44.8826581248802,6.04749145600798));
#66317=CARTESIAN_POINT('Ctrl Pts',(-20.0867754274658,44.9412,6.10220551584008));
#66318=CARTESIAN_POINT('',(-20.207719505839,44.8212,6.0602171833879));
#66319=CARTESIAN_POINT('Ctrl Pts',(-20.0867754274658,44.9412,6.10220551584008));
#66320=CARTESIAN_POINT('Ctrl Pts',(-20.1459563406292,44.8826581248801,6.08165959172247));
#66321=CARTESIAN_POINT('Ctrl Pts',(-20.207719505839,44.8212,6.0602171833879));
#66322=CARTESIAN_POINT('',(-20.442564502672,44.8212,6.39561059750827));
#66323=CARTESIAN_POINT('Origin',(-17.98,44.8212,7.87));
#66324=CARTESIAN_POINT('',(-20.361743065488,44.9412,6.4949));
#66325=CARTESIAN_POINT('Ctrl Pts',(-20.442564502672,44.8212,6.39561059750826));
#66326=CARTESIAN_POINT('Ctrl Pts',(-20.401290983171,44.8826581248798,6.44631525252014));
#66327=CARTESIAN_POINT('Ctrl Pts',(-20.361743065488,44.9412,6.4949));
#66328=CARTESIAN_POINT('',(-20.4881409289644,44.8212,6.47455128347415));
#66329=CARTESIAN_POINT('Ctrl Pts',(-20.361743065488,44.9412,6.4949));
#66330=CARTESIAN_POINT('Ctrl Pts',(-20.4235926498833,44.8826581248799,6.48494287235964));
#66331=CARTESIAN_POINT('Ctrl Pts',(-20.4881409289644,44.8212,6.47455128347414));
#66332=CARTESIAN_POINT('',(-20.6611776474381,44.8212,6.84562972374336));
#66333=CARTESIAN_POINT('Origin',(-17.98,44.8212,7.87));
#66334=CARTESIAN_POINT('',(-20.5643426456854,44.9412,6.92937620182574));
#66335=CARTESIAN_POINT('Ctrl Pts',(-20.6611776474381,44.8212,6.84562972374336));
#66336=CARTESIAN_POINT('Ctrl Pts',(-20.6117263944974,44.8826581248799,6.88839698966571));
#66337=CARTESIAN_POINT('Ctrl Pts',(-20.5643426456854,44.9412,6.92937620182574));
#66338=CARTESIAN_POINT('',(-20.6923537591437,44.8212,6.93128538668091));
#66339=CARTESIAN_POINT('Ctrl Pts',(-20.5643426456854,44.9412,6.92937620182574));
#66340=CARTESIAN_POINT('Ctrl Pts',(-20.6269816329882,44.8826581248799,6.9303104129475));
#66341=CARTESIAN_POINT('Ctrl Pts',(-20.6923537591437,44.8212,6.93128538668091));
#66342=CARTESIAN_POINT('',(-20.7983245661282,44.8212,7.32677382246615));
#66343=CARTESIAN_POINT('Origin',(-17.98,44.8212,7.87));
#66344=CARTESIAN_POINT('',(-20.6884182823342,44.9412,7.39243278178041));
#66345=CARTESIAN_POINT('Ctrl Pts',(-20.7983245661282,44.8212,7.32677382246615));
#66346=CARTESIAN_POINT('Ctrl Pts',(-20.7421981310449,44.8826581248798,7.36030423756504));
#66347=CARTESIAN_POINT('Ctrl Pts',(-20.6884182823342,44.9412,7.39243278178041));
#66348=CARTESIAN_POINT('',(-20.8141530928687,44.8212,7.41654185840086));
#66349=CARTESIAN_POINT('Ctrl Pts',(-20.6884182823342,44.9412,7.39243278178041));
#66350=CARTESIAN_POINT('Ctrl Pts',(-20.7499434186121,44.8826581248797,7.40422994613214));
#66351=CARTESIAN_POINT('Ctrl Pts',(-20.8141530928687,44.8212,7.41654185840087));
#66352=CARTESIAN_POINT('',(-20.8498381190176,44.8212,7.82442357370758));
#66353=CARTESIAN_POINT('Origin',(-17.98,44.8212,7.87));
#66354=CARTESIAN_POINT('Ctrl Pts',(-20.8498381190176,44.8212,7.82442357370758));
#66355=CARTESIAN_POINT('Ctrl Pts',(-20.7887418751198,44.8826581248802,7.8476983332877));
#66356=CARTESIAN_POINT('Ctrl Pts',(-20.7302,44.9412,7.87));
#66357=CARTESIAN_POINT('',(-20.5502,45.1212,7.87));
#66358=CARTESIAN_POINT('',(-20.7002,44.9712,7.87));
#66359=CARTESIAN_POINT('Origin',(-17.98,45.1212,7.87));
#66360=CARTESIAN_POINT('Origin',(-14.9462632306524,45.1212,6.93607856095471));
#66361=CARTESIAN_POINT('',(-15.2676462408563,42.216,6.93128538668091));
#66362=CARTESIAN_POINT('',(-15.2676462408563,41.616,6.93128538668091));
#66363=CARTESIAN_POINT('',(-15.3956573543146,42.216,6.92937620182574));
#66364=CARTESIAN_POINT('',(-14.9462632306524,42.216,6.93607856095471));
#66365=CARTESIAN_POINT('',(-15.3956573543146,45.1212,6.92937620182574));
#66366=CARTESIAN_POINT('Origin',(-15.3956573543146,45.1212,6.92937620182574));
#66367=CARTESIAN_POINT('',(-15.2988223525619,42.216,6.84562972374336));
#66368=CARTESIAN_POINT('',(-15.2988223525619,41.616,6.84562972374336));
#66369=CARTESIAN_POINT('',(-15.3956573543146,42.216,6.92937620182574));
#66370=CARTESIAN_POINT('Origin',(-15.1983219039495,42.216,6.85755197172735));
#66371=CARTESIAN_POINT('Origin',(-17.98,42.216,7.87));
#66372=CARTESIAN_POINT('Origin',(-15.1545262649226,45.1212,6.42346406460551));
#66373=CARTESIAN_POINT('',(-15.4718590710356,42.216,6.47455128347414));
#66374=CARTESIAN_POINT('',(-15.4718590710356,41.616,6.47455128347414));
#66375=CARTESIAN_POINT('',(-15.598256934512,42.216,6.4949));
#66376=CARTESIAN_POINT('',(-15.1545262649226,42.216,6.42346406460551));
#66377=CARTESIAN_POINT('',(-15.598256934512,45.1212,6.4949));
#66378=CARTESIAN_POINT('Origin',(-15.598256934512,45.1212,6.4949));
#66379=CARTESIAN_POINT('',(-15.517435497328,42.216,6.39561059750826));
#66380=CARTESIAN_POINT('',(-15.517435497328,41.616,6.39561059750826));
#66381=CARTESIAN_POINT('',(-15.598256934512,42.216,6.4949));
#66382=CARTESIAN_POINT('Origin',(-15.4163915997173,42.216,6.3899));
#66383=CARTESIAN_POINT('Origin',(-17.98,42.216,7.87));
#66384=CARTESIAN_POINT('Origin',(-15.4486398888744,45.1212,5.95480183067077));
#66385=CARTESIAN_POINT('',(-15.752280494161,42.216,6.0602171833879));
#66386=CARTESIAN_POINT('',(-15.752280494161,41.616,6.0602171833879));
#66387=CARTESIAN_POINT('',(-15.8732245725342,42.216,6.10220551584008));
#66388=CARTESIAN_POINT('',(-15.4486398888744,42.216,5.95480183067077));
#66389=CARTESIAN_POINT('',(-15.8732245725342,45.1212,6.10220551584008));
#66390=CARTESIAN_POINT('Origin',(-15.8732245725342,45.1212,6.10220551584008));
#66391=CARTESIAN_POINT('',(-15.8108724183901,42.216,5.99039004719084));
#66392=CARTESIAN_POINT('',(-15.8108724183901,41.616,5.99039004719084));
#66393=CARTESIAN_POINT('',(-15.8732245725342,42.216,6.10220551584008));
#66394=CARTESIAN_POINT('Origin',(-15.7123552394792,42.216,5.96722011780591));
#66395=CARTESIAN_POINT('Origin',(-17.98,42.216,7.87));
#66396=CARTESIAN_POINT('Origin',(-15.8196676088727,45.1212,5.54433192397406));
#66397=CARTESIAN_POINT('',(-16.1003900471908,42.216,5.70087241839011));
#66398=CARTESIAN_POINT('',(-16.1003900471908,41.616,5.70087241839011));
#66399=CARTESIAN_POINT('',(-16.2122055158401,42.216,5.76322457253418));
#66400=CARTESIAN_POINT('',(-15.8196676088727,42.216,5.54433192397406));
#66401=CARTESIAN_POINT('',(-16.2122055158401,45.1212,5.76322457253418));
#66402=CARTESIAN_POINT('Origin',(-16.2122055158401,45.1212,5.76322457253418));
#66403=CARTESIAN_POINT('',(-16.1702171833879,42.216,5.642280494161));
#66404=CARTESIAN_POINT('',(-16.1702171833879,41.616,5.642280494161));
#66405=CARTESIAN_POINT('',(-16.2122055158401,42.216,5.76322457253418));
#66406=CARTESIAN_POINT('Origin',(-16.0772201178059,42.216,5.6023552394792));
#66407=CARTESIAN_POINT('Origin',(-17.98,42.216,7.87));
#66408=CARTESIAN_POINT('Origin',(-16.2563359353945,45.1212,5.20452626492257));
#66409=CARTESIAN_POINT('',(-16.5056105975083,42.216,5.40743549732803));
#66410=CARTESIAN_POINT('',(-16.5056105975083,41.616,5.40743549732803));
#66411=CARTESIAN_POINT('',(-16.6049,42.216,5.48825693451204));
#66412=CARTESIAN_POINT('',(-16.2563359353945,42.216,5.20452626492257));
#66413=CARTESIAN_POINT('',(-16.6049,45.1212,5.48825693451204));
#66414=CARTESIAN_POINT('Origin',(-16.6049,45.1212,5.48825693451204));
#66415=CARTESIAN_POINT('',(-16.5845512834741,42.216,5.36185907103561));
#66416=CARTESIAN_POINT('',(-16.5845512834741,41.616,5.36185907103561));
#66417=CARTESIAN_POINT('',(-16.6049,42.216,5.48825693451204));
#66418=CARTESIAN_POINT('Origin',(-16.4999,42.216,5.30639159971731));
#66419=CARTESIAN_POINT('Origin',(-17.98,42.216,7.87));
#66420=CARTESIAN_POINT('Origin',(-16.7453769223032,45.1212,4.94570967651662));
#66421=CARTESIAN_POINT('',(-16.9556297237434,42.216,5.18882235256186));
#66422=CARTESIAN_POINT('',(-16.9556297237434,41.616,5.18882235256186));
#66423=CARTESIAN_POINT('',(-17.0393762018257,42.216,5.28565735431459));
#66424=CARTESIAN_POINT('',(-16.7453769223032,42.216,4.94570967651662));
#66425=CARTESIAN_POINT('',(-17.0393762018257,45.1212,5.28565735431459));
#66426=CARTESIAN_POINT('Origin',(-17.0393762018257,45.1212,5.28565735431459));
#66427=CARTESIAN_POINT('',(-17.0412853866809,42.216,5.15764624085626));
#66428=CARTESIAN_POINT('',(-17.0412853866809,41.616,5.15764624085626));
#66429=CARTESIAN_POINT('',(-17.0393762018257,42.216,5.28565735431459));
#66430=CARTESIAN_POINT('Origin',(-16.9675519717274,42.216,5.08832190394955));
#66431=CARTESIAN_POINT('Origin',(-17.98,42.216,7.87));
#66432=CARTESIAN_POINT('Origin',(-17.2719313066783,45.1212,4.77574616982741));
#66433=CARTESIAN_POINT('',(-17.4367738224661,42.216,5.05167543387175));
#66434=CARTESIAN_POINT('',(-17.4367738224661,41.616,5.05167543387175));
#66435=CARTESIAN_POINT('',(-17.5024327817804,42.216,5.16158171766583));
#66436=CARTESIAN_POINT('',(-17.2719313066783,42.216,4.77574616982741));
#66437=CARTESIAN_POINT('',(-17.5024327817804,45.1212,5.16158171766583));
#66438=CARTESIAN_POINT('Origin',(-17.5024327817804,45.1212,5.16158171766583));
#66439=CARTESIAN_POINT('',(-17.5265418584009,42.216,5.03584690713126));
#66440=CARTESIAN_POINT('',(-17.5265418584009,41.616,5.03584690713126));
#66441=CARTESIAN_POINT('',(-17.5024327817804,42.216,5.16158171766583));
#66442=CARTESIAN_POINT('Origin',(-17.4659666644704,42.216,4.95477208953326));
#66443=CARTESIAN_POINT('Origin',(-17.98,42.216,7.87));
#66444=CARTESIAN_POINT('Origin',(-17.82,45.1212,4.6998));
#66445=CARTESIAN_POINT('',(-17.9344235737076,42.216,5.00016188098241));
#66446=CARTESIAN_POINT('',(-17.9344235737076,41.616,5.00016188098241));
#66447=CARTESIAN_POINT('',(-17.98,42.216,5.1198));
#66448=CARTESIAN_POINT('',(-17.82,42.216,4.6998));
#66449=CARTESIAN_POINT('',(-17.98,45.1212,5.1198));
#66450=CARTESIAN_POINT('Origin',(-17.98,45.1212,5.1198));
#66451=CARTESIAN_POINT('',(-18.0255764262924,42.216,5.00016188098241));
#66452=CARTESIAN_POINT('',(-18.0255764262924,41.616,5.00016188098241));
#66453=CARTESIAN_POINT('',(-17.98,42.216,5.1198));
#66454=CARTESIAN_POINT('Origin',(-17.98,42.216,4.9098));
#66455=CARTESIAN_POINT('Origin',(-17.98,42.216,7.87));
#66456=CARTESIAN_POINT('Origin',(-18.3729302123577,45.1212,4.72017875297399));
#66457=CARTESIAN_POINT('',(-18.4334581415991,42.216,5.03584690713126));
#66458=CARTESIAN_POINT('',(-18.4334581415991,41.616,5.03584690713126));
#66459=CARTESIAN_POINT('',(-18.4575672182196,42.216,5.16158171766583));
#66460=CARTESIAN_POINT('',(-18.3729302123577,42.216,4.72017875297399));
#66461=CARTESIAN_POINT('',(-18.4575672182196,45.1212,5.16158171766583));
#66462=CARTESIAN_POINT('Origin',(-18.4575672182196,45.1212,5.16158171766583));
#66463=CARTESIAN_POINT('',(-18.5232261775339,42.216,5.05167543387175));
#66464=CARTESIAN_POINT('',(-18.5232261775339,41.616,5.05167543387175));
#66465=CARTESIAN_POINT('',(-18.4575672182196,42.216,5.16158171766583));
#66466=CARTESIAN_POINT('Origin',(-18.4940333355296,42.216,4.95477208953326));
#66467=CARTESIAN_POINT('Origin',(-17.98,42.216,7.87));
#66468=CARTESIAN_POINT('Origin',(-18.9139214390453,45.1212,4.83626323065241));
#66469=CARTESIAN_POINT('',(-18.9187146133191,42.216,5.15764624085626));
#66470=CARTESIAN_POINT('',(-18.9187146133191,41.616,5.15764624085626));
#66471=CARTESIAN_POINT('',(-18.9206237981743,42.216,5.28565735431459));
#66472=CARTESIAN_POINT('',(-18.9139214390453,42.216,4.83626323065241));
#66473=CARTESIAN_POINT('',(-18.9206237981743,45.1212,5.28565735431459));
#66474=CARTESIAN_POINT('Origin',(-18.9206237981743,45.1212,5.28565735431459));
#66475=CARTESIAN_POINT('',(-19.0043702762566,42.216,5.18882235256187));
#66476=CARTESIAN_POINT('',(-19.0043702762566,41.616,5.18882235256187));
#66477=CARTESIAN_POINT('',(-18.9206237981743,42.216,5.28565735431459));
#66478=CARTESIAN_POINT('Origin',(-18.9924480282726,42.216,5.08832190394955));
#66479=CARTESIAN_POINT('Origin',(-17.98,42.216,7.87));
#66480=CARTESIAN_POINT('Origin',(-19.4265359353945,45.1212,5.04452626492258));
#66481=CARTESIAN_POINT('',(-19.3754487165259,42.216,5.36185907103561));
#66482=CARTESIAN_POINT('',(-19.3754487165259,41.616,5.36185907103561));
#66483=CARTESIAN_POINT('',(-19.3551,42.216,5.48825693451204));
#66484=CARTESIAN_POINT('',(-19.4265359353945,42.216,5.04452626492258));
#66485=CARTESIAN_POINT('',(-19.3551,45.1212,5.48825693451204));
#66486=CARTESIAN_POINT('Origin',(-19.3551,45.1212,5.48825693451204));
#66487=CARTESIAN_POINT('',(-19.4543894024917,42.216,5.40743549732803));
#66488=CARTESIAN_POINT('',(-19.4543894024917,41.616,5.40743549732803));
#66489=CARTESIAN_POINT('',(-19.3551,42.216,5.48825693451204));
#66490=CARTESIAN_POINT('Origin',(-19.4601,42.216,5.30639159971731));
#66491=CARTESIAN_POINT('Origin',(-17.98,42.216,7.87));
#66492=CARTESIAN_POINT('Origin',(-19.8951981693292,45.1212,5.33863988887437));
#66493=CARTESIAN_POINT('',(-19.7897828166121,42.216,5.642280494161));
#66494=CARTESIAN_POINT('',(-19.7897828166121,41.616,5.642280494161));
#66495=CARTESIAN_POINT('',(-19.7477944841599,42.216,5.76322457253419));
#66496=CARTESIAN_POINT('',(-19.8951981693292,42.216,5.33863988887437));
#66497=CARTESIAN_POINT('',(-19.7477944841599,45.1212,5.76322457253419));
#66498=CARTESIAN_POINT('Origin',(-19.7477944841599,45.1212,5.76322457253419));
#66499=CARTESIAN_POINT('',(-19.8596099528092,42.216,5.70087241839011));
#66500=CARTESIAN_POINT('',(-19.8596099528092,41.616,5.70087241839011));
#66501=CARTESIAN_POINT('',(-19.7477944841599,42.216,5.76322457253419));
#66502=CARTESIAN_POINT('Origin',(-19.8827798821941,42.216,5.6023552394792));
#66503=CARTESIAN_POINT('Origin',(-17.98,42.216,7.87));
#66504=CARTESIAN_POINT('Origin',(-20.3056680760259,45.1212,5.7096676088727));
#66505=CARTESIAN_POINT('',(-20.1491275816099,42.216,5.99039004719085));
#66506=CARTESIAN_POINT('',(-20.1491275816099,41.616,5.99039004719085));
#66507=CARTESIAN_POINT('',(-20.0867754274658,42.216,6.10220551584008));
#66508=CARTESIAN_POINT('',(-20.3056680760259,42.216,5.7096676088727));
#66509=CARTESIAN_POINT('',(-20.0867754274658,45.1212,6.10220551584008));
#66510=CARTESIAN_POINT('Origin',(-20.0867754274658,45.1212,6.10220551584008));
#66511=CARTESIAN_POINT('',(-20.207719505839,42.216,6.0602171833879));
#66512=CARTESIAN_POINT('',(-20.207719505839,41.616,6.0602171833879));
#66513=CARTESIAN_POINT('',(-20.0867754274658,42.216,6.10220551584008));
#66514=CARTESIAN_POINT('Origin',(-20.2476447605208,42.216,5.96722011780591));
#66515=CARTESIAN_POINT('Origin',(-17.98,42.216,7.87));
#66516=CARTESIAN_POINT('Origin',(-20.6454737350774,45.1212,6.14633593539449));
#66517=CARTESIAN_POINT('',(-20.442564502672,42.216,6.39561059750827));
#66518=CARTESIAN_POINT('',(-20.442564502672,41.616,6.39561059750827));
#66519=CARTESIAN_POINT('',(-20.361743065488,42.216,6.4949));
#66520=CARTESIAN_POINT('',(-20.6454737350774,42.216,6.14633593539449));
#66521=CARTESIAN_POINT('',(-20.361743065488,45.1212,6.4949));
#66522=CARTESIAN_POINT('Origin',(-20.361743065488,45.1212,6.4949));
#66523=CARTESIAN_POINT('',(-20.4881409289644,42.216,6.47455128347415));
#66524=CARTESIAN_POINT('',(-20.4881409289644,41.616,6.47455128347415));
#66525=CARTESIAN_POINT('',(-20.361743065488,42.216,6.4949));
#66526=CARTESIAN_POINT('Origin',(-20.5436084002827,42.216,6.3899));
#66527=CARTESIAN_POINT('Origin',(-17.98,42.216,7.87));
#66528=CARTESIAN_POINT('Origin',(-20.9042903234834,45.1212,6.63537692230322));
#66529=CARTESIAN_POINT('',(-20.6611776474381,42.216,6.84562972374336));
#66530=CARTESIAN_POINT('',(-20.6611776474381,41.616,6.84562972374336));
#66531=CARTESIAN_POINT('',(-20.5643426456854,42.216,6.92937620182575));
#66532=CARTESIAN_POINT('',(-20.9042903234834,42.216,6.63537692230322));
#66533=CARTESIAN_POINT('',(-20.5643426456854,45.1212,6.92937620182575));
#66534=CARTESIAN_POINT('Origin',(-20.5643426456854,45.1212,6.92937620182575));
#66535=CARTESIAN_POINT('',(-20.6923537591437,42.216,6.93128538668091));
#66536=CARTESIAN_POINT('',(-20.6923537591437,41.616,6.93128538668091));
#66537=CARTESIAN_POINT('',(-20.5643426456854,42.216,6.92937620182575));
#66538=CARTESIAN_POINT('Origin',(-20.7616780960504,42.216,6.85755197172736));
#66539=CARTESIAN_POINT('Origin',(-17.98,42.216,7.87));
#66540=CARTESIAN_POINT('Origin',(-21.0742538301726,45.1212,7.16193130667835));
#66541=CARTESIAN_POINT('',(-20.7983245661282,42.216,7.32677382246615));
#66542=CARTESIAN_POINT('',(-20.7983245661282,41.616,7.32677382246615));
#66543=CARTESIAN_POINT('',(-20.6884182823342,42.216,7.39243278178041));
#66544=CARTESIAN_POINT('',(-21.0742538301726,42.216,7.16193130667835));
#66545=CARTESIAN_POINT('',(-20.6884182823342,45.1212,7.39243278178041));
#66546=CARTESIAN_POINT('Origin',(-20.6884182823342,45.1212,7.39243278178041));
#66547=CARTESIAN_POINT('',(-20.8141530928687,42.216,7.41654185840086));
#66548=CARTESIAN_POINT('',(-20.8141530928687,41.616,7.41654185840086));
#66549=CARTESIAN_POINT('',(-20.6884182823342,42.216,7.39243278178041));
#66550=CARTESIAN_POINT('Origin',(-20.8952279104667,42.216,7.35596666447035));
#66551=CARTESIAN_POINT('Origin',(-17.98,42.216,7.87));
#66552=CARTESIAN_POINT('Origin',(-21.1502,45.1212,7.71));
#66553=CARTESIAN_POINT('',(-20.8498381190176,42.216,7.82442357370758));
#66554=CARTESIAN_POINT('',(-20.8498381190176,41.616,7.82442357370758));
#66555=CARTESIAN_POINT('',(-20.7302,42.216,7.87));
#66556=CARTESIAN_POINT('',(-21.1502,42.216,7.71));
#66557=CARTESIAN_POINT('',(-20.7302,45.1212,7.87));
#66558=CARTESIAN_POINT('Origin',(-20.7302,45.1212,7.87));
#66559=CARTESIAN_POINT('',(-20.8498381190176,42.216,7.91557642629242));
#66560=CARTESIAN_POINT('',(-20.8498381190176,41.616,7.91557642629242));
#66561=CARTESIAN_POINT('',(-20.7302,42.216,7.87));
#66562=CARTESIAN_POINT('Origin',(-20.9402,42.216,7.87));
#66563=CARTESIAN_POINT('',(-20.8502,42.216,7.87));
#66564=CARTESIAN_POINT('Origin',(-17.98,42.216,7.87));
#66565=CARTESIAN_POINT('Origin',(-17.98,42.216,7.87));
#66566=CARTESIAN_POINT('Origin',(-21.129821247026,45.1212,8.26293021235775));
#66567=CARTESIAN_POINT('',(-20.8141530928687,42.216,8.32345814159914));
#66568=CARTESIAN_POINT('',(-20.8141530928687,41.616,8.32345814159914));
#66569=CARTESIAN_POINT('',(-20.6884182823342,42.216,8.34756721821959));
#66570=CARTESIAN_POINT('',(-21.129821247026,42.216,8.26293021235775));
#66571=CARTESIAN_POINT('',(-20.6884182823342,45.1212,8.34756721821959));
#66572=CARTESIAN_POINT('Origin',(-20.6884182823342,45.1212,8.34756721821959));
#66573=CARTESIAN_POINT('',(-20.7983245661282,42.216,8.41322617753386));
#66574=CARTESIAN_POINT('',(-20.7983245661282,41.616,8.41322617753386));
#66575=CARTESIAN_POINT('',(-20.6884182823342,42.216,8.34756721821959));
#66576=CARTESIAN_POINT('Origin',(-20.8952279104667,42.216,8.38403333552965));
#66577=CARTESIAN_POINT('Origin',(-17.98,42.216,7.87));
#66578=CARTESIAN_POINT('Origin',(-21.0137367693476,45.1212,8.80392143904529));
#66579=CARTESIAN_POINT('',(-20.6923537591437,42.216,8.80871461331909));
#66580=CARTESIAN_POINT('',(-20.6923537591437,41.616,8.80871461331909));
#66581=CARTESIAN_POINT('',(-20.5643426456854,42.216,8.81062379817425));
#66582=CARTESIAN_POINT('',(-21.0137367693476,42.216,8.80392143904529));
#66583=CARTESIAN_POINT('',(-20.5643426456854,45.1212,8.81062379817425));
#66584=CARTESIAN_POINT('Origin',(-20.5643426456854,45.1212,8.81062379817425));
#66585=CARTESIAN_POINT('',(-20.6611776474381,42.216,8.89437027625664));
#66586=CARTESIAN_POINT('',(-20.6611776474381,41.616,8.89437027625664));
#66587=CARTESIAN_POINT('',(-20.5643426456854,42.216,8.81062379817425));
#66588=CARTESIAN_POINT('Origin',(-20.7616780960504,42.216,8.88244802827264));
#66589=CARTESIAN_POINT('Origin',(-17.98,42.216,7.87));
#66590=CARTESIAN_POINT('Origin',(-20.8054737350774,45.1212,9.31653593539449));
#66591=CARTESIAN_POINT('',(-20.4881409289644,42.216,9.26544871652585));
#66592=CARTESIAN_POINT('',(-20.4881409289644,41.616,9.26544871652585));
#66593=CARTESIAN_POINT('',(-20.361743065488,42.216,9.2451));
#66594=CARTESIAN_POINT('',(-20.8054737350774,42.216,9.31653593539449));
#66595=CARTESIAN_POINT('',(-20.361743065488,45.1212,9.2451));
#66596=CARTESIAN_POINT('Origin',(-20.361743065488,45.1212,9.2451));
#66597=CARTESIAN_POINT('',(-20.442564502672,42.216,9.34438940249174));
#66598=CARTESIAN_POINT('',(-20.442564502672,41.616,9.34438940249174));
#66599=CARTESIAN_POINT('',(-20.361743065488,42.216,9.2451));
#66600=CARTESIAN_POINT('Origin',(-20.5436084002827,42.216,9.3501));
#66601=CARTESIAN_POINT('Origin',(-17.98,42.216,7.87));
#66602=CARTESIAN_POINT('Origin',(-20.5113601111256,45.1212,9.78519816932923));
#66603=CARTESIAN_POINT('',(-20.207719505839,42.216,9.67978281661211));
#66604=CARTESIAN_POINT('',(-20.207719505839,41.616,9.67978281661211));
#66605=CARTESIAN_POINT('',(-20.0867754274658,42.216,9.63779448415992));
#66606=CARTESIAN_POINT('',(-20.5113601111256,42.216,9.78519816932923));
#66607=CARTESIAN_POINT('',(-20.0867754274658,45.1212,9.63779448415992));
#66608=CARTESIAN_POINT('Origin',(-20.0867754274658,45.1212,9.63779448415992));
#66609=CARTESIAN_POINT('',(-20.1491275816099,42.216,9.74960995280916));
#66610=CARTESIAN_POINT('',(-20.1491275816099,41.616,9.74960995280916));
#66611=CARTESIAN_POINT('',(-20.0867754274658,42.216,9.63779448415992));
#66612=CARTESIAN_POINT('Origin',(-20.2476447605208,42.216,9.77277988219409));
#66613=CARTESIAN_POINT('Origin',(-17.98,42.216,7.87));
#66614=CARTESIAN_POINT('Origin',(-20.1403323911273,45.1212,10.1956680760259));
#66615=CARTESIAN_POINT('',(-19.8596099528092,42.216,10.0391275816099));
#66616=CARTESIAN_POINT('',(-19.8596099528092,41.616,10.0391275816099));
#66617=CARTESIAN_POINT('',(-19.7477944841599,42.216,9.97677542746581));
#66618=CARTESIAN_POINT('',(-20.1403323911273,42.216,10.1956680760259));
#66619=CARTESIAN_POINT('',(-19.7477944841599,45.1212,9.97677542746581));
#66620=CARTESIAN_POINT('Origin',(-19.7477944841599,45.1212,9.97677542746581));
#66621=CARTESIAN_POINT('',(-19.7897828166121,42.216,10.097719505839));
#66622=CARTESIAN_POINT('',(-19.7897828166121,41.616,10.097719505839));
#66623=CARTESIAN_POINT('',(-19.7477944841599,42.216,9.97677542746581));
#66624=CARTESIAN_POINT('Origin',(-19.8827798821941,42.216,10.1376447605208));
#66625=CARTESIAN_POINT('Origin',(-17.98,42.216,7.87));
#66626=CARTESIAN_POINT('Origin',(-19.7036640646055,45.1212,10.5354737350774));
#66627=CARTESIAN_POINT('',(-19.4543894024917,42.216,10.332564502672));
#66628=CARTESIAN_POINT('',(-19.4543894024917,41.616,10.332564502672));
#66629=CARTESIAN_POINT('',(-19.3551,42.216,10.251743065488));
#66630=CARTESIAN_POINT('',(-19.7036640646055,42.216,10.5354737350774));
#66631=CARTESIAN_POINT('',(-19.3551,45.1212,10.251743065488));
#66632=CARTESIAN_POINT('Origin',(-19.3551,45.1212,10.251743065488));
#66633=CARTESIAN_POINT('',(-19.3754487165258,42.216,10.3781409289644));
#66634=CARTESIAN_POINT('',(-19.3754487165258,41.616,10.3781409289644));
#66635=CARTESIAN_POINT('',(-19.3551,42.216,10.251743065488));
#66636=CARTESIAN_POINT('Origin',(-19.4601,42.216,10.4336084002827));
#66637=CARTESIAN_POINT('Origin',(-17.98,42.216,7.87));
#66638=CARTESIAN_POINT('Origin',(-19.2146230776968,45.1212,10.7942903234834));
#66639=CARTESIAN_POINT('',(-19.0043702762566,42.216,10.5511776474381));
#66640=CARTESIAN_POINT('',(-19.0043702762566,41.616,10.5511776474381));
#66641=CARTESIAN_POINT('',(-18.9206237981742,42.216,10.4543426456854));
#66642=CARTESIAN_POINT('',(-19.2146230776968,42.216,10.7942903234834));
#66643=CARTESIAN_POINT('',(-18.9206237981742,45.1212,10.4543426456854));
#66644=CARTESIAN_POINT('Origin',(-18.9206237981742,45.1212,10.4543426456854));
#66645=CARTESIAN_POINT('',(-18.9187146133191,42.216,10.5823537591437));
#66646=CARTESIAN_POINT('',(-18.9187146133191,41.616,10.5823537591437));
#66647=CARTESIAN_POINT('',(-18.9206237981742,42.216,10.4543426456854));
#66648=CARTESIAN_POINT('Origin',(-18.9924480282726,42.216,10.6516780960504));
#66649=CARTESIAN_POINT('Origin',(-17.98,42.216,7.87));
#66650=CARTESIAN_POINT('Origin',(-18.6880686933217,45.1212,10.9642538301726));
#66651=CARTESIAN_POINT('',(-18.5232261775339,42.216,10.6883245661282));
#66652=CARTESIAN_POINT('',(-18.5232261775339,41.616,10.6883245661282));
#66653=CARTESIAN_POINT('',(-18.4575672182196,42.216,10.5784182823342));
#66654=CARTESIAN_POINT('',(-18.6880686933217,42.216,10.9642538301726));
#66655=CARTESIAN_POINT('',(-18.4575672182196,45.1212,10.5784182823342));
#66656=CARTESIAN_POINT('Origin',(-18.4575672182196,45.1212,10.5784182823342));
#66657=CARTESIAN_POINT('',(-18.4334581415991,42.216,10.7041530928687));
#66658=CARTESIAN_POINT('',(-18.4334581415991,41.616,10.7041530928687));
#66659=CARTESIAN_POINT('',(-18.4575672182196,42.216,10.5784182823342));
#66660=CARTESIAN_POINT('Origin',(-18.4940333355296,42.216,10.7852279104667));
#66661=CARTESIAN_POINT('Origin',(-17.98,42.216,7.87));
#66662=CARTESIAN_POINT('Origin',(-18.14,45.1212,11.0402));
#66663=CARTESIAN_POINT('',(-18.0255764262924,42.216,10.7398381190176));
#66664=CARTESIAN_POINT('',(-18.0255764262924,41.616,10.7398381190176));
#66665=CARTESIAN_POINT('',(-17.98,42.216,10.6202));
#66666=CARTESIAN_POINT('',(-18.14,42.216,11.0402));
#66667=CARTESIAN_POINT('',(-17.98,45.1212,10.6202));
#66668=CARTESIAN_POINT('Origin',(-17.98,45.1212,10.6202));
#66669=CARTESIAN_POINT('',(-17.9344235737076,42.216,10.7398381190176));
#66670=CARTESIAN_POINT('',(-17.9344235737076,41.616,10.7398381190176));
#66671=CARTESIAN_POINT('',(-17.98,42.216,10.6202));
#66672=CARTESIAN_POINT('Origin',(-17.98,42.216,10.8302));
#66673=CARTESIAN_POINT('Origin',(-17.98,42.216,7.87));
#66674=CARTESIAN_POINT('Origin',(-17.5870697876422,45.1212,11.019821247026));
#66675=CARTESIAN_POINT('',(-17.5265418584009,42.216,10.7041530928687));
#66676=CARTESIAN_POINT('',(-17.5265418584009,41.616,10.7041530928687));
#66677=CARTESIAN_POINT('',(-17.5024327817804,42.216,10.5784182823342));
#66678=CARTESIAN_POINT('',(-17.5870697876422,42.216,11.019821247026));
#66679=CARTESIAN_POINT('',(-17.5024327817804,45.1212,10.5784182823342));
#66680=CARTESIAN_POINT('Origin',(-17.5024327817804,45.1212,10.5784182823342));
#66681=CARTESIAN_POINT('',(-17.4367738224661,42.216,10.6883245661282));
#66682=CARTESIAN_POINT('',(-17.4367738224661,41.616,10.6883245661282));
#66683=CARTESIAN_POINT('',(-17.5024327817804,42.216,10.5784182823342));
#66684=CARTESIAN_POINT('Origin',(-17.4659666644703,42.216,10.7852279104667));
#66685=CARTESIAN_POINT('Origin',(-17.98,42.216,7.87));
#66686=CARTESIAN_POINT('Origin',(-17.0460785609547,45.1212,10.9037367693476));
#66687=CARTESIAN_POINT('',(-17.0412853866809,42.216,10.5823537591437));
#66688=CARTESIAN_POINT('',(-17.0412853866809,41.616,10.5823537591437));
#66689=CARTESIAN_POINT('',(-17.0393762018257,42.216,10.4543426456854));
#66690=CARTESIAN_POINT('',(-17.0460785609547,42.216,10.9037367693476));
#66691=CARTESIAN_POINT('',(-17.0393762018257,45.1212,10.4543426456854));
#66692=CARTESIAN_POINT('Origin',(-17.0393762018257,45.1212,10.4543426456854));
#66693=CARTESIAN_POINT('',(-16.9556297237434,42.216,10.5511776474381));
#66694=CARTESIAN_POINT('',(-16.9556297237434,41.616,10.5511776474381));
#66695=CARTESIAN_POINT('',(-17.0393762018257,42.216,10.4543426456854));
#66696=CARTESIAN_POINT('Origin',(-16.9675519717273,42.216,10.6516780960504));
#66697=CARTESIAN_POINT('Origin',(-17.98,42.216,7.87));
#66698=CARTESIAN_POINT('Origin',(-16.5334640646055,45.1212,10.6954737350774));
#66699=CARTESIAN_POINT('',(-16.5845512834741,42.216,10.3781409289644));
#66700=CARTESIAN_POINT('',(-16.5845512834741,41.616,10.3781409289644));
#66701=CARTESIAN_POINT('',(-16.6049,42.216,10.251743065488));
#66702=CARTESIAN_POINT('',(-16.5334640646055,42.216,10.6954737350774));
#66703=CARTESIAN_POINT('',(-16.6049,45.1212,10.251743065488));
#66704=CARTESIAN_POINT('Origin',(-16.6049,45.1212,10.251743065488));
#66705=CARTESIAN_POINT('',(-16.5056105975083,42.216,10.332564502672));
#66706=CARTESIAN_POINT('',(-16.5056105975083,41.616,10.332564502672));
#66707=CARTESIAN_POINT('',(-16.6049,42.216,10.251743065488));
#66708=CARTESIAN_POINT('Origin',(-16.4999,42.216,10.4336084002827));
#66709=CARTESIAN_POINT('Origin',(-17.98,42.216,7.87));
#66710=CARTESIAN_POINT('Origin',(-16.0648018306708,45.1212,10.4013601111256));
#66711=CARTESIAN_POINT('',(-16.1702171833879,42.216,10.097719505839));
#66712=CARTESIAN_POINT('',(-16.1702171833879,41.616,10.097719505839));
#66713=CARTESIAN_POINT('',(-16.2122055158401,42.216,9.97677542746581));
#66714=CARTESIAN_POINT('',(-16.0648018306708,42.216,10.4013601111256));
#66715=CARTESIAN_POINT('',(-16.2122055158401,45.1212,9.97677542746581));
#66716=CARTESIAN_POINT('Origin',(-16.2122055158401,45.1212,9.97677542746581));
#66717=CARTESIAN_POINT('',(-16.1003900471908,42.216,10.0391275816099));
#66718=CARTESIAN_POINT('',(-16.1003900471908,41.616,10.0391275816099));
#66719=CARTESIAN_POINT('',(-16.2122055158401,42.216,9.97677542746581));
#66720=CARTESIAN_POINT('Origin',(-16.0772201178059,42.216,10.1376447605208));
#66721=CARTESIAN_POINT('Origin',(-17.98,42.216,7.87));
#66722=CARTESIAN_POINT('Origin',(-15.6543319239741,45.1212,10.0303323911273));
#66723=CARTESIAN_POINT('',(-15.8108724183901,42.216,9.74960995280916));
#66724=CARTESIAN_POINT('',(-15.8108724183901,41.616,9.74960995280916));
#66725=CARTESIAN_POINT('',(-15.8732245725342,42.216,9.63779448415992));
#66726=CARTESIAN_POINT('',(-15.6543319239741,42.216,10.0303323911273));
#66727=CARTESIAN_POINT('',(-15.8732245725342,45.1212,9.63779448415992));
#66728=CARTESIAN_POINT('Origin',(-15.8732245725342,45.1212,9.63779448415992));
#66729=CARTESIAN_POINT('',(-15.752280494161,42.216,9.67978281661211));
#66730=CARTESIAN_POINT('',(-15.752280494161,41.616,9.67978281661211));
#66731=CARTESIAN_POINT('',(-15.8732245725342,42.216,9.63779448415992));
#66732=CARTESIAN_POINT('Origin',(-15.7123552394792,42.216,9.77277988219409));
#66733=CARTESIAN_POINT('Origin',(-17.98,42.216,7.87));
#66734=CARTESIAN_POINT('Origin',(-15.3145262649226,45.1212,9.59366406460551));
#66735=CARTESIAN_POINT('',(-15.517435497328,42.216,9.34438940249174));
#66736=CARTESIAN_POINT('',(-15.517435497328,41.616,9.34438940249174));
#66737=CARTESIAN_POINT('',(-15.598256934512,42.216,9.2451));
#66738=CARTESIAN_POINT('',(-15.3145262649226,42.216,9.59366406460551));
#66739=CARTESIAN_POINT('',(-15.598256934512,45.1212,9.2451));
#66740=CARTESIAN_POINT('Origin',(-15.598256934512,45.1212,9.2451));
#66741=CARTESIAN_POINT('',(-15.4718590710356,42.216,9.26544871652585));
#66742=CARTESIAN_POINT('',(-15.4718590710356,41.616,9.26544871652585));
#66743=CARTESIAN_POINT('',(-15.598256934512,42.216,9.2451));
#66744=CARTESIAN_POINT('Origin',(-15.4163915997173,42.216,9.3501));
#66745=CARTESIAN_POINT('Origin',(-17.98,42.216,7.87));
#66746=CARTESIAN_POINT('Origin',(-15.0557096765166,45.1212,9.10462307769678));
#66747=CARTESIAN_POINT('',(-15.2988223525619,42.216,8.89437027625664));
#66748=CARTESIAN_POINT('',(-15.2988223525619,41.616,8.89437027625664));
#66749=CARTESIAN_POINT('',(-15.3956573543146,42.216,8.81062379817425));
#66750=CARTESIAN_POINT('',(-15.0557096765166,42.216,9.10462307769678));
#66751=CARTESIAN_POINT('',(-15.3956573543146,45.1212,8.81062379817425));
#66752=CARTESIAN_POINT('Origin',(-15.3956573543146,45.1212,8.81062379817425));
#66753=CARTESIAN_POINT('',(-15.2676462408563,42.216,8.80871461331909));
#66754=CARTESIAN_POINT('',(-15.2676462408563,41.616,8.80871461331909));
#66755=CARTESIAN_POINT('',(-15.3956573543146,42.216,8.81062379817425));
#66756=CARTESIAN_POINT('Origin',(-15.1983219039496,42.216,8.88244802827264));
#66757=CARTESIAN_POINT('Origin',(-17.98,42.216,7.87));
#66758=CARTESIAN_POINT('Origin',(-14.8857461698274,45.1212,8.57806869332165));
#66759=CARTESIAN_POINT('',(-15.1616754338717,42.216,8.41322617753385));
#66760=CARTESIAN_POINT('',(-15.1616754338717,41.616,8.41322617753385));
#66761=CARTESIAN_POINT('',(-15.2715817176658,42.216,8.34756721821959));
#66762=CARTESIAN_POINT('',(-14.8857461698274,42.216,8.57806869332165));
#66763=CARTESIAN_POINT('',(-15.2715817176658,45.1212,8.34756721821959));
#66764=CARTESIAN_POINT('Origin',(-15.2715817176658,45.1212,8.34756721821959));
#66765=CARTESIAN_POINT('',(-15.1458469071313,42.216,8.32345814159914));
#66766=CARTESIAN_POINT('',(-15.1458469071313,41.616,8.32345814159913));
#66767=CARTESIAN_POINT('',(-15.2715817176658,42.216,8.34756721821959));
#66768=CARTESIAN_POINT('Origin',(-15.0647720895333,42.216,8.38403333552965));
#66769=CARTESIAN_POINT('Origin',(-17.98,42.216,7.87));
#66770=CARTESIAN_POINT('Origin',(-14.8098,45.1212,8.03));
#66771=CARTESIAN_POINT('',(-15.1101618809824,42.216,7.91557642629241));
#66772=CARTESIAN_POINT('',(-15.1101618809824,41.616,7.91557642629241));
#66773=CARTESIAN_POINT('',(-15.2298,42.216,7.87));
#66774=CARTESIAN_POINT('',(-14.8098,42.216,8.03));
#66775=CARTESIAN_POINT('',(-15.2298,45.1212,7.87));
#66776=CARTESIAN_POINT('Origin',(-15.2298,45.1212,7.87));
#66777=CARTESIAN_POINT('',(-15.1101618809824,42.216,7.82442357370758));
#66778=CARTESIAN_POINT('',(-15.1101618809824,41.616,7.82442357370758));
#66779=CARTESIAN_POINT('',(-15.2298,42.216,7.87));
#66780=CARTESIAN_POINT('Origin',(-15.0198,42.216,7.87));
#66781=CARTESIAN_POINT('Origin',(-17.98,42.216,7.87));
#66782=CARTESIAN_POINT('Origin',(-17.98,41.616,7.87));
#66783=CARTESIAN_POINT('',(-20.8502,41.616,7.87));
#66784=CARTESIAN_POINT('Origin',(-17.98,45.1212,7.87));
#66785=CARTESIAN_POINT('',(-19.5839512165924,45.1212,7.87));
#66786=CARTESIAN_POINT('',(-18.7819756082962,45.1212,6.4809375));
#66787=CARTESIAN_POINT('',(-19.3834573145184,45.1212,7.522734375));
#66788=CARTESIAN_POINT('',(-17.1780243917038,45.1212,6.4809375));
#66789=CARTESIAN_POINT('',(-18.3809878041481,45.1212,6.4809375));
#66790=CARTESIAN_POINT('',(-16.3760487834076,45.1212,7.87));
#66791=CARTESIAN_POINT('',(-16.9775304896297,45.1212,6.828203125));
#66792=CARTESIAN_POINT('',(-17.1780243917038,45.1212,9.2590625));
#66793=CARTESIAN_POINT('',(-16.5765426854816,45.1212,8.217265625));
#66794=CARTESIAN_POINT('',(-18.7819756082962,45.1212,9.2590625));
#66795=CARTESIAN_POINT('',(-17.5790121958519,45.1212,9.2590625));
#66796=CARTESIAN_POINT('',(-18.9824695103703,45.1212,8.911796875));
#66797=CARTESIAN_POINT('Origin',(-16.3760487834076,43.3212,7.87));
#66798=CARTESIAN_POINT('',(-19.5839512165924,43.3212,7.87));
#66799=CARTESIAN_POINT('',(-18.7819756082962,43.3212,6.4809375));
#66800=CARTESIAN_POINT('',(-19.5839512165924,43.3212,7.87));
#66801=CARTESIAN_POINT('Origin',(-17.98,43.3212,7.87));
#66802=CARTESIAN_POINT('Origin',(-16.3760487834076,43.3212,7.87));
#66803=CARTESIAN_POINT('',(-17.1780243917038,43.3212,6.4809375));
#66804=CARTESIAN_POINT('',(-18.7819756082962,43.3212,6.4809375));
#66805=CARTESIAN_POINT('Origin',(-17.98,43.3212,7.87));
#66806=CARTESIAN_POINT('Origin',(-16.3760487834076,43.3212,7.87));
#66807=CARTESIAN_POINT('',(-16.3760487834076,43.3212,7.87));
#66808=CARTESIAN_POINT('',(-17.1780243917038,43.3212,6.4809375));
#66809=CARTESIAN_POINT('Origin',(-17.98,43.3212,7.87));
#66810=CARTESIAN_POINT('Origin',(-16.3760487834076,43.3212,7.87));
#66811=CARTESIAN_POINT('',(-17.1780243917038,43.3212,9.2590625));
#66812=CARTESIAN_POINT('',(-16.3760487834076,43.3212,7.87));
#66813=CARTESIAN_POINT('Origin',(-17.98,43.3212,7.87));
#66814=CARTESIAN_POINT('Origin',(-16.3760487834076,43.3212,7.87));
#66815=CARTESIAN_POINT('',(-18.7819756082962,43.3212,9.2590625));
#66816=CARTESIAN_POINT('',(-17.1780243917038,43.3212,9.2590625));
#66817=CARTESIAN_POINT('Origin',(-17.98,43.3212,7.87));
#66818=CARTESIAN_POINT('Origin',(-16.3760487834076,43.3212,7.87));
#66819=CARTESIAN_POINT('',(-18.7819756082962,43.3212,9.2590625));
#66820=CARTESIAN_POINT('Origin',(-17.98,43.3212,7.87));
#66821=CARTESIAN_POINT('Origin',(-17.98,43.3212,7.87));
#66822=CARTESIAN_POINT('',(-17.98,42.3574488791083,7.87));
#66823=CARTESIAN_POINT('',(-19.5839512165924,43.3212,7.87));
#66824=CARTESIAN_POINT('Origin',(-19.5839512165924,45.1212,7.87));
#66825=CARTESIAN_POINT('',(-19.5839512165924,45.1212,7.87));
#66826=CARTESIAN_POINT('',(-18.7819756082962,45.1212,6.4809375));
#66827=CARTESIAN_POINT('Origin',(-18.7819756082962,45.1212,9.2590625));
#66828=CARTESIAN_POINT('',(-18.7819756082962,45.1212,9.2590625));
#66829=CARTESIAN_POINT('Origin',(-17.1780243917038,45.1212,9.2590625));
#66830=CARTESIAN_POINT('',(-17.1780243917038,45.1212,9.2590625));
#66831=CARTESIAN_POINT('Origin',(-16.3760487834076,45.1212,7.87));
#66832=CARTESIAN_POINT('',(-16.3760487834076,45.1212,7.87));
#66833=CARTESIAN_POINT('Origin',(-17.1780243917038,45.1212,6.4809375));
#66834=CARTESIAN_POINT('',(-17.1780243917038,45.1212,6.4809375));
#66835=CARTESIAN_POINT('Origin',(-18.7819756082962,45.1212,6.4809375));
#83199=UNCERTAINTY_MEASURE_WITH_UNIT(LENGTH_MEASURE(0.01),#83220,
'DISTANCE_ACCURACY_VALUE',
'Maximum model space distance between geometric entities at asserted c
onnectivities');
#83203=UNCERTAINTY_MEASURE_WITH_UNIT(LENGTH_MEASURE(0.01),#83220,
'DISTANCE_ACCURACY_VALUE',
'Maximum model space distance between geometric entities at asserted c
onnectivities');
#83215=(
GEOMETRIC_REPRESENTATION_CONTEXT(3)
GLOBAL_UNCERTAINTY_ASSIGNED_CONTEXT((#83199))
GLOBAL_UNIT_ASSIGNED_CONTEXT((#83220,#83222,#83223))
REPRESENTATION_CONTEXT('','3D')
);
#83219=(
GEOMETRIC_REPRESENTATION_CONTEXT(3)
GLOBAL_UNCERTAINTY_ASSIGNED_CONTEXT((#83203))
GLOBAL_UNIT_ASSIGNED_CONTEXT((#83220,#83222,#83223))
REPRESENTATION_CONTEXT('','3D')
);
#83220=(
LENGTH_UNIT()
NAMED_UNIT(*)
SI_UNIT(.MILLI.,.METRE.)
);
#83222=(
NAMED_UNIT(*)
PLANE_ANGLE_UNIT()
SI_UNIT($,.RADIAN.)
);
#83223=(
NAMED_UNIT(*)
SI_UNIT($,.STERADIAN.)
SOLID_ANGLE_UNIT()
);
#83235=SHAPE_DEFINITION_REPRESENTATION(#83250,#83310);
#83250=PRODUCT_DEFINITION_SHAPE('',$,#83326);
#83310=SHAPE_REPRESENTATION('',(#28693),#83215);
#83314=PRODUCT_DEFINITION_CONTEXT('part definition',#83361,'design');
#83326=PRODUCT_DEFINITION('ASME B18.3 SHCS 6-32 UNC x 0.3125',
'ASME B18.3 SHCS 6-32 UNC x 0.3125',#83341,#83314);
#83341=PRODUCT_DEFINITION_FORMATION('',$,#83374);
#83361=APPLICATION_CONTEXT(
'Core Data for Automotive Mechanical Design Process');
#83362=PRODUCT_CONTEXT('part definition',#83361,'mechanical');
#83374=PRODUCT('ASME B18.3 SHCS 6-32 UNC x 0.3125',
'ASME B18.3 SHCS 6-32 UNC x 0.3125',$,(#83362));
#83389=PRESENTATION_STYLE_ASSIGNMENT((#83404));
#83404=SURFACE_STYLE_USAGE(.BOTH.,#83419);
#83419=SURFACE_SIDE_STYLE('',(#83434));
#83434=SURFACE_STYLE_FILL_AREA(#83449);
#83449=FILL_AREA_STYLE('Opaque(201,205,211)',(#83464));
#83464=FILL_AREA_STYLE_COLOUR('Opaque(201,205,211)',#83479);
#83479=COLOUR_RGB('Opaque(201,205,211)', 0.08235294, 0.09019608, 0.10196078);
ENDSEC;
END-ISO-10303-21;
